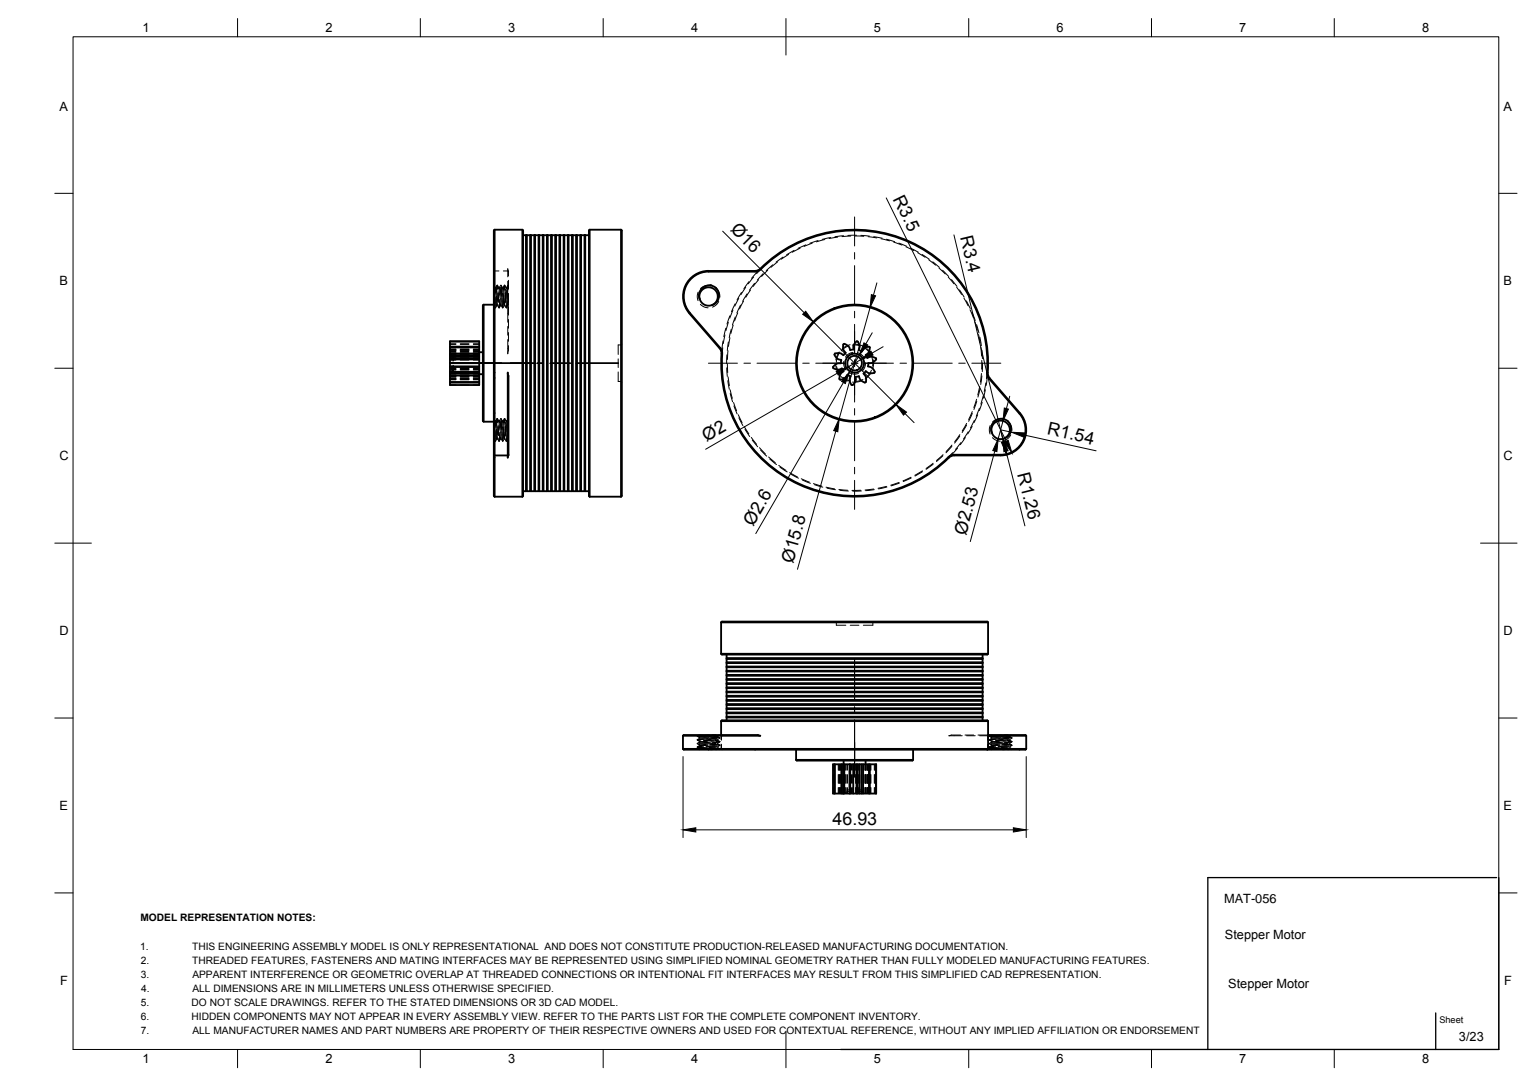
ISO-10303-21;
HEADER;
/* Generated by software containing ST-Developer
 * from STEP Tools, Inc. (www.steptools.com) 
 */

FILE_DESCRIPTION(
/* description */ (''),
/* implementation_level */ '2;1');

FILE_NAME(
/* name */ 'Stepper Motor.step',
/* time_stamp */ '2026-10-28T16:47:13+01:00',
/* author */ (''),
/* organization */ (''),
/* preprocessor_version */ 'ST-DEVELOPER v20.2',
/* originating_system */ 'Autodesk Translation Framework v15.17.0.0',
/* authorisation */ '');

FILE_SCHEMA (('AUTOMOTIVE_DESIGN { 1 0 10303 214 3 1 1 }'));
ENDSEC;

DATA;
#10=MECHANICAL_DESIGN_GEOMETRIC_PRESENTATION_REPRESENTATION('',(#4494,#4495,#4496,#4497,#4498,#4499,#4500,#4501,#4502,#4503,#4504,#4505,#4506,#4507,#4508,#4509,#4510,#4511,#4512,#4513,#4514,#4515,#4516,#4517,#4518,#4519,#4520,#4521,#4522,#4523,#4524,#4525,#4526,#4527,#4528,#4529,#4530,#4531,#4532,#4533,#4534,#4535,#4536,#4537,#4538,#4539,#4540,#4541,#4542,#4543,#4544,#4545,#4546,#4547,#4548,#4549,#4550,#4551,#4552,#4553,#4554,#4555,#4556,#4557,#4558,#4559,#4560,#4561,#4562,#4563,#4564,#4565,#4566),#459242);
#4405=SHAPE_REPRESENTATION_RELATIONSHIP('SRR','None',#459330,#4426);
#4426=ADVANCED_BREP_SHAPE_REPRESENTATION('',(#4447),#459219);
#4447=MANIFOLD_SOLID_BREP('NEMA14 body',#94623);
#4494=STYLED_ITEM('',(#459540),#88842);
#4495=STYLED_ITEM('',(#459540),#88843);
#4496=STYLED_ITEM('',(#459540),#88846);
#4497=STYLED_ITEM('',(#459540),#88849);
#4498=STYLED_ITEM('',(#459540),#88881);
#4499=STYLED_ITEM('',(#459540),#88885);
#4500=STYLED_ITEM('',(#459540),#88886);
#4501=STYLED_ITEM('',(#459540),#88887);
#4502=STYLED_ITEM('',(#459540),#88888);
#4503=STYLED_ITEM('',(#459540),#88889);
#4504=STYLED_ITEM('',(#459540),#88890);
#4505=STYLED_ITEM('',(#459540),#88891);
#4506=STYLED_ITEM('',(#459540),#88892);
#4507=STYLED_ITEM('',(#459540),#88893);
#4508=STYLED_ITEM('',(#459540),#88894);
#4509=STYLED_ITEM('',(#459540),#88895);
#4510=STYLED_ITEM('',(#459540),#88896);
#4511=STYLED_ITEM('',(#459540),#88897);
#4512=STYLED_ITEM('',(#459540),#88898);
#4513=STYLED_ITEM('',(#459540),#88899);
#4514=STYLED_ITEM('',(#459540),#88900);
#4515=STYLED_ITEM('',(#459540),#88901);
#4516=STYLED_ITEM('',(#459540),#88902);
#4517=STYLED_ITEM('',(#459540),#88903);
#4518=STYLED_ITEM('',(#459540),#88904);
#4519=STYLED_ITEM('',(#459540),#88905);
#4520=STYLED_ITEM('',(#459540),#88906);
#4521=STYLED_ITEM('',(#459540),#88907);
#4522=STYLED_ITEM('',(#459540),#88908);
#4523=STYLED_ITEM('',(#459540),#88909);
#4524=STYLED_ITEM('',(#459540),#88910);
#4525=STYLED_ITEM('',(#459540),#88911);
#4526=STYLED_ITEM('',(#459540),#88912);
#4527=STYLED_ITEM('',(#459540),#88913);
#4528=STYLED_ITEM('',(#459540),#88914);
#4529=STYLED_ITEM('',(#459540),#88915);
#4530=STYLED_ITEM('',(#459540),#88916);
#4531=STYLED_ITEM('',(#459540),#88917);
#4532=STYLED_ITEM('',(#459540),#88918);
#4533=STYLED_ITEM('',(#459540),#88919);
#4534=STYLED_ITEM('',(#459540),#88920);
#4535=STYLED_ITEM('',(#459540),#88921);
#4536=STYLED_ITEM('',(#459540),#88922);
#4537=STYLED_ITEM('',(#459540),#88923);
#4538=STYLED_ITEM('',(#459540),#88924);
#4539=STYLED_ITEM('',(#459540),#88925);
#4540=STYLED_ITEM('',(#459540),#88926);
#4541=STYLED_ITEM('',(#459540),#88927);
#4542=STYLED_ITEM('',(#459540),#88928);
#4543=STYLED_ITEM('',(#459540),#88929);
#4544=STYLED_ITEM('',(#459540),#88930);
#4545=STYLED_ITEM('',(#459540),#88931);
#4546=STYLED_ITEM('',(#459540),#88932);
#4547=STYLED_ITEM('',(#459540),#88933);
#4548=STYLED_ITEM('',(#459540),#88934);
#4549=STYLED_ITEM('',(#459540),#88935);
#4550=STYLED_ITEM('',(#459540),#88936);
#4551=STYLED_ITEM('',(#459540),#88937);
#4552=STYLED_ITEM('',(#459540),#88938);
#4553=STYLED_ITEM('',(#459540),#88939);
#4554=STYLED_ITEM('',(#459540),#88940);
#4555=STYLED_ITEM('',(#459540),#88941);
#4556=STYLED_ITEM('',(#459540),#88942);
#4557=STYLED_ITEM('',(#459540),#88943);
#4558=STYLED_ITEM('',(#459540),#88944);
#4559=STYLED_ITEM('',(#459540),#88945);
#4560=STYLED_ITEM('',(#459540),#88946);
#4561=STYLED_ITEM('',(#459540),#88947);
#4562=STYLED_ITEM('',(#459540),#88948);
#4563=STYLED_ITEM('',(#459540),#88949);
#4564=STYLED_ITEM('',(#459540),#88997);
#4565=STYLED_ITEM('',(#459540),#88999);
#4566=STYLED_ITEM('',(#459540),#4447);
#4614=CONICAL_SURFACE('',#94946,7.95,0.785398163397448);
#4615=CONICAL_SURFACE('',#94953,18.2,0.785398163397448);
#4616=CONICAL_SURFACE('',#94962,18.2,0.785398163397437);
#4617=CONICAL_SURFACE('',#94970,2.55,0.785398163397459);
#4618=CONICAL_SURFACE('',#94977,18.2,0.785398163397459);
#4619=CONICAL_SURFACE('',#94978,1.05,0.785398163397442);
#4620=CONICAL_SURFACE('',#94981,3.45000000056584,0.785398163397459);
#4621=CONICAL_SURFACE('',#94984,1.05,0.785398163397449);
#4622=CONICAL_SURFACE('',#94986,1.05,0.785398163397451);
#4623=CONICAL_SURFACE('',#94989,3.44999999943895,0.785398163397441);
#4624=CONICAL_SURFACE('',#94992,1.05,0.785398163397451);
#4625=CONICAL_SURFACE('',#94995,3.44999999943895,0.785398163397441);
#4626=CONICAL_SURFACE('',#94999,1.05,0.785398163397451);
#4627=CONICAL_SURFACE('',#95002,18.2,0.785398163397448);
#4628=CONICAL_SURFACE('',#95004,1.05,0.785398163397449);
#4629=CONICAL_SURFACE('',#95008,3.45000000056584,0.785398163397459);
#4630=CONICAL_SURFACE('',#95012,1.05,0.785398163397442);
#4631=CONICAL_SURFACE('',#95015,18.2,0.785398163397437);
#4632=CONICAL_SURFACE('',#95017,1.05,0.785398163397451);
#4633=CONICAL_SURFACE('',#95029,1.15,0.785398163397448);
#4634=CONICAL_SURFACE('',#95118,17.45,1.10714871779409);
#4635=CONICAL_SURFACE('',#95122,17.45,1.10714871779411);
#4636=CONICAL_SURFACE('',#95129,17.45,1.10714871779409);
#4637=CONICAL_SURFACE('',#95133,17.45,1.10714871779411);
#4638=CONICAL_SURFACE('',#95137,17.45,1.10714871779409);
#4639=CONICAL_SURFACE('',#95141,17.45,1.10714871779411);
#4640=CONICAL_SURFACE('',#95145,17.45,1.10714871779409);
#4641=CONICAL_SURFACE('',#95149,17.45,1.10714871779411);
#4642=CONICAL_SURFACE('',#95153,17.45,1.10714871779409);
#4643=CONICAL_SURFACE('',#95157,17.45,1.10714871779411);
#4644=CONICAL_SURFACE('',#95161,17.45,1.10714871779409);
#4645=CONICAL_SURFACE('',#95165,17.45,1.10714871779411);
#4646=CONICAL_SURFACE('',#95169,17.45,1.10714871779409);
#4647=CONICAL_SURFACE('',#95173,17.45,1.10714871779411);
#4648=CONICAL_SURFACE('',#95177,17.45,1.10714871779409);
#4649=CONICAL_SURFACE('',#95181,17.45,1.10714871779411);
#4650=CONICAL_SURFACE('',#95185,17.45,1.10714871779409);
#4651=CONICAL_SURFACE('',#95189,17.45,1.10714871779411);
#4652=CONICAL_SURFACE('',#95193,17.45,1.10714871779409);
#4653=CONICAL_SURFACE('',#95197,17.45,1.10714871779411);
#4654=CONICAL_SURFACE('',#95201,17.45,1.10714871779409);
#4655=CONICAL_SURFACE('',#95205,17.45,1.10714871779411);
#4656=CONICAL_SURFACE('',#95209,17.45,1.10714871779409);
#4657=CONICAL_SURFACE('',#95213,17.45,1.10714871779411);
#4658=CONICAL_SURFACE('',#95217,17.45,1.10714871779409);
#4659=CONICAL_SURFACE('',#95221,17.45,1.10714871779411);
#4660=CONICAL_SURFACE('',#95225,17.45,1.10714871779409);
#4661=CONICAL_SURFACE('',#95229,17.45,1.10714871779411);
#4662=CONICAL_SURFACE('',#95234,17.45,1.10714871779409);
#4663=CONICAL_SURFACE('',#95238,17.45,1.10714871779411);
#5113=FACE_BOUND('',#12182,.T.);
#5114=FACE_BOUND('',#12186,.T.);
#5115=FACE_BOUND('',#12190,.T.);
#5116=FACE_BOUND('',#12194,.T.);
#5117=FACE_BOUND('',#12198,.T.);
#5118=FACE_BOUND('',#12201,.T.);
#5119=FACE_BOUND('',#12232,.T.);
#5120=FACE_BOUND('',#12233,.T.);
#5121=FACE_BOUND('',#12234,.T.);
#5122=FACE_BOUND('',#12241,.T.);
#5123=FACE_BOUND('',#12244,.T.);
#5278=PLANE('',#94935);
#5279=PLANE('',#94940);
#5280=PLANE('',#94951);
#5281=PLANE('',#94960);
#5282=PLANE('',#94968);
#5283=PLANE('',#94973);
#5284=PLANE('',#94980);
#5285=PLANE('',#94983);
#5286=PLANE('',#94988);
#5287=PLANE('',#94991);
#5288=PLANE('',#94994);
#5289=PLANE('',#94998);
#5290=PLANE('',#95007);
#5291=PLANE('',#95011);
#5292=PLANE('',#95021);
#5293=PLANE('',#95024);
#5294=PLANE('',#95025);
#5295=PLANE('',#95028);
#5296=PLANE('',#95034);
#5297=PLANE('',#95055);
#5298=PLANE('',#95056);
#5299=PLANE('',#95078);
#5300=PLANE('',#95080);
#5301=PLANE('',#95083);
#5302=PLANE('',#95085);
#5303=PLANE('',#95087);
#5304=PLANE('',#95089);
#5305=PLANE('',#95091);
#5306=PLANE('',#95093);
#5307=PLANE('',#95095);
#5308=PLANE('',#95097);
#5309=PLANE('',#95099);
#5310=PLANE('',#95101);
#5311=PLANE('',#95103);
#5312=PLANE('',#95105);
#5313=PLANE('',#95107);
#5314=PLANE('',#95109);
#5315=PLANE('',#95111);
#5316=PLANE('',#95113);
#5317=PLANE('',#95115);
#5318=PLANE('',#95117);
#5319=PLANE('',#95241);
#5320=PLANE('',#95242);
#6181=B_SPLINE_SURFACE_WITH_KNOTS('',3,3,((#136116,#136117,#136118,#136119,
#136120,#136121,#136122,#136123,#136124,#136125,#136126,#136127,#136128,
#136129,#136130,#136131,#136132,#136133,#136134,#136135,#136136,#136137,
#136138,#136139,#136140,#136141,#136142,#136143,#136144,#136145,#136146),
(#136147,#136148,#136149,#136150,#136151,#136152,#136153,#136154,#136155,
#136156,#136157,#136158,#136159,#136160,#136161,#136162,#136163,#136164,
#136165,#136166,#136167,#136168,#136169,#136170,#136171,#136172,#136173,
#136174,#136175,#136176,#136177),(#136178,#136179,#136180,#136181,#136182,
#136183,#136184,#136185,#136186,#136187,#136188,#136189,#136190,#136191,
#136192,#136193,#136194,#136195,#136196,#136197,#136198,#136199,#136200,
#136201,#136202,#136203,#136204,#136205,#136206,#136207,#136208),(#136209,
#136210,#136211,#136212,#136213,#136214,#136215,#136216,#136217,#136218,
#136219,#136220,#136221,#136222,#136223,#136224,#136225,#136226,#136227,
#136228,#136229,#136230,#136231,#136232,#136233,#136234,#136235,#136236,
#136237,#136238,#136239)),.UNSPECIFIED.,.F.,.F.,.F.,(4,4),(4,1,1,1,1,1,
1,1,1,1,1,1,1,1,1,1,1,1,1,1,1,1,1,1,1,1,1,1,4),(-0.000238175110720029,0.0327432610208062),
(11.8551230884687,12.8251224678821,13.7948836721847,14.7646448764874,15.7344060807901,
16.7041672850928,17.6739284893955,18.6436896936982,19.6134508980009,20.5832121023036,
21.5529733066062,22.5227345109089,23.4924957152116,24.4622569195143,25.432018123817,
26.4017793281197,27.3715405324224,28.3413017367251,29.3110629410278,30.2808241453304,
31.2505853496331,32.2203465539358,33.1901077582385,34.1598689625412,35.1296301668439,
36.0993913711466,37.0691525754493,38.038913779752,39.0090475285257),
 .UNSPECIFIED.);
#6182=B_SPLINE_SURFACE_WITH_KNOTS('',3,3,((#136336,#136337,#136338,#136339,
#136340,#136341,#136342,#136343,#136344,#136345,#136346,#136347,#136348,
#136349,#136350,#136351,#136352,#136353,#136354,#136355,#136356,#136357,
#136358,#136359,#136360,#136361,#136362,#136363,#136364,#136365,#136366),
(#136367,#136368,#136369,#136370,#136371,#136372,#136373,#136374,#136375,
#136376,#136377,#136378,#136379,#136380,#136381,#136382,#136383,#136384,
#136385,#136386,#136387,#136388,#136389,#136390,#136391,#136392,#136393,
#136394,#136395,#136396,#136397),(#136398,#136399,#136400,#136401,#136402,
#136403,#136404,#136405,#136406,#136407,#136408,#136409,#136410,#136411,
#136412,#136413,#136414,#136415,#136416,#136417,#136418,#136419,#136420,
#136421,#136422,#136423,#136424,#136425,#136426,#136427,#136428),(#136429,
#136430,#136431,#136432,#136433,#136434,#136435,#136436,#136437,#136438,
#136439,#136440,#136441,#136442,#136443,#136444,#136445,#136446,#136447,
#136448,#136449,#136450,#136451,#136452,#136453,#136454,#136455,#136456,
#136457,#136458,#136459)),.UNSPECIFIED.,.F.,.F.,.F.,(4,4),(4,1,1,1,1,1,
1,1,1,1,1,1,1,1,1,1,1,1,1,1,1,1,1,1,1,1,1,1,4),(-0.000593092618099697,0.0323402178569243),
(14.3981249632437,15.3681613312746,16.3379225355772,17.3076837398799,18.2774449441826,
19.2472061484853,20.216967352788,21.1867285570907,22.1564897613934,23.1262509656961,
24.0960121699988,25.0657733743014,26.0355345786041,27.0052957829068,27.9750569872095,
28.9448181915122,29.9145793958149,30.8843406001176,31.8541018044203,32.8238630087229,
33.7936242130256,34.7633854173283,35.733146621631,36.7029078259337,37.6726690302364,
38.6424302345391,39.6121914388418,40.5819526431444,41.5517138474471),
 .UNSPECIFIED.);
#6183=B_SPLINE_SURFACE_WITH_KNOTS('',3,3,((#136639,#136640,#136641,#136642,
#136643,#136644,#136645,#136646,#136647,#136648,#136649,#136650,#136651,
#136652,#136653,#136654,#136655,#136656,#136657,#136658,#136659,#136660,
#136661,#136662,#136663,#136664,#136665,#136666,#136667,#136668,#136669),
(#136670,#136671,#136672,#136673,#136674,#136675,#136676,#136677,#136678,
#136679,#136680,#136681,#136682,#136683,#136684,#136685,#136686,#136687,
#136688,#136689,#136690,#136691,#136692,#136693,#136694,#136695,#136696,
#136697,#136698,#136699,#136700),(#136701,#136702,#136703,#136704,#136705,
#136706,#136707,#136708,#136709,#136710,#136711,#136712,#136713,#136714,
#136715,#136716,#136717,#136718,#136719,#136720,#136721,#136722,#136723,
#136724,#136725,#136726,#136727,#136728,#136729,#136730,#136731),(#136732,
#136733,#136734,#136735,#136736,#136737,#136738,#136739,#136740,#136741,
#136742,#136743,#136744,#136745,#136746,#136747,#136748,#136749,#136750,
#136751,#136752,#136753,#136754,#136755,#136756,#136757,#136758,#136759,
#136760,#136761,#136762)),.UNSPECIFIED.,.F.,.F.,.F.,(4,4),(4,1,1,1,1,1,
1,1,1,1,1,1,1,1,1,1,1,1,1,1,1,1,1,1,1,1,1,1,4),(-0.000238191648974563,0.0327432700752779),
(11.8551230719304,12.825122467882,13.7948836721847,14.7646448764874,15.7344060807901,
16.7041672850928,17.6739284893955,18.6436896936982,19.6134508980009,20.5832121023035,
21.5529733066062,22.5227345109089,23.4924957152116,24.4622569195143,25.432018123817,
26.4017793281197,27.3715405324224,28.3413017367251,29.3110629410277,30.2808241453304,
31.2505853496331,32.2203465539358,33.1901077582385,34.1598689625412,35.1296301668439,
36.0993913711466,37.0691525754492,38.0389137797519,39.0090475313925),
 .UNSPECIFIED.);
#6184=B_SPLINE_SURFACE_WITH_KNOTS('',3,3,((#136859,#136860,#136861,#136862,
#136863,#136864,#136865,#136866,#136867,#136868,#136869,#136870,#136871,
#136872,#136873,#136874,#136875,#136876,#136877,#136878,#136879,#136880,
#136881,#136882,#136883,#136884,#136885,#136886,#136887,#136888,#136889),
(#136890,#136891,#136892,#136893,#136894,#136895,#136896,#136897,#136898,
#136899,#136900,#136901,#136902,#136903,#136904,#136905,#136906,#136907,
#136908,#136909,#136910,#136911,#136912,#136913,#136914,#136915,#136916,
#136917,#136918,#136919,#136920),(#136921,#136922,#136923,#136924,#136925,
#136926,#136927,#136928,#136929,#136930,#136931,#136932,#136933,#136934,
#136935,#136936,#136937,#136938,#136939,#136940,#136941,#136942,#136943,
#136944,#136945,#136946,#136947,#136948,#136949,#136950,#136951),(#136952,
#136953,#136954,#136955,#136956,#136957,#136958,#136959,#136960,#136961,
#136962,#136963,#136964,#136965,#136966,#136967,#136968,#136969,#136970,
#136971,#136972,#136973,#136974,#136975,#136976,#136977,#136978,#136979,
#136980,#136981,#136982)),.UNSPECIFIED.,.F.,.F.,.F.,(4,4),(4,1,1,1,1,1,
1,1,1,1,1,1,1,1,1,1,1,1,1,1,1,1,1,1,1,1,1,1,4),(-0.000593069084645025,0.0323402181589899),
(14.3981249570381,15.3681613312745,16.3379225355772,17.3076837398799,18.2774449441826,
19.2472061484853,20.216967352788,21.1867285570907,22.1564897613934,23.1262509656961,
24.0960121699987,25.0657733743014,26.0355345786041,27.0052957829068,27.9750569872095,
28.9448181915122,29.9145793958149,30.8843406001176,31.8541018044202,32.8238630087229,
33.7936242130256,34.7633854173283,35.733146621631,36.7029078259337,37.6726690302364,
38.6424302345391,39.6121914388417,40.5819526431444,41.5517138474471),
 .UNSPECIFIED.);
#6185=B_SPLINE_SURFACE_WITH_KNOTS('',3,1,((#137824,#137825),(#137826,#137827),
(#137828,#137829),(#137830,#137831),(#137832,#137833),(#137834,#137835)),
 .UNSPECIFIED.,.F.,.F.,.F.,(4,1,1,4),(2,2),(0.,0.285714285714286,0.571428571428571,
1.),(0.,0.576),.UNSPECIFIED.);
#6186=B_SPLINE_SURFACE_WITH_KNOTS('',3,1,((#137839,#137840),(#137841,#137842),
(#137843,#137844),(#137845,#137846),(#137847,#137848),(#137849,#137850)),
 .UNSPECIFIED.,.F.,.F.,.F.,(4,2,4),(2,2),(0.,0.483208689475554,1.),(0.,
0.576000000000006),.UNSPECIFIED.);
#6187=B_SPLINE_SURFACE_WITH_KNOTS('',3,1,((#137861,#137862),(#137863,#137864),
(#137865,#137866),(#137867,#137868),(#137869,#137870),(#137871,#137872)),
 .UNSPECIFIED.,.F.,.F.,.F.,(4,1,1,4),(2,2),(0.,0.285714285714286,0.571428571428571,
1.),(0.,0.576),.UNSPECIFIED.);
#6188=B_SPLINE_SURFACE_WITH_KNOTS('',3,1,((#137876,#137877),(#137878,#137879),
(#137880,#137881),(#137882,#137883),(#137884,#137885),(#137886,#137887)),
 .UNSPECIFIED.,.F.,.F.,.F.,(4,2,4),(2,2),(0.,0.483208689475554,1.),(0.,
0.576000000000006),.UNSPECIFIED.);
#6189=B_SPLINE_SURFACE_WITH_KNOTS('',3,1,((#137895,#137896),(#137897,#137898),
(#137899,#137900),(#137901,#137902),(#137903,#137904),(#137905,#137906)),
 .UNSPECIFIED.,.F.,.F.,.F.,(4,1,1,4),(2,2),(0.,0.285714285714286,0.571428571428571,
1.),(0.,0.576),.UNSPECIFIED.);
#6190=B_SPLINE_SURFACE_WITH_KNOTS('',3,1,((#137910,#137911),(#137912,#137913),
(#137914,#137915),(#137916,#137917),(#137918,#137919),(#137920,#137921)),
 .UNSPECIFIED.,.F.,.F.,.F.,(4,2,4),(2,2),(0.,0.483208689475554,1.),(0.,
0.576000000000006),.UNSPECIFIED.);
#6191=B_SPLINE_SURFACE_WITH_KNOTS('',3,1,((#137929,#137930),(#137931,#137932),
(#137933,#137934),(#137935,#137936),(#137937,#137938),(#137939,#137940)),
 .UNSPECIFIED.,.F.,.F.,.F.,(4,1,1,4),(2,2),(0.,0.285714285714286,0.571428571428571,
1.),(0.,0.576),.UNSPECIFIED.);
#6192=B_SPLINE_SURFACE_WITH_KNOTS('',3,1,((#137944,#137945),(#137946,#137947),
(#137948,#137949),(#137950,#137951),(#137952,#137953),(#137954,#137955)),
 .UNSPECIFIED.,.F.,.F.,.F.,(4,2,4),(2,2),(0.,0.483208689475554,1.),(0.,
0.576000000000006),.UNSPECIFIED.);
#6193=B_SPLINE_SURFACE_WITH_KNOTS('',3,1,((#137963,#137964),(#137965,#137966),
(#137967,#137968),(#137969,#137970),(#137971,#137972),(#137973,#137974)),
 .UNSPECIFIED.,.F.,.F.,.F.,(4,1,1,4),(2,2),(0.,0.285714285714286,0.571428571428571,
1.),(0.,0.576),.UNSPECIFIED.);
#6194=B_SPLINE_SURFACE_WITH_KNOTS('',3,1,((#137978,#137979),(#137980,#137981),
(#137982,#137983),(#137984,#137985),(#137986,#137987),(#137988,#137989)),
 .UNSPECIFIED.,.F.,.F.,.F.,(4,2,4),(2,2),(0.,0.483208689475554,1.),(0.,
0.576000000000006),.UNSPECIFIED.);
#6195=B_SPLINE_SURFACE_WITH_KNOTS('',3,1,((#137997,#137998),(#137999,#138000),
(#138001,#138002),(#138003,#138004),(#138005,#138006),(#138007,#138008)),
 .UNSPECIFIED.,.F.,.F.,.F.,(4,1,1,4),(2,2),(0.,0.285714285714286,0.571428571428571,
1.),(0.,0.576),.UNSPECIFIED.);
#6196=B_SPLINE_SURFACE_WITH_KNOTS('',3,1,((#138012,#138013),(#138014,#138015),
(#138016,#138017),(#138018,#138019),(#138020,#138021),(#138022,#138023)),
 .UNSPECIFIED.,.F.,.F.,.F.,(4,2,4),(2,2),(0.,0.483208689475554,1.),(0.,
0.576000000000006),.UNSPECIFIED.);
#6197=B_SPLINE_SURFACE_WITH_KNOTS('',3,1,((#138031,#138032),(#138033,#138034),
(#138035,#138036),(#138037,#138038),(#138039,#138040),(#138041,#138042)),
 .UNSPECIFIED.,.F.,.F.,.F.,(4,1,1,4),(2,2),(0.,0.285714285714286,0.571428571428571,
1.),(0.,0.576),.UNSPECIFIED.);
#6198=B_SPLINE_SURFACE_WITH_KNOTS('',3,1,((#138046,#138047),(#138048,#138049),
(#138050,#138051),(#138052,#138053),(#138054,#138055),(#138056,#138057)),
 .UNSPECIFIED.,.F.,.F.,.F.,(4,2,4),(2,2),(0.,0.483208689475554,1.),(0.,
0.576000000000006),.UNSPECIFIED.);
#6199=B_SPLINE_SURFACE_WITH_KNOTS('',3,1,((#138065,#138066),(#138067,#138068),
(#138069,#138070),(#138071,#138072),(#138073,#138074),(#138075,#138076)),
 .UNSPECIFIED.,.F.,.F.,.F.,(4,1,1,4),(2,2),(0.,0.285714285714286,0.571428571428571,
1.),(0.,0.576),.UNSPECIFIED.);
#6200=B_SPLINE_SURFACE_WITH_KNOTS('',3,1,((#138080,#138081),(#138082,#138083),
(#138084,#138085),(#138086,#138087),(#138088,#138089),(#138090,#138091)),
 .UNSPECIFIED.,.F.,.F.,.F.,(4,2,4),(2,2),(0.,0.483208689475554,1.),(0.,
0.576000000000006),.UNSPECIFIED.);
#6201=B_SPLINE_SURFACE_WITH_KNOTS('',3,1,((#138099,#138100),(#138101,#138102),
(#138103,#138104),(#138105,#138106),(#138107,#138108),(#138109,#138110)),
 .UNSPECIFIED.,.F.,.F.,.F.,(4,1,1,4),(2,2),(0.,0.285714285714286,0.571428571428571,
1.),(0.,0.576),.UNSPECIFIED.);
#6202=B_SPLINE_SURFACE_WITH_KNOTS('',3,1,((#138114,#138115),(#138116,#138117),
(#138118,#138119),(#138120,#138121),(#138122,#138123),(#138124,#138125)),
 .UNSPECIFIED.,.F.,.F.,.F.,(4,2,4),(2,2),(0.,0.483208689475554,1.),(0.,
0.576000000000006),.UNSPECIFIED.);
#6203=B_SPLINE_SURFACE_WITH_KNOTS('',3,1,((#138132,#138133),(#138134,#138135),
(#138136,#138137),(#138138,#138139),(#138140,#138141),(#138142,#138143)),
 .UNSPECIFIED.,.F.,.F.,.F.,(4,1,1,4),(2,2),(0.,0.285714285714286,0.571428571428571,
1.),(0.,0.576),.UNSPECIFIED.);
#6204=B_SPLINE_SURFACE_WITH_KNOTS('',3,1,((#138147,#138148),(#138149,#138150),
(#138151,#138152),(#138153,#138154),(#138155,#138156),(#138157,#138158)),
 .UNSPECIFIED.,.F.,.F.,.F.,(4,2,4),(2,2),(0.,0.483208689475554,1.),(0.,
0.576000000000006),.UNSPECIFIED.);
#6351=FACE_OUTER_BOUND('',#12159,.T.);
#6352=FACE_OUTER_BOUND('',#12160,.T.);
#6353=FACE_OUTER_BOUND('',#12161,.T.);
#6354=FACE_OUTER_BOUND('',#12162,.T.);
#6355=FACE_OUTER_BOUND('',#12163,.T.);
#6356=FACE_OUTER_BOUND('',#12164,.T.);
#6357=FACE_OUTER_BOUND('',#12165,.T.);
#6358=FACE_OUTER_BOUND('',#12166,.T.);
#6359=FACE_OUTER_BOUND('',#12167,.T.);
#6360=FACE_OUTER_BOUND('',#12168,.T.);
#6361=FACE_OUTER_BOUND('',#12169,.T.);
#6362=FACE_OUTER_BOUND('',#12170,.T.);
#6363=FACE_OUTER_BOUND('',#12171,.T.);
#6364=FACE_OUTER_BOUND('',#12172,.T.);
#6365=FACE_OUTER_BOUND('',#12173,.T.);
#6366=FACE_OUTER_BOUND('',#12174,.T.);
#6367=FACE_OUTER_BOUND('',#12175,.T.);
#6368=FACE_OUTER_BOUND('',#12176,.T.);
#6369=FACE_OUTER_BOUND('',#12177,.T.);
#6370=FACE_OUTER_BOUND('',#12178,.T.);
#6371=FACE_OUTER_BOUND('',#12179,.T.);
#6372=FACE_OUTER_BOUND('',#12180,.T.);
#6373=FACE_OUTER_BOUND('',#12181,.T.);
#6374=FACE_OUTER_BOUND('',#12183,.T.);
#6375=FACE_OUTER_BOUND('',#12184,.T.);
#6376=FACE_OUTER_BOUND('',#12185,.T.);
#6377=FACE_OUTER_BOUND('',#12187,.T.);
#6378=FACE_OUTER_BOUND('',#12188,.T.);
#6379=FACE_OUTER_BOUND('',#12189,.T.);
#6380=FACE_OUTER_BOUND('',#12191,.T.);
#6381=FACE_OUTER_BOUND('',#12192,.T.);
#6382=FACE_OUTER_BOUND('',#12193,.T.);
#6383=FACE_OUTER_BOUND('',#12195,.T.);
#6384=FACE_OUTER_BOUND('',#12196,.T.);
#6385=FACE_OUTER_BOUND('',#12197,.T.);
#6386=FACE_OUTER_BOUND('',#12199,.T.);
#6387=FACE_OUTER_BOUND('',#12200,.T.);
#6388=FACE_OUTER_BOUND('',#12202,.T.);
#6389=FACE_OUTER_BOUND('',#12203,.T.);
#6390=FACE_OUTER_BOUND('',#12204,.T.);
#6391=FACE_OUTER_BOUND('',#12205,.T.);
#6392=FACE_OUTER_BOUND('',#12206,.T.);
#6393=FACE_OUTER_BOUND('',#12207,.T.);
#6394=FACE_OUTER_BOUND('',#12208,.T.);
#6395=FACE_OUTER_BOUND('',#12209,.T.);
#6396=FACE_OUTER_BOUND('',#12210,.T.);
#6397=FACE_OUTER_BOUND('',#12211,.T.);
#6398=FACE_OUTER_BOUND('',#12212,.T.);
#6399=FACE_OUTER_BOUND('',#12213,.T.);
#6400=FACE_OUTER_BOUND('',#12214,.T.);
#6401=FACE_OUTER_BOUND('',#12215,.T.);
#6402=FACE_OUTER_BOUND('',#12216,.T.);
#6403=FACE_OUTER_BOUND('',#12217,.T.);
#6404=FACE_OUTER_BOUND('',#12218,.T.);
#6405=FACE_OUTER_BOUND('',#12219,.T.);
#6406=FACE_OUTER_BOUND('',#12220,.T.);
#6407=FACE_OUTER_BOUND('',#12221,.T.);
#6408=FACE_OUTER_BOUND('',#12222,.T.);
#6409=FACE_OUTER_BOUND('',#12223,.T.);
#6410=FACE_OUTER_BOUND('',#12224,.T.);
#6411=FACE_OUTER_BOUND('',#12225,.T.);
#6412=FACE_OUTER_BOUND('',#12226,.T.);
#6413=FACE_OUTER_BOUND('',#12227,.T.);
#6414=FACE_OUTER_BOUND('',#12228,.T.);
#6415=FACE_OUTER_BOUND('',#12229,.T.);
#6416=FACE_OUTER_BOUND('',#12230,.T.);
#6417=FACE_OUTER_BOUND('',#12231,.T.);
#6418=FACE_OUTER_BOUND('',#12235,.T.);
#6419=FACE_OUTER_BOUND('',#12236,.T.);
#6420=FACE_OUTER_BOUND('',#12237,.T.);
#6421=FACE_OUTER_BOUND('',#12238,.T.);
#6422=FACE_OUTER_BOUND('',#12239,.T.);
#6423=FACE_OUTER_BOUND('',#12240,.T.);
#6424=FACE_OUTER_BOUND('',#12242,.T.);
#6425=FACE_OUTER_BOUND('',#12243,.T.);
#6426=FACE_OUTER_BOUND('',#12245,.T.);
#6427=FACE_OUTER_BOUND('',#12246,.T.);
#6428=FACE_OUTER_BOUND('',#12247,.T.);
#6429=FACE_OUTER_BOUND('',#12248,.T.);
#6430=FACE_OUTER_BOUND('',#12249,.T.);
#6431=FACE_OUTER_BOUND('',#12250,.T.);
#6432=FACE_OUTER_BOUND('',#12251,.T.);
#6433=FACE_OUTER_BOUND('',#12252,.T.);
#6434=FACE_OUTER_BOUND('',#12253,.T.);
#6435=FACE_OUTER_BOUND('',#12254,.T.);
#6436=FACE_OUTER_BOUND('',#12255,.T.);
#6437=FACE_OUTER_BOUND('',#12256,.T.);
#6438=FACE_OUTER_BOUND('',#12257,.T.);
#6439=FACE_OUTER_BOUND('',#12258,.T.);
#6440=FACE_OUTER_BOUND('',#12259,.T.);
#6441=FACE_OUTER_BOUND('',#12260,.T.);
#6442=FACE_OUTER_BOUND('',#12261,.T.);
#6443=FACE_OUTER_BOUND('',#12262,.T.);
#6444=FACE_OUTER_BOUND('',#12263,.T.);
#6445=FACE_OUTER_BOUND('',#12264,.T.);
#6446=FACE_OUTER_BOUND('',#12265,.T.);
#6447=FACE_OUTER_BOUND('',#12266,.T.);
#6448=FACE_OUTER_BOUND('',#12267,.T.);
#6449=FACE_OUTER_BOUND('',#12268,.T.);
#6450=FACE_OUTER_BOUND('',#12269,.T.);
#6451=FACE_OUTER_BOUND('',#12270,.T.);
#6452=FACE_OUTER_BOUND('',#12271,.T.);
#6453=FACE_OUTER_BOUND('',#12272,.T.);
#6454=FACE_OUTER_BOUND('',#12273,.T.);
#6455=FACE_OUTER_BOUND('',#12274,.T.);
#6456=FACE_OUTER_BOUND('',#12275,.T.);
#6457=FACE_OUTER_BOUND('',#12276,.T.);
#6458=FACE_OUTER_BOUND('',#12277,.T.);
#6459=FACE_OUTER_BOUND('',#12278,.T.);
#6460=FACE_OUTER_BOUND('',#12279,.T.);
#6461=FACE_OUTER_BOUND('',#12280,.T.);
#6462=FACE_OUTER_BOUND('',#12281,.T.);
#6463=FACE_OUTER_BOUND('',#12282,.T.);
#6464=FACE_OUTER_BOUND('',#12283,.T.);
#6465=FACE_OUTER_BOUND('',#12284,.T.);
#6466=FACE_OUTER_BOUND('',#12285,.T.);
#6467=FACE_OUTER_BOUND('',#12286,.T.);
#6468=FACE_OUTER_BOUND('',#12287,.T.);
#6469=FACE_OUTER_BOUND('',#12288,.T.);
#6470=FACE_OUTER_BOUND('',#12289,.T.);
#6471=FACE_OUTER_BOUND('',#12290,.T.);
#6472=FACE_OUTER_BOUND('',#12291,.T.);
#6473=FACE_OUTER_BOUND('',#12292,.T.);
#6474=FACE_OUTER_BOUND('',#12293,.T.);
#6475=FACE_OUTER_BOUND('',#12294,.T.);
#6476=FACE_OUTER_BOUND('',#12295,.T.);
#6477=FACE_OUTER_BOUND('',#12296,.T.);
#6478=FACE_OUTER_BOUND('',#12297,.T.);
#6479=FACE_OUTER_BOUND('',#12298,.T.);
#6480=FACE_OUTER_BOUND('',#12299,.T.);
#6481=FACE_OUTER_BOUND('',#12300,.T.);
#6482=FACE_OUTER_BOUND('',#12301,.T.);
#6483=FACE_OUTER_BOUND('',#12302,.T.);
#6484=FACE_OUTER_BOUND('',#12303,.T.);
#6485=FACE_OUTER_BOUND('',#12304,.T.);
#6486=FACE_OUTER_BOUND('',#12305,.T.);
#6487=FACE_OUTER_BOUND('',#12306,.T.);
#6488=FACE_OUTER_BOUND('',#12307,.T.);
#6489=FACE_OUTER_BOUND('',#12308,.T.);
#6490=FACE_OUTER_BOUND('',#12309,.T.);
#6491=FACE_OUTER_BOUND('',#12310,.T.);
#6492=FACE_OUTER_BOUND('',#12311,.T.);
#6493=FACE_OUTER_BOUND('',#12312,.T.);
#6494=FACE_OUTER_BOUND('',#12313,.T.);
#6495=FACE_OUTER_BOUND('',#12314,.T.);
#6496=FACE_OUTER_BOUND('',#12315,.T.);
#6497=FACE_OUTER_BOUND('',#12316,.T.);
#6498=FACE_OUTER_BOUND('',#12317,.T.);
#6499=FACE_OUTER_BOUND('',#12318,.T.);
#6500=FACE_OUTER_BOUND('',#12319,.T.);
#6501=FACE_OUTER_BOUND('',#12320,.T.);
#6502=FACE_OUTER_BOUND('',#12321,.T.);
#6503=FACE_OUTER_BOUND('',#12322,.T.);
#6504=FACE_OUTER_BOUND('',#12323,.T.);
#6505=FACE_OUTER_BOUND('',#12324,.T.);
#6506=FACE_OUTER_BOUND('',#12325,.T.);
#6507=FACE_OUTER_BOUND('',#12326,.T.);
#6508=FACE_OUTER_BOUND('',#12327,.T.);
#6509=FACE_OUTER_BOUND('',#12328,.T.);
#6510=FACE_OUTER_BOUND('',#12329,.T.);
#6511=FACE_OUTER_BOUND('',#12330,.T.);
#6512=FACE_OUTER_BOUND('',#12331,.T.);
#6513=FACE_OUTER_BOUND('',#12332,.T.);
#6514=FACE_OUTER_BOUND('',#12333,.T.);
#6515=FACE_OUTER_BOUND('',#12334,.T.);
#6516=FACE_OUTER_BOUND('',#12335,.T.);
#6517=FACE_OUTER_BOUND('',#12336,.T.);
#6518=FACE_OUTER_BOUND('',#12337,.T.);
#6519=FACE_OUTER_BOUND('',#12338,.T.);
#6520=FACE_OUTER_BOUND('',#12339,.T.);
#6521=FACE_OUTER_BOUND('',#12340,.T.);
#6522=FACE_OUTER_BOUND('',#12341,.T.);
#6523=FACE_OUTER_BOUND('',#12342,.T.);
#6524=FACE_OUTER_BOUND('',#12343,.T.);
#6525=FACE_OUTER_BOUND('',#12344,.T.);
#6526=FACE_OUTER_BOUND('',#12345,.T.);
#6527=FACE_OUTER_BOUND('',#12346,.T.);
#6528=FACE_OUTER_BOUND('',#12347,.T.);
#6529=FACE_OUTER_BOUND('',#12348,.T.);
#6530=FACE_OUTER_BOUND('',#12349,.T.);
#6531=FACE_OUTER_BOUND('',#12350,.T.);
#6532=FACE_OUTER_BOUND('',#12351,.T.);
#6533=FACE_OUTER_BOUND('',#12352,.T.);
#6534=FACE_OUTER_BOUND('',#12353,.T.);
#6535=FACE_OUTER_BOUND('',#12354,.T.);
#12159=EDGE_LOOP('',(#58028,#58029,#58030,#58031,#58032));
#12160=EDGE_LOOP('',(#58033,#58034,#58035,#58036,#58037));
#12161=EDGE_LOOP('',(#58038,#58039,#58040,#58041,#58042));
#12162=EDGE_LOOP('',(#58043,#58044,#58045,#58046));
#12163=EDGE_LOOP('',(#58047,#58048,#58049,#58050,#58051));
#12164=EDGE_LOOP('',(#58052,#58053,#58054,#58055,#58056));
#12165=EDGE_LOOP('',(#58057,#58058,#58059,#58060,#58061));
#12166=EDGE_LOOP('',(#58062,#58063,#58064,#58065));
#12167=EDGE_LOOP('',(#58066,#58067,#58068,#58069));
#12168=EDGE_LOOP('',(#58070,#58071,#58072,#58073,#58074,#58075));
#12169=EDGE_LOOP('',(#58076,#58077,#58078,#58079,#58080,#58081));
#12170=EDGE_LOOP('',(#58082,#58083,#58084,#58085,#58086));
#12171=EDGE_LOOP('',(#58087,#58088,#58089,#58090));
#12172=EDGE_LOOP('',(#58091,#58092,#58093,#58094,#58095,#58096));
#12173=EDGE_LOOP('',(#58097,#58098,#58099,#58100,#58101,#58102));
#12174=EDGE_LOOP('',(#58103,#58104,#58105,#58106,#58107));
#12175=EDGE_LOOP('',(#58108,#58109,#58110,#58111));
#12176=EDGE_LOOP('',(#58112,#58113,#58114,#58115));
#12177=EDGE_LOOP('',(#58116,#58117,#58118,#58119,#58120));
#12178=EDGE_LOOP('',(#58121,#58122,#58123,#58124,#58125));
#12179=EDGE_LOOP('',(#58126,#58127,#58128,#58129,#58130,#58131,#58132,#58133,
#58134,#58135,#58136,#58137,#58138,#58139));
#12180=EDGE_LOOP('',(#58140,#58141,#58142,#58143,#58144,#58145,#58146,#58147,
#58148,#58149,#58150,#58151,#58152,#58153,#58154,#58155,#58156,#58157,#58158,
#58159));
#12181=EDGE_LOOP('',(#58160,#58161,#58162,#58163,#58164,#58165));
#12182=EDGE_LOOP('',(#58166,#58167,#58168,#58169));
#12183=EDGE_LOOP('',(#58170,#58171,#58172,#58173,#58174,#58175,#58176,#58177,
#58178,#58179,#58180,#58181,#58182,#58183));
#12184=EDGE_LOOP('',(#58184,#58185,#58186,#58187,#58188,#58189,#58190,#58191,
#58192,#58193,#58194,#58195,#58196,#58197,#58198,#58199,#58200,#58201,#58202,
#58203));
#12185=EDGE_LOOP('',(#58204,#58205,#58206,#58207,#58208,#58209,#58210));
#12186=EDGE_LOOP('',(#58211,#58212,#58213,#58214));
#12187=EDGE_LOOP('',(#58215,#58216,#58217,#58218));
#12188=EDGE_LOOP('',(#58219,#58220,#58221,#58222));
#12189=EDGE_LOOP('',(#58223));
#12190=EDGE_LOOP('',(#58224));
#12191=EDGE_LOOP('',(#58225,#58226,#58227,#58228,#58229));
#12192=EDGE_LOOP('',(#58230,#58231,#58232,#58233,#58234,#58235,#58236,#58237,
#58238,#58239,#58240,#58241,#58242,#58243,#58244,#58245,#58246));
#12193=EDGE_LOOP('',(#58247));
#12194=EDGE_LOOP('',(#58248));
#12195=EDGE_LOOP('',(#58249,#58250,#58251,#58252,#58253));
#12196=EDGE_LOOP('',(#58254,#58255,#58256,#58257,#58258));
#12197=EDGE_LOOP('',(#58259));
#12198=EDGE_LOOP('',(#58260));
#12199=EDGE_LOOP('',(#58261,#58262,#58263,#58264));
#12200=EDGE_LOOP('',(#58265));
#12201=EDGE_LOOP('',(#58266));
#12202=EDGE_LOOP('',(#58267,#58268,#58269,#58270));
#12203=EDGE_LOOP('',(#58271,#58272,#58273,#58274));
#12204=EDGE_LOOP('',(#58275,#58276,#58277,#58278));
#12205=EDGE_LOOP('',(#58279,#58280,#58281,#58282));
#12206=EDGE_LOOP('',(#58283,#58284,#58285,#58286));
#12207=EDGE_LOOP('',(#58287,#58288,#58289,#58290));
#12208=EDGE_LOOP('',(#58291,#58292,#58293,#58294));
#12209=EDGE_LOOP('',(#58295,#58296,#58297,#58298));
#12210=EDGE_LOOP('',(#58299,#58300,#58301,#58302));
#12211=EDGE_LOOP('',(#58303,#58304,#58305,#58306));
#12212=EDGE_LOOP('',(#58307,#58308,#58309,#58310));
#12213=EDGE_LOOP('',(#58311,#58312,#58313,#58314));
#12214=EDGE_LOOP('',(#58315,#58316,#58317,#58318));
#12215=EDGE_LOOP('',(#58319,#58320,#58321,#58322));
#12216=EDGE_LOOP('',(#58323,#58324,#58325,#58326));
#12217=EDGE_LOOP('',(#58327,#58328,#58329,#58330));
#12218=EDGE_LOOP('',(#58331,#58332,#58333,#58334));
#12219=EDGE_LOOP('',(#58335,#58336,#58337,#58338));
#12220=EDGE_LOOP('',(#58339,#58340,#58341,#58342));
#12221=EDGE_LOOP('',(#58343,#58344,#58345,#58346));
#12222=EDGE_LOOP('',(#58347,#58348,#58349,#58350));
#12223=EDGE_LOOP('',(#58351,#58352,#58353,#58354));
#12224=EDGE_LOOP('',(#58355,#58356,#58357,#58358));
#12225=EDGE_LOOP('',(#58359,#58360,#58361,#58362));
#12226=EDGE_LOOP('',(#58363,#58364,#58365,#58366));
#12227=EDGE_LOOP('',(#58367,#58368,#58369,#58370));
#12228=EDGE_LOOP('',(#58371,#58372,#58373,#58374));
#12229=EDGE_LOOP('',(#58375,#58376,#58377,#58378));
#12230=EDGE_LOOP('',(#58379,#58380,#58381,#58382));
#12231=EDGE_LOOP('',(#58383,#58384,#58385,#58386,#58387,#58388,#58389,#58390,
#58391,#58392,#58393,#58394));
#12232=EDGE_LOOP('',(#58395,#58396,#58397,#58398,#58399));
#12233=EDGE_LOOP('',(#58400,#58401,#58402,#58403,#58404));
#12234=EDGE_LOOP('',(#58405));
#12235=EDGE_LOOP('',(#58406,#58407,#58408,#58409));
#12236=EDGE_LOOP('',(#58410,#58411,#58412,#58413));
#12237=EDGE_LOOP('',(#58414,#58415,#58416,#58417));
#12238=EDGE_LOOP('',(#58418,#58419,#58420,#58421));
#12239=EDGE_LOOP('',(#58422,#58423,#58424,#58425));
#12240=EDGE_LOOP('',(#58426,#58427,#58428,#58429,#58430,#58431,#58432,#58433,
#58434,#58435,#58436,#58437,#58438,#58439,#58440,#58441,#58442,#58443,#58444,
#58445,#58446,#58447,#58448,#58449,#58450,#58451,#58452,#58453,#58454,#58455,
#58456,#58457,#58458,#58459,#58460,#58461,#58462,#58463,#58464,#58465,#58466,
#58467,#58468,#58469,#58470,#58471,#58472,#58473,#58474,#58475,#58476,#58477,
#58478,#58479,#58480,#58481,#58482,#58483,#58484,#58485));
#12241=EDGE_LOOP('',(#58486));
#12242=EDGE_LOOP('',(#58487));
#12243=EDGE_LOOP('',(#58488,#58489,#58490,#58491,#58492,#58493,#58494,#58495,
#58496,#58497,#58498,#58499,#58500,#58501,#58502,#58503,#58504,#58505,#58506,
#58507,#58508,#58509,#58510,#58511,#58512,#58513,#58514,#58515,#58516,#58517,
#58518,#58519,#58520,#58521,#58522,#58523,#58524,#58525,#58526,#58527,#58528,
#58529,#58530,#58531,#58532,#58533,#58534,#58535,#58536,#58537,#58538,#58539,
#58540,#58541,#58542,#58543,#58544,#58545,#58546,#58547));
#12244=EDGE_LOOP('',(#58548));
#12245=EDGE_LOOP('',(#58549,#58550,#58551,#58552));
#12246=EDGE_LOOP('',(#58553,#58554,#58555,#58556));
#12247=EDGE_LOOP('',(#58557,#58558,#58559,#58560));
#12248=EDGE_LOOP('',(#58561,#58562,#58563,#58564));
#12249=EDGE_LOOP('',(#58565,#58566,#58567,#58568));
#12250=EDGE_LOOP('',(#58569,#58570,#58571,#58572));
#12251=EDGE_LOOP('',(#58573,#58574,#58575,#58576));
#12252=EDGE_LOOP('',(#58577,#58578,#58579,#58580));
#12253=EDGE_LOOP('',(#58581,#58582,#58583,#58584));
#12254=EDGE_LOOP('',(#58585,#58586,#58587,#58588));
#12255=EDGE_LOOP('',(#58589,#58590,#58591,#58592));
#12256=EDGE_LOOP('',(#58593,#58594,#58595,#58596));
#12257=EDGE_LOOP('',(#58597,#58598,#58599,#58600));
#12258=EDGE_LOOP('',(#58601,#58602,#58603,#58604));
#12259=EDGE_LOOP('',(#58605,#58606,#58607,#58608));
#12260=EDGE_LOOP('',(#58609,#58610,#58611,#58612));
#12261=EDGE_LOOP('',(#58613,#58614,#58615,#58616));
#12262=EDGE_LOOP('',(#58617,#58618,#58619,#58620));
#12263=EDGE_LOOP('',(#58621,#58622,#58623,#58624));
#12264=EDGE_LOOP('',(#58625,#58626,#58627,#58628));
#12265=EDGE_LOOP('',(#58629,#58630,#58631,#58632));
#12266=EDGE_LOOP('',(#58633,#58634,#58635,#58636));
#12267=EDGE_LOOP('',(#58637,#58638,#58639,#58640));
#12268=EDGE_LOOP('',(#58641,#58642,#58643,#58644));
#12269=EDGE_LOOP('',(#58645,#58646,#58647,#58648));
#12270=EDGE_LOOP('',(#58649,#58650,#58651,#58652));
#12271=EDGE_LOOP('',(#58653,#58654,#58655,#58656));
#12272=EDGE_LOOP('',(#58657,#58658,#58659,#58660));
#12273=EDGE_LOOP('',(#58661,#58662,#58663,#58664));
#12274=EDGE_LOOP('',(#58665,#58666,#58667,#58668));
#12275=EDGE_LOOP('',(#58669,#58670,#58671,#58672));
#12276=EDGE_LOOP('',(#58673,#58674,#58675,#58676));
#12277=EDGE_LOOP('',(#58677,#58678,#58679,#58680));
#12278=EDGE_LOOP('',(#58681,#58682,#58683,#58684));
#12279=EDGE_LOOP('',(#58685,#58686,#58687,#58688));
#12280=EDGE_LOOP('',(#58689,#58690,#58691,#58692));
#12281=EDGE_LOOP('',(#58693,#58694,#58695,#58696));
#12282=EDGE_LOOP('',(#58697,#58698,#58699,#58700));
#12283=EDGE_LOOP('',(#58701,#58702,#58703,#58704));
#12284=EDGE_LOOP('',(#58705,#58706,#58707,#58708));
#12285=EDGE_LOOP('',(#58709,#58710,#58711,#58712));
#12286=EDGE_LOOP('',(#58713,#58714,#58715,#58716));
#12287=EDGE_LOOP('',(#58717,#58718,#58719,#58720));
#12288=EDGE_LOOP('',(#58721,#58722,#58723,#58724));
#12289=EDGE_LOOP('',(#58725,#58726,#58727,#58728));
#12290=EDGE_LOOP('',(#58729,#58730,#58731,#58732));
#12291=EDGE_LOOP('',(#58733,#58734,#58735,#58736));
#12292=EDGE_LOOP('',(#58737,#58738,#58739,#58740));
#12293=EDGE_LOOP('',(#58741,#58742,#58743,#58744));
#12294=EDGE_LOOP('',(#58745,#58746,#58747,#58748));
#12295=EDGE_LOOP('',(#58749,#58750,#58751,#58752));
#12296=EDGE_LOOP('',(#58753,#58754,#58755,#58756));
#12297=EDGE_LOOP('',(#58757,#58758,#58759,#58760));
#12298=EDGE_LOOP('',(#58761,#58762,#58763,#58764));
#12299=EDGE_LOOP('',(#58765,#58766,#58767,#58768));
#12300=EDGE_LOOP('',(#58769,#58770,#58771,#58772));
#12301=EDGE_LOOP('',(#58773,#58774,#58775,#58776));
#12302=EDGE_LOOP('',(#58777,#58778,#58779,#58780));
#12303=EDGE_LOOP('',(#58781,#58782,#58783,#58784));
#12304=EDGE_LOOP('',(#58785,#58786,#58787,#58788));
#12305=EDGE_LOOP('',(#58789,#58790,#58791,#58792,#58793));
#12306=EDGE_LOOP('',(#58794,#58795,#58796,#58797,#58798));
#12307=EDGE_LOOP('',(#58799,#58800,#58801,#58802,#58803,#58804));
#12308=EDGE_LOOP('',(#58805,#58806,#58807,#58808,#58809));
#12309=EDGE_LOOP('',(#58810,#58811,#58812,#58813,#58814));
#12310=EDGE_LOOP('',(#58815,#58816,#58817,#58818,#58819));
#12311=EDGE_LOOP('',(#58820,#58821,#58822,#58823,#58824,#58825));
#12312=EDGE_LOOP('',(#58826,#58827,#58828,#58829,#58830));
#12313=EDGE_LOOP('',(#58831,#58832,#58833,#58834,#58835));
#12314=EDGE_LOOP('',(#58836,#58837,#58838,#58839,#58840,#58841));
#12315=EDGE_LOOP('',(#58842,#58843,#58844,#58845,#58846));
#12316=EDGE_LOOP('',(#58847,#58848,#58849,#58850,#58851));
#12317=EDGE_LOOP('',(#58852,#58853,#58854,#58855,#58856,#58857));
#12318=EDGE_LOOP('',(#58858,#58859,#58860,#58861,#58862));
#12319=EDGE_LOOP('',(#58863,#58864,#58865,#58866,#58867));
#12320=EDGE_LOOP('',(#58868,#58869,#58870,#58871,#58872,#58873));
#12321=EDGE_LOOP('',(#58874,#58875,#58876,#58877,#58878));
#12322=EDGE_LOOP('',(#58879,#58880,#58881,#58882,#58883));
#12323=EDGE_LOOP('',(#58884,#58885,#58886,#58887,#58888,#58889));
#12324=EDGE_LOOP('',(#58890,#58891,#58892,#58893,#58894));
#12325=EDGE_LOOP('',(#58895,#58896,#58897,#58898,#58899));
#12326=EDGE_LOOP('',(#58900,#58901,#58902,#58903,#58904,#58905));
#12327=EDGE_LOOP('',(#58906,#58907,#58908,#58909,#58910));
#12328=EDGE_LOOP('',(#58911,#58912,#58913,#58914,#58915));
#12329=EDGE_LOOP('',(#58916,#58917,#58918,#58919,#58920,#58921));
#12330=EDGE_LOOP('',(#58922,#58923,#58924,#58925,#58926));
#12331=EDGE_LOOP('',(#58927,#58928,#58929,#58930,#58931));
#12332=EDGE_LOOP('',(#58932,#58933,#58934,#58935,#58936,#58937));
#12333=EDGE_LOOP('',(#58938,#58939,#58940,#58941,#58942));
#12334=EDGE_LOOP('',(#58943,#58944,#58945,#58946,#58947));
#12335=EDGE_LOOP('',(#58948,#58949,#58950,#58951,#58952,#58953));
#12336=EDGE_LOOP('',(#58954,#58955,#58956,#58957,#58958));
#12337=EDGE_LOOP('',(#58959,#58960,#58961,#58962,#58963));
#12338=EDGE_LOOP('',(#58964,#58965,#58966,#58967,#58968,#58969));
#12339=EDGE_LOOP('',(#58970,#58971,#58972,#58973,#58974));
#12340=EDGE_LOOP('',(#58975,#58976,#58977,#58978,#58979));
#12341=EDGE_LOOP('',(#58980,#58981,#58982,#58983,#58984,#58985));
#12342=EDGE_LOOP('',(#58986,#58987,#58988,#58989,#58990));
#12343=EDGE_LOOP('',(#58991,#58992,#58993,#58994,#58995));
#12344=EDGE_LOOP('',(#58996,#58997,#58998,#58999,#59000,#59001));
#12345=EDGE_LOOP('',(#59002,#59003,#59004,#59005,#59006));
#12346=EDGE_LOOP('',(#59007,#59008,#59009,#59010,#59011));
#12347=EDGE_LOOP('',(#59012,#59013,#59014,#59015));
#12348=EDGE_LOOP('',(#59016,#59017,#59018,#59019,#59020,#59021));
#12349=EDGE_LOOP('',(#59022,#59023,#59024,#59025,#59026));
#12350=EDGE_LOOP('',(#59027,#59028,#59029,#59030,#59031));
#12351=EDGE_LOOP('',(#59032,#59033,#59034,#59035,#59036));
#12352=EDGE_LOOP('',(#59037,#59038,#59039,#59040));
#12353=EDGE_LOOP('',(#59041,#59042,#59043,#59044));
#12354=EDGE_LOOP('',(#59045));
#18132=CIRCLE('',#94908,1.2645);
#18133=CIRCLE('',#94912,1.2645);
#18134=CIRCLE('',#94914,1.2645);
#18135=CIRCLE('',#94918,1.2645);
#18136=CIRCLE('',#94920,1.543);
#18137=CIRCLE('',#94924,1.543);
#18138=CIRCLE('',#94926,1.543);
#18139=CIRCLE('',#94930,1.543);
#18140=CIRCLE('',#94936,1.1);
#18141=CIRCLE('',#94937,3.40000000056584);
#18142=CIRCLE('',#94938,1.1);
#18143=CIRCLE('',#94939,18.25);
#18144=CIRCLE('',#94941,1.1);
#18145=CIRCLE('',#94942,3.39999999943896);
#18146=CIRCLE('',#94943,1.1);
#18147=CIRCLE('',#94944,18.25);
#18148=CIRCLE('',#94945,18.25);
#18149=CIRCLE('',#94947,8.);
#18150=CIRCLE('',#94948,7.9);
#18151=CIRCLE('',#94950,8.);
#18152=CIRCLE('',#94952,1.5);
#18153=CIRCLE('',#94954,18.25);
#18154=CIRCLE('',#94955,18.15);
#18155=CIRCLE('',#94956,18.25);
#18156=CIRCLE('',#94958,18.25);
#18157=CIRCLE('',#94959,18.25);
#18158=CIRCLE('',#94961,17.5);
#18159=CIRCLE('',#94963,18.25);
#18160=CIRCLE('',#94964,18.15);
#18161=CIRCLE('',#94965,18.25);
#18162=CIRCLE('',#94967,18.25);
#18163=CIRCLE('',#94969,17.5);
#18164=CIRCLE('',#94971,2.5);
#18165=CIRCLE('',#94972,2.6);
#18166=CIRCLE('',#94974,18.15);
#18167=CIRCLE('',#94976,2.5);
#18168=CIRCLE('',#94979,1.);
#18169=CIRCLE('',#94982,3.50000000056584);
#18170=CIRCLE('',#94985,1.);
#18171=CIRCLE('',#94987,1.);
#18172=CIRCLE('',#94990,3.49999999943895);
#18173=CIRCLE('',#94993,1.);
#18174=CIRCLE('',#94996,3.49999999943895);
#18175=CIRCLE('',#94997,3.39999999943896);
#18176=CIRCLE('',#95000,1.);
#18177=CIRCLE('',#95001,1.1);
#18178=CIRCLE('',#95003,18.15);
#18179=CIRCLE('',#95005,1.);
#18180=CIRCLE('',#95006,1.1);
#18181=CIRCLE('',#95009,3.50000000056584);
#18182=CIRCLE('',#95010,3.40000000056584);
#18183=CIRCLE('',#95013,1.);
#18184=CIRCLE('',#95014,1.1);
#18185=CIRCLE('',#95016,18.15);
#18186=CIRCLE('',#95018,1.);
#18187=CIRCLE('',#95019,1.1);
#18188=CIRCLE('',#95030,1.);
#18189=CIRCLE('',#95031,1.3);
#18190=CIRCLE('',#95033,1.);
#18191=CIRCLE('',#95035,1.875);
#18192=CIRCLE('',#95036,3.);
#18193=CIRCLE('',#95037,1.875);
#18194=CIRCLE('',#95038,3.);
#18195=CIRCLE('',#95039,1.875);
#18196=CIRCLE('',#95040,3.);
#18197=CIRCLE('',#95041,1.875);
#18198=CIRCLE('',#95042,3.);
#18199=CIRCLE('',#95043,1.875);
#18200=CIRCLE('',#95044,3.);
#18201=CIRCLE('',#95045,1.875);
#18202=CIRCLE('',#95046,3.);
#18203=CIRCLE('',#95047,1.875);
#18204=CIRCLE('',#95048,3.);
#18205=CIRCLE('',#95049,1.875);
#18206=CIRCLE('',#95050,3.);
#18207=CIRCLE('',#95051,1.875);
#18208=CIRCLE('',#95052,3.);
#18209=CIRCLE('',#95053,1.875);
#18210=CIRCLE('',#95054,3.);
#18211=CIRCLE('',#95057,1.875);
#18212=CIRCLE('',#95058,3.);
#18213=CIRCLE('',#95059,1.875);
#18214=CIRCLE('',#95060,3.);
#18215=CIRCLE('',#95061,1.875);
#18216=CIRCLE('',#95062,3.);
#18217=CIRCLE('',#95063,1.875);
#18218=CIRCLE('',#95064,3.);
#18219=CIRCLE('',#95065,1.875);
#18220=CIRCLE('',#95066,3.);
#18221=CIRCLE('',#95067,1.875);
#18222=CIRCLE('',#95068,3.);
#18223=CIRCLE('',#95069,1.875);
#18224=CIRCLE('',#95070,3.);
#18225=CIRCLE('',#95071,1.875);
#18226=CIRCLE('',#95072,3.);
#18227=CIRCLE('',#95073,1.875);
#18228=CIRCLE('',#95074,3.);
#18229=CIRCLE('',#95075,1.875);
#18230=CIRCLE('',#95076,3.);
#18231=CIRCLE('',#95077,1.5);
#18232=CIRCLE('',#95119,17.5);
#18233=CIRCLE('',#95120,17.4);
#18234=CIRCLE('',#95121,17.5);
#18235=CIRCLE('',#95123,17.5);
#18236=CIRCLE('',#95124,17.5);
#18237=CIRCLE('',#95126,17.5);
#18238=CIRCLE('',#95127,17.5);
#18239=CIRCLE('',#95130,17.5);
#18240=CIRCLE('',#95131,17.4);
#18241=CIRCLE('',#95132,17.5);
#18242=CIRCLE('',#95135,17.5);
#18243=CIRCLE('',#95136,17.5);
#18244=CIRCLE('',#95138,17.5);
#18245=CIRCLE('',#95139,17.4);
#18246=CIRCLE('',#95140,17.5);
#18247=CIRCLE('',#95143,17.5);
#18248=CIRCLE('',#95144,17.5);
#18249=CIRCLE('',#95146,17.5);
#18250=CIRCLE('',#95147,17.4);
#18251=CIRCLE('',#95148,17.5);
#18252=CIRCLE('',#95151,17.5);
#18253=CIRCLE('',#95152,17.5);
#18254=CIRCLE('',#95154,17.5);
#18255=CIRCLE('',#95155,17.4);
#18256=CIRCLE('',#95156,17.5);
#18257=CIRCLE('',#95159,17.5);
#18258=CIRCLE('',#95160,17.5);
#18259=CIRCLE('',#95162,17.5);
#18260=CIRCLE('',#95163,17.4);
#18261=CIRCLE('',#95164,17.5);
#18262=CIRCLE('',#95167,17.5);
#18263=CIRCLE('',#95168,17.5);
#18264=CIRCLE('',#95170,17.5);
#18265=CIRCLE('',#95171,17.4);
#18266=CIRCLE('',#95172,17.5);
#18267=CIRCLE('',#95175,17.5);
#18268=CIRCLE('',#95176,17.5);
#18269=CIRCLE('',#95178,17.5);
#18270=CIRCLE('',#95179,17.4);
#18271=CIRCLE('',#95180,17.5);
#18272=CIRCLE('',#95183,17.5);
#18273=CIRCLE('',#95184,17.5);
#18274=CIRCLE('',#95186,17.5);
#18275=CIRCLE('',#95187,17.4);
#18276=CIRCLE('',#95188,17.5);
#18277=CIRCLE('',#95191,17.5);
#18278=CIRCLE('',#95192,17.5);
#18279=CIRCLE('',#95194,17.5);
#18280=CIRCLE('',#95195,17.4);
#18281=CIRCLE('',#95196,17.5);
#18282=CIRCLE('',#95199,17.5);
#18283=CIRCLE('',#95200,17.5);
#18284=CIRCLE('',#95202,17.5);
#18285=CIRCLE('',#95203,17.4);
#18286=CIRCLE('',#95204,17.5);
#18287=CIRCLE('',#95207,17.5);
#18288=CIRCLE('',#95208,17.5);
#18289=CIRCLE('',#95210,17.5);
#18290=CIRCLE('',#95211,17.4);
#18291=CIRCLE('',#95212,17.5);
#18292=CIRCLE('',#95215,17.5);
#18293=CIRCLE('',#95216,17.5);
#18294=CIRCLE('',#95218,17.5);
#18295=CIRCLE('',#95219,17.4);
#18296=CIRCLE('',#95220,17.5);
#18297=CIRCLE('',#95223,17.5);
#18298=CIRCLE('',#95224,17.5);
#18299=CIRCLE('',#95226,17.5);
#18300=CIRCLE('',#95227,17.4);
#18301=CIRCLE('',#95228,17.5);
#18302=CIRCLE('',#95232,17.5);
#18303=CIRCLE('',#95233,17.5);
#18304=CIRCLE('',#95235,17.5);
#18305=CIRCLE('',#95236,17.5);
#18306=CIRCLE('',#95237,17.4);
#23498=B_SPLINE_CURVE_WITH_KNOTS('',3,(#130727,#130728,#130729,#130730,
#130731,#130732,#130733,#130734,#130735,#130736,#130737,#130738,#130739,
#130740,#130741,#130742,#130743,#130744,#130745,#130746,#130747,#130748,
#130749,#130750,#130751,#130752,#130753,#130754,#130755,#130756,#130757,
#130758,#130759,#130760,#130761,#130762,#130763,#130764,#130765,#130766,
#130767,#130768,#130769,#130770,#130771,#130772,#130773,#130774,#130775,
#130776,#130777,#130778,#130779,#130780,#130781,#130782,#130783,#130784,
#130785,#130786,#130787,#130788,#130789,#130790,#130791,#130792,#130793),
 .UNSPECIFIED.,.F.,.F.,(4,3,3,3,3,3,3,3,3,3,3,3,3,3,3,3,3,3,3,3,3,3,4),
(24.5160776815829,24.6338502836512,24.7515779097144,24.8693943986912,24.9872495119034,
25.105327266425,25.2137469589919,25.2137913118699,25.3221913605844,25.3350114624077,
25.4518815112335,25.5686444395478,25.6853513110055,25.8020530911996,25.9188834125999,
26.0357913091352,26.1452292168737,26.1529168472848,26.1835170015641,26.1835525161726,
26.3016558198144,26.3399124732618,26.4422968683701),.UNSPECIFIED.);
#23499=B_SPLINE_CURVE_WITH_KNOTS('',3,(#130795,#130796,#130797,#130798,
#130799,#130800,#130801,#130802,#130803,#130804,#130805,#130806,#130807,
#130808,#130809,#130810,#130811,#130812,#130813,#130814,#130815,#130816),
 .UNSPECIFIED.,.F.,.F.,(4,3,3,3,3,3,3,4),(-0.0902749387754822,-0.0742826152768497,
-0.0647281330592198,-0.0554146586505969,-0.0451640473161138,-0.033509184847726,
-0.00675287661166353,0.),.UNSPECIFIED.);
#23500=B_SPLINE_CURVE_WITH_KNOTS('',3,(#130819,#130820,#130821,#130822,
#130823,#130824,#130825,#130826,#130827,#130828,#130829,#130830,#130831,
#130832,#130833,#130834,#130835,#130836,#130837,#130838,#130839,#130840,
#130841,#130842,#130843,#130844,#130845,#130846,#130847,#130848,#130849,
#130850,#130851,#130852,#130853,#130854,#130855,#130856,#130857,#130858,
#130859,#130860,#130861,#130862,#130863,#130864,#130865,#130866,#130867,
#130868,#130869,#130870,#130871,#130872,#130873,#130874,#130875,#130876,
#130877,#130878,#130879,#130880,#130881,#130882,#130883,#130884,#130885,
#130886,#130887,#130888,#130889,#130890,#130891,#130892,#130893,#130894,
#130895,#130896,#130897,#130898,#130899,#130900,#130901,#130902),
 .UNSPECIFIED.,.F.,.F.,(4,2,2,2,2,2,2,2,2,2,2,2,2,2,2,2,2,2,2,2,2,2,2,2,
2,2,2,2,2,2,2,2,2,2,2,2,2,2,2,2,2,4),(-3.18439516658457,-3.15974881539495,
-3.14750129282652,-3.13703041818299,-3.12844802307121,-3.11639166588861,
-3.08592199300131,-3.07681556285727,-3.07174260228611,-3.06513991741923,
-3.03589139873531,-3.02003342723502,-3.01118711648019,-3.0019557243139,
-2.97314287852745,-2.96147727551602,-2.9533181918626,-2.94843288600149,
-2.94182402102507,-2.91271400453299,-2.89692673378685,-2.88814855910042,
-2.87904381531293,-2.8610699969371,-2.84219439832436,-2.83162052918509,
-2.82647232988103,-2.82058879757083,-2.79817695746129,-2.77549565690187,
-2.76631068751743,-2.75747581459958,-2.74152565839784,-2.72017905583269,
-2.71215881373051,-2.70573910057196,-2.70073398133747,-2.69173779062522,
-2.66793712484695,-2.65135784589242,-2.64248009746824,-2.63341280352093),
 .UNSPECIFIED.);
#23501=B_SPLINE_CURVE_WITH_KNOTS('',3,(#130908,#130909,#130910,#130911,
#130912,#130913,#130914,#130915,#130916,#130917,#130918,#130919,#130920,
#130921,#130922,#130923,#130924,#130925,#130926,#130927,#130928,#130929,
#130930,#130931,#130932,#130933,#130934,#130935,#130936,#130937,#130938,
#130939,#130940,#130941,#130942,#130943,#130944,#130945,#130946,#130947,
#130948,#130949,#130950,#130951,#130952,#130953,#130954,#130955,#130956,
#130957,#130958,#130959,#130960,#130961,#130962,#130963,#130964,#130965,
#130966,#130967,#130968,#130969,#130970,#130971,#130972,#130973,#130974,
#130975,#130976,#130977),.UNSPECIFIED.,.F.,.F.,(4,3,3,3,3,3,3,3,3,3,3,3,
3,3,3,3,3,3,3,3,3,3,3,4),(18.2318964876154,18.3499056532152,18.4254225164394,
18.4254628817511,18.534901772586,18.5466830322889,18.6645202599371,18.7822476497643,
18.89991442255,19.0237418384259,19.1415118943581,19.2593532998693,19.3681535102728,
19.3773894458933,19.3951836495535,19.3952240860538,19.5034482315185,19.5116532718969,
19.6279187937169,19.7440728916638,19.8602107593755,19.9763360740262,20.0925768794781,
20.1591190620682),.UNSPECIFIED.);
#23502=B_SPLINE_CURVE_WITH_KNOTS('',3,(#130978,#130979,#130980,#130981,
#130982,#130983,#130984,#130985,#130986,#130987,#130988,#130989,#130990,
#130991,#130992,#130993,#130994,#130995,#130996,#130997,#130998,#130999,
#131000,#131001,#131002,#131003,#131004,#131005,#131006,#131007,#131008,
#131009,#131010,#131011,#131012,#131013,#131014,#131015,#131016,#131017,
#131018,#131019,#131020,#131021,#131022,#131023,#131024,#131025,#131026,
#131027,#131028,#131029,#131030,#131031,#131032,#131033,#131034,#131035,
#131036,#131037,#131038,#131039,#131040,#131041,#131042,#131043,#131044,
#131045,#131046,#131047,#131048,#131049,#131050,#131051,#131052,#131053,
#131054,#131055,#131056,#131057,#131058,#131059,#131060,#131061,#131062,
#131063,#131064,#131065,#131066,#131067,#131068,#131069,#131070,#131071,
#131072,#131073,#131074,#131075,#131076,#131077,#131078,#131079,#131080,
#131081,#131082,#131083,#131084,#131085,#131086,#131087,#131088,#131089,
#131090,#131091,#131092,#131093,#131094,#131095,#131096,#131097,#131098,
#131099,#131100,#131101,#131102,#131103,#131104,#131105,#131106,#131107,
#131108,#131109,#131110,#131111,#131112,#131113,#131114,#131115,#131116,
#131117,#131118,#131119,#131120,#131121,#131122,#131123,#131124,#131125,
#131126,#131127,#131128,#131129,#131130,#131131,#131132,#131133,#131134,
#131135,#131136,#131137,#131138,#131139,#131140,#131141,#131142,#131143,
#131144,#131145,#131146),.UNSPECIFIED.,.F.,.F.,(4,3,3,3,3,3,3,3,3,3,3,3,
3,3,3,3,3,3,3,3,3,3,3,3,3,3,3,3,3,3,3,3,3,3,3,3,3,3,3,3,3,3,3,3,3,3,3,3,
3,3,3,3,3,3,3,3,4),(20.1591190625159,20.2764390861516,20.3187722441127,
20.3649448921207,20.3649852903565,20.4744178307227,20.4862054408943,20.6040549110511,
20.7217943849732,20.8394730597834,20.9632914185023,21.081072765058,21.198925234886,
21.3077530804529,21.3169720402184,21.3347063043336,21.3347464946591,21.4442281539202,
21.4559666451969,21.5738204779957,21.6915646661758,21.8092483924545,21.9330632190813,
22.0508503771043,22.1687089093655,22.2774753621084,22.2867620791089,22.3044668695445,
22.3045076989618,22.4138254986466,22.4257278494996,22.5434478115752,22.6610580097667,
22.7786079083108,22.8961468703754,23.0137997695757,23.1315225935855,23.2408830638024,
23.2494441255917,23.2742286828635,23.2742689032645,23.3837602833423,23.3954890538023,
23.5135003420354,23.6314006664449,23.7492388874001,23.8729366924419,23.9908721599826,
24.10887664777,24.2178717905383,24.227071312369,24.243991123088,24.2440301075672,
24.3536754995663,24.3621270739351,24.480036883431,24.5160776809557),
 .UNSPECIFIED.);
#23503=B_SPLINE_CURVE_WITH_KNOTS('',3,(#131147,#131148,#131149,#131150,
#131151,#131152,#131153,#131154,#131155,#131156,#131157,#131158,#131159,
#131160,#131161,#131162,#131163,#131164,#131165,#131166,#131167,#131168,
#131169,#131170,#131171,#131172,#131173,#131174,#131175,#131176,#131177,
#131178,#131179,#131180,#131181,#131182,#131183,#131184,#131185,#131186,
#131187,#131188,#131189,#131190,#131191,#131192,#131193,#131194,#131195,
#131196,#131197,#131198,#131199,#131200,#131201,#131202,#131203,#131204,
#131205,#131206,#131207,#131208,#131209,#131210,#131211,#131212,#131213,
#131214,#131215,#131216,#131217,#131218,#131219,#131220,#131221,#131222,
#131223,#131224,#131225,#131226,#131227,#131228,#131229,#131230,#131231,
#131232,#131233,#131234,#131235,#131236,#131237,#131238,#131239,#131240,
#131241,#131242,#131243,#131244,#131245,#131246,#131247,#131248,#131249,
#131250,#131251,#131252,#131253,#131254,#131255,#131256,#131257,#131258,
#131259,#131260,#131261,#131262,#131263,#131264,#131265,#131266,#131267,
#131268,#131269,#131270,#131271,#131272,#131273,#131274,#131275,#131276,
#131277,#131278),.UNSPECIFIED.,.F.,.F.,(4,2,2,2,2,2,2,2,2,2,2,2,2,2,2,2,
2,2,2,2,2,2,2,2,2,2,2,2,2,2,2,2,2,2,2,2,2,2,2,2,2,2,2,2,2,2,2,2,2,2,2,2,
2,2,2,2,2,2,2,2,2,2,2,2,2,4),(-2.63341280352093,-2.63338908590916,-2.61475077252263,
-2.59625974636104,-2.58578420982809,-2.58063284435739,-2.57470277043636,
-2.5603653957494,-2.54033455876387,-2.53026043017817,-2.52097003372362,
-2.51223669831331,-2.49728887792193,-2.47471711241325,-2.46325775592071,
-2.45800484991181,-2.45225752364046,-2.43791426300124,-2.41757964125372,
-2.40744820567261,-2.39812483100095,-2.38939762360827,-2.37457182362478,
-2.35186459507239,-2.34365529463354,-2.33713766240529,-2.33216521116693,
-2.32346121809268,-2.2995507987335,-2.2875813199158,-2.27729863580044,-2.26882022586542,
-2.25694334169315,-2.23001808279554,-2.2212988600583,-2.21451702781106,
-2.20958429245329,-2.20138147088039,-2.17574348926931,-2.16413634608837,
-2.1540388650897,-2.14553861920783,-2.13331947430134,-2.10696134396377,
-2.09830456306287,-2.09155462124085,-2.0866177365907,-2.07835966124171,
-2.05425218617961,-2.03700607791523,-2.02807903382094,-2.01905076582828,
-1.98720884630738,-1.97243327564618,-1.96690070443741,-1.96147826300303,
-1.95047478829063,-1.92724571493476,-1.91274763706247,-1.90405001510231,
-1.89466835474604,-1.86490369174868,-1.85426067665749,-1.84655505358699,
-1.84164637788602,-1.83698289437714),.UNSPECIFIED.);
#23504=B_SPLINE_CURVE_WITH_KNOTS('',3,(#131284,#131285,#131286,#131287,
#131288,#131289,#131290,#131291,#131292,#131293,#131294,#131295,#131296,
#131297,#131298,#131299,#131300,#131301,#131302,#131303,#131304,#131305,
#131306,#131307,#131308,#131309,#131310,#131311,#131312,#131313,#131314,
#131315,#131316,#131317,#131318,#131319,#131320,#131321,#131322,#131323,
#131324,#131325,#131326,#131327,#131328,#131329,#131330,#131331,#131332,
#131333,#131334,#131335,#131336,#131337,#131338,#131339,#131340,#131341,
#131342,#131343,#131344,#131345,#131346,#131347,#131348,#131349,#131350,
#131351,#131352,#131353,#131354,#131355,#131356),.UNSPECIFIED.,.F.,.F.,
(4,3,3,3,3,3,3,3,3,3,3,3,3,3,3,3,3,3,3,3,3,3,3,3,4),(11.949635603067,12.0673156376958,
12.1849657013768,12.3027149435704,12.4205166426525,12.5385271257885,12.6068552638494,
12.6068956559349,12.7163278647347,12.7281158064727,12.8459491616131,12.9636726575015,
13.081335523404,13.2051658576124,13.3229320283064,13.4407695618705,13.549573048494,
13.5588018855446,13.5766164679027,13.5766568602376,13.6924275886706,13.7171311440579,
13.8384365525919,13.8560591163181,13.8759337548445),.UNSPECIFIED.);
#23505=B_SPLINE_CURVE_WITH_KNOTS('',3,(#131357,#131358,#131359,#131360,
#131361,#131362,#131363,#131364,#131365,#131366,#131367,#131368,#131369,
#131370,#131371,#131372,#131373,#131374,#131375,#131376,#131377,#131378,
#131379,#131380,#131381,#131382,#131383,#131384,#131385,#131386,#131387,
#131388,#131389,#131390,#131391,#131392,#131393,#131394,#131395,#131396,
#131397,#131398,#131399,#131400,#131401,#131402,#131403,#131404,#131405,
#131406,#131407,#131408,#131409,#131410,#131411,#131412,#131413,#131414,
#131415,#131416,#131417,#131418,#131419,#131420,#131421,#131422,#131423,
#131424,#131425,#131426,#131427,#131428,#131429,#131430,#131431,#131432,
#131433,#131434,#131435,#131436,#131437,#131438,#131439,#131440,#131441,
#131442,#131443,#131444,#131445,#131446,#131447,#131448,#131449,#131450,
#131451,#131452,#131453,#131454,#131455,#131456,#131457,#131458,#131459,
#131460,#131461,#131462,#131463,#131464,#131465,#131466,#131467,#131468,
#131469,#131470,#131471,#131472,#131473,#131474,#131475,#131476,#131477,
#131478,#131479,#131480,#131481,#131482,#131483,#131484,#131485,#131486,
#131487,#131488,#131489,#131490,#131491,#131492,#131493,#131494,#131495,
#131496,#131497,#131498,#131499,#131500,#131501,#131502,#131503,#131504,
#131505,#131506,#131507,#131508,#131509,#131510),.UNSPECIFIED.,.F.,.F.,
(4,3,3,3,3,3,3,3,3,3,3,3,3,3,3,3,3,3,3,3,3,3,3,3,3,3,3,3,3,3,3,3,3,3,3,
3,3,3,3,3,3,3,3,3,3,3,3,3,3,3,3,4),(13.8759337553363,13.9931001932589,14.1102297434989,
14.227456018938,14.344730230585,14.4622230561964,14.5463776723912,14.5464180645403,
14.6558502206054,14.6676382150781,14.7854717016337,14.9031953297728,15.0208583284965,
15.1446885635831,15.2624548668063,15.3802925326214,15.4890963578799,15.4983249871425,
15.5161388802809,15.516179268843,15.6256123754232,15.6373994193808,15.7552334260967,
15.8729575772568,15.9906211007147,16.1144509438225,16.2322177687725,16.3500559544883,
16.4588592317635,16.4680889221782,16.4859000772313,16.4859404731457,16.5953716279568,
16.6071606236835,16.7249924873266,16.8427144992418,16.9603758917638,17.0842073381849,
17.2019720818873,17.3198082065096,17.4286109026081,17.4378391578116,17.4556612819127,
17.4557016774484,17.5649968567153,17.5737108697352,17.6915524576925,17.8092758653084,
17.9269654710807,18.0446320306057,18.1623925787244,18.2318964870053),
 .UNSPECIFIED.);
#23506=B_SPLINE_CURVE_WITH_KNOTS('',3,(#131511,#131512,#131513,#131514,
#131515,#131516,#131517,#131518,#131519,#131520,#131521,#131522,#131523,
#131524,#131525,#131526,#131527,#131528,#131529,#131530,#131531,#131532,
#131533,#131534,#131535,#131536,#131537,#131538,#131539,#131540,#131541,
#131542,#131543,#131544,#131545,#131546,#131547,#131548,#131549,#131550,
#131551,#131552,#131553,#131554,#131555,#131556,#131557,#131558,#131559,
#131560,#131561,#131562,#131563,#131564,#131565,#131566,#131567,#131568,
#131569,#131570,#131571,#131572,#131573,#131574,#131575,#131576,#131577,
#131578,#131579,#131580,#131581,#131582,#131583,#131584,#131585,#131586,
#131587,#131588,#131589,#131590,#131591,#131592,#131593,#131594,#131595,
#131596,#131597,#131598,#131599,#131600,#131601,#131602,#131603,#131604,
#131605,#131606,#131607,#131608,#131609,#131610,#131611,#131612,#131613,
#131614,#131615,#131616,#131617,#131618,#131619,#131620,#131621,#131622,
#131623,#131624,#131625,#131626,#131627,#131628,#131629,#131630,#131631,
#131632,#131633,#131634,#131635,#131636),.UNSPECIFIED.,.F.,.F.,(4,2,2,2,
2,2,2,2,2,2,2,2,2,2,2,2,2,2,2,2,2,2,2,2,2,2,2,2,2,2,2,2,2,2,2,2,2,2,2,2,
2,2,2,2,2,2,2,2,2,2,2,2,2,2,2,2,2,2,2,2,2,2,4),(-1.83698289437714,-1.83450952322168,
-1.80608476101656,-1.79042517070769,-1.78162444808961,-1.77243081013779,
-1.7503408384697,-1.73456941244788,-1.7249015434468,-1.71983535496605,-1.71368757517374,
-1.6837109178935,-1.67220860664121,-1.66216542597266,-1.65365749763611,
-1.64132646297389,-1.61515183154271,-1.60298920152642,-1.59766578617113,
-1.59201641470727,-1.57475374211352,-1.5466611850744,-1.53741065722368,
-1.52864837761914,-1.51340581989546,-1.48699773037434,-1.47841600401358,
-1.47345504174387,-1.46688302543023,-1.45856799126273,-1.435069853613,-1.42085695998277,
-1.4122731987527,-1.40286934027383,-1.39258460820883,-1.37134319401564,
-1.35810032092574,-1.35246748979556,-1.34713280090652,-1.33484535845507,
-1.30796723459815,-1.29605786773587,-1.28757933475715,-1.27732000283747,
-1.26539595606936,-1.24153571280251,-1.23276161007615,-1.22778473505187,
-1.22130699705758,-1.21317068503583,-1.19100494486867,-1.17570953094654,
-1.16694325088905,-1.15770293996463,-1.13397037665446,-1.11328131781741,
-1.10727342224715,-1.10215365759373,-1.09197859212924,-1.0745490245242,
-1.05465390886544,-1.04551395773332,-1.04064761107749),.UNSPECIFIED.);
#23507=B_SPLINE_CURVE_WITH_KNOTS('',3,(#131642,#131643,#131644,#131645,
#131646,#131647,#131648,#131649,#131650,#131651,#131652,#131653,#131654,
#131655,#131656,#131657,#131658,#131659,#131660,#131661,#131662,#131663,
#131664,#131665,#131666,#131667,#131668,#131669,#131670,#131671,#131672,
#131673,#131674,#131675,#131676,#131677,#131678,#131679,#131680,#131681,
#131682,#131683),.UNSPECIFIED.,.F.,.F.,(4,2,2,2,2,2,2,2,2,2,2,2,2,2,2,2,
2,2,2,2,4),(-0.244126851835458,-0.242266589745228,-0.232767411029632,-0.20227844630268,
-0.189805359946467,-0.181570707052886,-0.172343713890524,-0.162123567604387,
-0.140240762435818,-0.128266635619279,-0.12281204083496,-0.117496476174122,
-0.105970253642188,-0.0842702830154775,-0.066515665373926,-0.0566811651008963,
-0.0466317253481053,-0.025601938924746,-0.00728212488525174,-0.00327759413548372,
-9.99999999390377E-7),.UNSPECIFIED.);
#23508=B_SPLINE_CURVE_WITH_KNOTS('',3,(#131686,#131687,#131688,#131689,
#131690,#131691,#131692,#131693,#131694,#131695,#131696,#131697,#131698,
#131699,#131700,#131701,#131702,#131703,#131704,#131705,#131706,#131707,
#131708,#131709,#131710,#131711,#131712,#131713,#131714,#131715,#131716,
#131717,#131718,#131719,#131720,#131721,#131722,#131723,#131724,#131725,
#131726,#131727,#131728,#131729,#131730,#131731,#131732,#131733,#131734,
#131735,#131736,#131737,#131738,#131739,#131740,#131741,#131742,#131743,
#131744,#131745,#131746,#131747,#131748,#131749,#131750,#131751,#131752,
#131753,#131754,#131755,#131756,#131757,#131758,#131759,#131760,#131761,
#131762,#131763,#131764,#131765,#131766,#131767,#131768,#131769,#131770,
#131771,#131772,#131773,#131774,#131775,#131776,#131777,#131778,#131779,
#131780,#131781,#131782,#131783,#131784,#131785,#131786,#131787,#131788,
#131789,#131790,#131791,#131792,#131793,#131794,#131795,#131796,#131797,
#131798,#131799,#131800,#131801,#131802,#131803,#131804,#131805,#131806,
#131807,#131808,#131809),.UNSPECIFIED.,.F.,.F.,(4,3,3,3,3,3,3,3,3,3,3,3,
3,3,3,3,3,3,3,3,3,3,3,3,3,3,3,3,3,3,3,3,3,3,3,3,3,3,3,3,3,4),(2.02979676262917,
2.13731224702246,2.25387842932559,2.37034643280507,2.48676778078347,2.60327116203147,
2.71981651592146,2.83656470629628,2.90924454559889,2.90928361290806,3.01897299074406,
3.0305037634459,3.14850451785552,3.26639853642502,3.3842346685647,3.50793720572621,
3.62588111593657,3.74389766548153,3.85268061258365,3.86210939485147,3.87900455825299,
3.87904481721075,3.98841323710296,4.00026496774859,4.11798860660234,4.23560100936115,
4.35315164410215,4.47068987590689,4.58833990365881,4.70605859647816,4.8153662846805,
4.82397422696118,4.84876523421727,4.84880602151344,4.95807676401619,4.96683180286505,
5.08469155674416,5.20243465709765,5.32015563758868,5.43785412192805,5.55567628577564,
5.66554986544235),.UNSPECIFIED.);
#23509=B_SPLINE_CURVE_WITH_KNOTS('',3,(#131815,#131816,#131817,#131818,
#131819,#131820,#131821,#131822,#131823,#131824,#131825,#131826,#131827,
#131828,#131829,#131830,#131831,#131832,#131833,#131834,#131835,#131836,
#131837,#131838,#131839,#131840,#131841,#131842,#131843,#131844,#131845,
#131846,#131847,#131848,#131849,#131850,#131851,#131852,#131853,#131854,
#131855,#131856,#131857,#131858,#131859,#131860,#131861,#131862,#131863,
#131864,#131865,#131866,#131867,#131868,#131869,#131870,#131871,#131872,
#131873,#131874,#131875,#131876,#131877,#131878,#131879,#131880,#131881),
 .UNSPECIFIED.,.F.,.F.,(4,3,3,3,3,3,3,3,3,3,3,3,3,3,3,3,3,3,3,3,3,3,4),
(24.5160781364108,24.6338513924193,24.7515796689379,24.8693967972321,24.9872525443042,
25.1053309156037,25.2137469623114,25.2137913118699,25.3221904411987,25.3350114624077,
25.4518800492476,25.5686415181165,25.68534693484,25.8020472671814,25.9188761600837,
26.0357826375004,26.1452199094595,26.1529067833318,26.1835169867254,26.1835525161726,
26.3016565030475,26.3399218786873,26.4422968782847),.UNSPECIFIED.);
#23510=B_SPLINE_CURVE_WITH_KNOTS('',3,(#131883,#131884,#131885,#131886,
#131887,#131888,#131889,#131890,#131891,#131892,#131893,#131894,#131895,
#131896,#131897,#131898,#131899,#131900,#131901,#131902,#131903,#131904),
 .UNSPECIFIED.,.F.,.F.,(4,3,3,3,3,3,3,4),(-0.0902748495005752,-0.074282404340397,
-0.0647286421966786,-0.0554142010493536,-0.045164026211744,-0.0335103866407499,
-0.00675201620121094,0.),.UNSPECIFIED.);
#23511=B_SPLINE_CURVE_WITH_KNOTS('',3,(#131907,#131908,#131909,#131910,
#131911,#131912,#131913,#131914,#131915,#131916,#131917,#131918,#131919,
#131920,#131921,#131922,#131923,#131924,#131925,#131926,#131927,#131928,
#131929,#131930,#131931,#131932,#131933,#131934,#131935,#131936,#131937,
#131938,#131939,#131940,#131941,#131942,#131943,#131944,#131945,#131946,
#131947,#131948,#131949,#131950,#131951,#131952,#131953,#131954,#131955,
#131956,#131957,#131958,#131959,#131960,#131961,#131962,#131963,#131964,
#131965,#131966,#131967,#131968,#131969,#131970,#131971,#131972,#131973,
#131974,#131975,#131976,#131977,#131978,#131979,#131980,#131981,#131982,
#131983,#131984,#131985,#131986,#131987,#131988,#131989,#131990,#131991,
#131992),.UNSPECIFIED.,.F.,.F.,(4,2,2,2,2,2,2,2,2,2,2,2,2,2,2,2,2,2,2,2,
2,2,2,2,2,2,2,2,2,2,2,2,2,2,2,2,2,2,2,2,2,2,4),(-3.18475804076959,-3.15980016638694,
-3.14273948012479,-3.13374539783552,-3.12454062706717,-3.10423748937383,
-3.08760027365706,-3.07766771004778,-3.07251605124589,-3.06621772700951,
-3.03649018045794,-3.02050583915172,-3.01165074901096,-3.00243773194935,
-2.98151171764926,-2.9592535975697,-2.95250011400159,-2.94757330454844,
-2.93935856742012,-2.91247851666974,-2.89715062959167,-2.88841337344926,
-2.87924916601703,-2.85742178608931,-2.83610768400626,-2.82941275923196,
-2.82448685551502,-2.81623443939348,-2.7921150364245,-2.77989286674714,
-2.76947546235326,-2.76098995901444,-2.74925789120506,-2.7221445396627,
-2.71340473293917,-2.70661000614579,-2.70166558365389,-2.69341637264005,
-2.66929546992004,-2.65205014777285,-2.6431216788472,-2.63409010065303,
-2.63384867082664),.UNSPECIFIED.);
#23512=B_SPLINE_CURVE_WITH_KNOTS('',3,(#131998,#131999,#132000,#132001,
#132002,#132003,#132004,#132005,#132006,#132007,#132008,#132009,#132010,
#132011,#132012,#132013,#132014,#132015,#132016,#132017,#132018,#132019,
#132020,#132021,#132022,#132023,#132024,#132025,#132026,#132027,#132028,
#132029,#132030,#132031,#132032,#132033,#132034,#132035,#132036,#132037,
#132038,#132039,#132040,#132041,#132042,#132043,#132044,#132045,#132046,
#132047,#132048,#132049,#132050,#132051,#132052,#132053,#132054,#132055,
#132056,#132057,#132058,#132059,#132060,#132061,#132062,#132063,#132064,
#132065,#132066,#132067),.UNSPECIFIED.,.F.,.F.,(4,3,3,3,3,3,3,3,3,3,3,3,
3,3,3,3,3,3,3,3,3,3,3,4),(18.2318968787514,18.3499060448615,18.4254225216423,
18.4254628817511,18.5349017943127,18.5466830322889,18.6645202762246,18.7822476823724,
18.8999144714775,19.0237418751216,19.1415119471466,19.2593533686491,19.3681535768292,
19.3773895303943,19.3951836545557,19.3952240860538,19.5034482068642,19.5116532354367,
19.6279187208041,19.7440727823547,19.8602106139534,19.9763358926106,20.0925766625481,
20.1591190620686),.UNSPECIFIED.);
#23513=B_SPLINE_CURVE_WITH_KNOTS('',3,(#132068,#132069,#132070,#132071,
#132072,#132073,#132074,#132075,#132076,#132077,#132078,#132079,#132080,
#132081,#132082,#132083,#132084,#132085,#132086,#132087,#132088,#132089,
#132090,#132091,#132092,#132093,#132094,#132095,#132096,#132097,#132098,
#132099,#132100,#132101,#132102,#132103,#132104,#132105,#132106,#132107,
#132108,#132109,#132110,#132111,#132112,#132113,#132114,#132115,#132116,
#132117,#132118,#132119,#132120,#132121,#132122,#132123,#132124,#132125,
#132126,#132127,#132128,#132129,#132130,#132131,#132132,#132133,#132134,
#132135,#132136,#132137,#132138,#132139,#132140,#132141,#132142,#132143,
#132144,#132145,#132146,#132147,#132148,#132149,#132150,#132151,#132152,
#132153,#132154,#132155,#132156,#132157,#132158,#132159,#132160,#132161,
#132162,#132163,#132164,#132165,#132166,#132167,#132168,#132169,#132170,
#132171,#132172,#132173,#132174,#132175,#132176,#132177,#132178,#132179,
#132180,#132181,#132182,#132183,#132184,#132185,#132186,#132187,#132188,
#132189,#132190,#132191,#132192,#132193,#132194,#132195,#132196,#132197,
#132198,#132199,#132200,#132201,#132202,#132203,#132204,#132205,#132206,
#132207,#132208,#132209,#132210,#132211,#132212,#132213,#132214,#132215,
#132216,#132217,#132218,#132219,#132220,#132221,#132222,#132223,#132224,
#132225,#132226,#132227,#132228,#132229,#132230,#132231,#132232,#132233,
#132234,#132235,#132236),.UNSPECIFIED.,.F.,.F.,(4,3,3,3,3,3,3,3,3,3,3,3,
3,3,3,3,3,3,3,3,3,3,3,3,3,3,3,3,3,3,3,3,3,3,3,3,3,3,3,3,3,3,3,3,3,3,3,3,
3,3,3,3,3,3,3,3,4),(20.1591190625159,20.2764390510706,20.3187721935057,
20.3649448970694,20.3649852903564,20.474417801013,20.4862054408942,20.6040549230358,
20.7217944086693,20.8394730948977,20.963291444838,21.0810728019401,21.1989252820012,
21.3077531878469,21.3169720970495,21.3347063100803,21.3347464946591,21.4442282833429,
21.4559666451969,21.5738205697139,21.6915648498455,21.8092486681115,21.9330634258241,
22.0508506746636,22.1687092972027,22.2774757196079,22.286762555749,22.3044668739246,
22.3045076989618,22.4138253643461,22.4257278494996,22.5434476083366,22.6610576036881,
22.7786073001942,22.8961460614269,23.0137987630076,23.1315213911073,23.2408817617996,
23.2494427315033,23.2742286871683,23.2742689032645,23.3837601059622,23.3954890538023,
23.5135004049658,23.6314007909792,23.7492390721056,23.872936830971,23.9908723543834,
24.1088768964893,24.2178723756311,24.227071612826,24.243991132142,24.2440301075672,
24.3536763359503,24.36212772944,24.4800381950529,24.5160781357833),
 .UNSPECIFIED.);
#23514=B_SPLINE_CURVE_WITH_KNOTS('',3,(#132237,#132238,#132239,#132240,
#132241,#132242,#132243,#132244,#132245,#132246,#132247,#132248,#132249,
#132250,#132251,#132252,#132253,#132254,#132255,#132256,#132257,#132258,
#132259,#132260,#132261,#132262,#132263,#132264,#132265,#132266,#132267,
#132268,#132269,#132270,#132271,#132272,#132273,#132274,#132275,#132276,
#132277,#132278,#132279,#132280,#132281,#132282,#132283,#132284,#132285,
#132286,#132287,#132288,#132289,#132290,#132291,#132292,#132293,#132294,
#132295,#132296,#132297,#132298,#132299,#132300,#132301,#132302,#132303,
#132304,#132305,#132306,#132307,#132308,#132309,#132310,#132311,#132312,
#132313,#132314,#132315,#132316,#132317,#132318,#132319,#132320,#132321,
#132322,#132323,#132324,#132325,#132326,#132327,#132328,#132329,#132330,
#132331,#132332,#132333,#132334,#132335,#132336,#132337,#132338,#132339,
#132340,#132341,#132342,#132343,#132344,#132345,#132346,#132347,#132348,
#132349,#132350,#132351,#132352,#132353,#132354,#132355,#132356,#132357,
#132358,#132359,#132360,#132361,#132362,#132363,#132364),.UNSPECIFIED.,
 .F.,.F.,(4,2,2,2,2,2,2,2,2,2,2,2,2,2,2,2,2,2,2,2,2,2,2,2,2,2,2,2,2,2,2,
2,2,2,2,2,2,2,2,2,2,2,2,2,2,2,2,2,2,2,2,2,2,2,2,2,2,2,2,2,2,2,2,4),(-2.63384867082664,
-2.60067956115208,-2.59119414892037,-2.58402991229563,-2.57912411549598,
-2.57146069037577,-2.5473132317638,-2.53466143758753,-2.52403834163957,
-2.5155862270938,-2.50422460492688,-2.4778500674872,-2.46829890759395,-2.4611038002552,
-2.45619820385995,-2.44856786564464,-2.42444097166765,-2.41174747505461,
-2.40110117074743,-2.39264221378778,-2.38128293886777,-2.35344473355548,
-2.34099561201416,-2.33564330964062,-2.33002410084309,-2.31728322222918,
-2.29564491923898,-2.28528930652753,-2.27584719821023,-2.26727488092526,
-2.25321574587793,-2.22951661748433,-2.22117593417236,-2.21458911856265,
-2.20962903418765,-2.20107179807238,-2.17709296678601,-2.16011550663879,
-2.1512076056052,-2.14215607868278,-2.12531024847009,-2.1054024507707,-2.09455795636171,
-2.08936637732718,-2.08350642644974,-2.05509108134002,-2.04263269994247,
-2.03210378346703,-2.02364244755537,-2.01213803513009,-1.98581119979471,
-1.97640028808093,-1.9692728629665,-1.96436386244352,-1.95664639724681,
-1.93246646956722,-1.91455841226969,-1.905585369101,-1.89660593350099,-1.86360397177841,
-1.85380258767236,-1.84648679371643,-1.84158243035126,-1.83725267846888),
 .UNSPECIFIED.);
#23515=B_SPLINE_CURVE_WITH_KNOTS('',3,(#132370,#132371,#132372,#132373,
#132374,#132375,#132376,#132377,#132378,#132379,#132380,#132381,#132382,
#132383,#132384,#132385,#132386,#132387,#132388,#132389,#132390,#132391,
#132392,#132393,#132394,#132395,#132396,#132397,#132398,#132399,#132400,
#132401,#132402,#132403,#132404,#132405,#132406,#132407,#132408,#132409,
#132410,#132411,#132412,#132413,#132414,#132415,#132416,#132417,#132418,
#132419,#132420,#132421,#132422,#132423,#132424,#132425,#132426,#132427,
#132428,#132429,#132430,#132431,#132432,#132433,#132434,#132435,#132436,
#132437,#132438,#132439,#132440,#132441,#132442),.UNSPECIFIED.,.F.,.F.,
(4,3,3,3,3,3,3,3,3,3,3,3,3,3,3,3,3,3,3,3,3,3,3,3,4),(11.9496359932348,12.0673160274323,
12.1849660908497,12.3027153329077,12.4205170320056,12.5385275150523,12.6068552689481,
12.6068956559349,12.716327864626,12.7281158064727,12.8459491614091,12.9636726570828,
13.0813355227604,13.2051658571297,13.322932027576,13.4407695608851,13.5495730494168,
13.5588018842955,13.5766164730029,13.5766568602376,13.6924275909584,13.7171311431147,
13.8384365563071,13.8560591145712,13.8759337548442),.UNSPECIFIED.);
#23516=B_SPLINE_CURVE_WITH_KNOTS('',3,(#132443,#132444,#132445,#132446,
#132447,#132448,#132449,#132450,#132451,#132452,#132453,#132454,#132455,
#132456,#132457,#132458,#132459,#132460,#132461,#132462,#132463,#132464,
#132465,#132466,#132467,#132468,#132469,#132470,#132471,#132472,#132473,
#132474,#132475,#132476,#132477,#132478,#132479,#132480,#132481,#132482,
#132483,#132484,#132485,#132486,#132487,#132488,#132489,#132490,#132491,
#132492,#132493,#132494,#132495,#132496,#132497,#132498,#132499,#132500,
#132501,#132502,#132503,#132504,#132505,#132506,#132507,#132508,#132509,
#132510,#132511,#132512,#132513,#132514,#132515,#132516,#132517,#132518,
#132519,#132520,#132521,#132522,#132523,#132524,#132525,#132526,#132527,
#132528,#132529,#132530,#132531,#132532,#132533,#132534,#132535,#132536,
#132537,#132538,#132539,#132540,#132541,#132542,#132543,#132544,#132545,
#132546,#132547,#132548,#132549,#132550,#132551,#132552,#132553,#132554,
#132555,#132556,#132557,#132558,#132559,#132560,#132561,#132562,#132563,
#132564,#132565,#132566,#132567,#132568,#132569,#132570,#132571,#132572,
#132573,#132574,#132575,#132576,#132577,#132578,#132579,#132580,#132581,
#132582,#132583,#132584,#132585,#132586,#132587,#132588,#132589,#132590,
#132591,#132592,#132593,#132594,#132595,#132596),.UNSPECIFIED.,.F.,.F.,
(4,3,3,3,3,3,3,3,3,3,3,3,3,3,3,3,3,3,3,3,3,3,3,3,3,3,3,3,3,3,3,3,3,3,3,
3,3,3,3,3,3,3,3,3,3,3,3,3,3,3,3,4),(13.8759337553363,13.9931001931372,14.1102297432661,
14.227456018611,14.3447302301731,14.4622230557154,14.5463776774895,14.5464180645403,
14.6558502199931,14.6676382150781,14.7854717014034,14.9031953293054,15.0208583277855,
15.1446885630499,15.2624548660176,15.3802925315736,15.4890963596955,15.4983249858325,
15.5161388853966,15.516179268843,15.6256123789708,15.6373994193808,15.7552334287766,
15.8729575826182,15.9906211087535,16.1144509498516,16.2322177774323,16.350055965759,
16.4588592445964,16.468088936011,16.4859000823221,16.4859404731457,16.5953716256398,
16.6071606236835,16.72499248228,16.8427144891674,16.9603758766909,17.0842073268803,
17.201972065724,17.3198081855426,17.4286108793835,17.4378391321563,17.4556612869848,
17.4557016774484,17.5649968511712,17.5737108704674,17.691552459125,17.809275867409,
17.9269654738832,18.0446320340746,18.1623925830577,18.2318968781416),
 .UNSPECIFIED.);
#23517=B_SPLINE_CURVE_WITH_KNOTS('',3,(#132597,#132598,#132599,#132600,
#132601,#132602,#132603,#132604,#132605,#132606,#132607,#132608,#132609,
#132610,#132611,#132612,#132613,#132614,#132615,#132616,#132617,#132618,
#132619,#132620,#132621,#132622,#132623,#132624,#132625,#132626,#132627,
#132628,#132629,#132630,#132631,#132632,#132633,#132634,#132635,#132636,
#132637,#132638,#132639,#132640,#132641,#132642,#132643,#132644,#132645,
#132646,#132647,#132648,#132649,#132650,#132651,#132652,#132653,#132654,
#132655,#132656,#132657,#132658,#132659,#132660,#132661,#132662,#132663,
#132664,#132665,#132666,#132667,#132668,#132669,#132670,#132671,#132672,
#132673,#132674,#132675,#132676,#132677,#132678,#132679,#132680,#132681,
#132682,#132683,#132684,#132685,#132686,#132687,#132688,#132689,#132690,
#132691,#132692,#132693,#132694,#132695,#132696,#132697,#132698,#132699,
#132700,#132701,#132702,#132703,#132704,#132705,#132706,#132707,#132708,
#132709,#132710,#132711,#132712,#132713,#132714,#132715,#132716,#132717,
#132718,#132719,#132720,#132721,#132722),.UNSPECIFIED.,.F.,.F.,(4,2,2,2,
2,2,2,2,2,2,2,2,2,2,2,2,2,2,2,2,2,2,2,2,2,2,2,2,2,2,2,2,2,2,2,2,2,2,2,2,
2,2,2,2,2,2,2,2,2,2,2,2,2,2,2,2,2,2,2,2,2,2,4),(-1.83725267846888,-1.83540027261704,
-1.80649375697848,-1.7907382655999,-1.78192911062747,-1.77274762825419,
-1.75171025246169,-1.72954720864117,-1.72288070231471,-1.71793252782111,
-1.70952556097505,-1.68548227945112,-1.67335330776921,-1.66298902805841,
-1.65451607444484,-1.64276697738429,-1.61561732441011,-1.60328339766176,
-1.5979428133892,-1.59231277798626,-1.57562459927013,-1.54653158396036,
-1.53736727038257,-1.52854686968659,-1.51265221693632,-1.4832057820726,
-1.47673981772376,-1.47175743220665,-1.46294422715869,-1.44962073482292,
-1.42498282195484,-1.41544140299866,-1.4068077330654,-1.39301630384327,
-1.3723064328929,-1.35832268342317,-1.3526594265846,-1.34734360822437,-1.33527350157431,
-1.30963880664845,-1.29693930152237,-1.28840114107177,-1.27851407155737,
-1.26731537638929,-1.23958430815731,-1.23198506747337,-1.22707912560906,
-1.21985226203874,-1.21023587080884,-1.18383288203522,-1.17252500208232,
-1.16406968181561,-1.15338946439338,-1.14062577328499,-1.11656054394905,
-1.10900138834538,-1.10409489772297,-1.09682586225881,-1.08712210264066,
-1.06070683511646,-1.0494855520871,-1.04103037475671,-1.04064001717697),
 .UNSPECIFIED.);
#23518=B_SPLINE_CURVE_WITH_KNOTS('',3,(#132728,#132729,#132730,#132731,
#132732,#132733,#132734,#132735,#132736,#132737,#132738,#132739,#132740,
#132741,#132742,#132743,#132744,#132745,#132746,#132747,#132748,#132749,
#132750,#132751,#132752,#132753,#132754,#132755,#132756,#132757,#132758,
#132759,#132760,#132761,#132762,#132763,#132764,#132765,#132766,#132767),
 .UNSPECIFIED.,.F.,.F.,(4,2,2,2,2,2,2,2,2,2,2,2,2,2,2,2,2,2,2,4),(-0.244113824073537,
-0.239274607958611,-0.232075560584042,-0.215284623761484,-0.193721270389367,
-0.184734703888983,-0.176413733489245,-0.162966360303477,-0.142799703874305,
-0.128605522576123,-0.123032716585563,-0.117806633684679,-0.106999069803744,
-0.088067278378308,-0.0671333114716234,-0.0571684315808229,-0.0472634875266598,
-0.0365466086441564,-0.00613189374829842,-9.999999997512E-7),
 .UNSPECIFIED.);
#23519=B_SPLINE_CURVE_WITH_KNOTS('',3,(#132770,#132771,#132772,#132773,
#132774,#132775,#132776,#132777,#132778,#132779,#132780,#132781,#132782,
#132783,#132784,#132785,#132786,#132787,#132788,#132789,#132790,#132791,
#132792,#132793,#132794,#132795,#132796,#132797,#132798,#132799,#132800,
#132801,#132802,#132803,#132804,#132805,#132806,#132807,#132808,#132809,
#132810,#132811,#132812,#132813,#132814,#132815,#132816,#132817,#132818,
#132819,#132820,#132821,#132822,#132823,#132824,#132825,#132826,#132827,
#132828,#132829,#132830,#132831,#132832,#132833,#132834,#132835,#132836,
#132837,#132838,#132839,#132840,#132841,#132842,#132843,#132844,#132845,
#132846,#132847,#132848,#132849,#132850,#132851,#132852,#132853,#132854,
#132855,#132856,#132857,#132858,#132859,#132860,#132861,#132862,#132863,
#132864,#132865,#132866,#132867,#132868,#132869,#132870,#132871,#132872,
#132873,#132874,#132875,#132876,#132877,#132878,#132879,#132880,#132881,
#132882,#132883,#132884,#132885,#132886,#132887,#132888,#132889,#132890,
#132891,#132892,#132893),.UNSPECIFIED.,.F.,.F.,(4,3,3,3,3,3,3,3,3,3,3,3,
3,3,3,3,3,3,3,3,3,3,3,3,3,3,3,3,3,3,3,3,3,3,3,3,3,3,3,3,3,4),(2.02979616106461,
2.13731278964836,2.25387952414295,2.37034808538608,2.48676999582052,2.60327394271786,
2.7198198649459,2.83656862171718,2.90924455446903,2.90928361290806,3.01897333379382,
3.0305037634459,3.14850457265912,3.26639864796982,3.38423483867336,3.50793733330771,
3.62588130590733,3.74389791908222,3.85268065170137,3.86210971336039,3.87900456259159,
3.87904481721075,3.98841302401164,4.00026496774859,4.1179884109348,4.23560061539567,
4.3531510496196,4.47068907909621,4.58833890332437,4.70605739173758,4.81536506782819,
4.82397281846676,4.84876523864822,4.84880602151344,4.95807677792782,4.96683189172654,
5.0846917355895,5.20243492684846,5.32015599904385,5.43785457553909,5.55567683153886,
5.66555025291942),.UNSPECIFIED.);
#23520=B_SPLINE_CURVE_WITH_KNOTS('',3,(#132899,#132900,#132901,#132902,
#132903,#132904,#132905,#132906,#132907,#132908,#132909,#132910,#132911,
#132912,#132913,#132914,#132915,#132916,#132917,#132918,#132919,#132920,
#132921,#132922,#132923,#132924,#132925,#132926,#132927,#132928,#132929,
#132930,#132931,#132932,#132933,#132934,#132935,#132936,#132937,#132938,
#132939,#132940,#132941,#132942,#132943,#132944,#132945,#132946,#132947,
#132948,#132949,#132950),.UNSPECIFIED.,.F.,.F.,(4,2,2,2,2,2,2,2,2,2,2,2,
2,2,2,2,2,2,2,2,2,2,2,2,2,4),(0.344554558968716,0.344695447752049,0.370408719319506,
0.382229545579032,0.387689649352779,0.39262279171678,0.401708900904157,
0.414890311351945,0.450541662365071,0.460731339588076,0.468816672676823,
0.47883136281416,0.501888851608725,0.531468925320272,0.537561368006789,
0.542411001121594,0.549967383213274,0.559703908103843,0.587319345975018,
0.607371005886695,0.617729857954321,0.627231554499862,0.642213057001694,
0.678980954192163,0.68447448160504,0.688655615358866),.UNSPECIFIED.);
#23521=B_SPLINE_CURVE_WITH_KNOTS('',3,(#132953,#132954,#132955,#132956,
#132957,#132958,#132959,#132960,#132961,#132962,#132963,#132964,#132965,
#132966,#132967,#132968,#132969,#132970,#132971,#132972,#132973,#132974,
#132975,#132976,#132977,#132978,#132979,#132980,#132981,#132982,#132983,
#132984,#132985,#132986,#132987,#132988,#132989,#132990,#132991,#132992,
#132993,#132994,#132995,#132996,#132997,#132998,#132999,#133000,#133001,
#133002,#133003,#133004,#133005,#133006,#133007,#133008,#133009,#133010),
 .UNSPECIFIED.,.F.,.F.,(4,2,2,2,2,2,2,2,2,2,2,2,2,2,2,2,2,2,2,2,2,2,2,2,
2,2,2,2,4),(0.00011252101050449,0.041699780384492,0.0557287632500945,0.0645534172788003,
0.0737635674151307,0.091079388371737,0.11795996984337,0.12736070271703,
0.134692008622996,0.13962170386702,0.14639769538055,0.168035682739452,0.196617660235601,
0.207522562098428,0.215900590072862,0.226230086770072,0.247670796581079,
0.276081175629665,0.28396280928484,0.28886530845821,0.295003459806395,0.311857396532249,
0.336823282175015,0.352803198578938,0.36176534231516,0.370488610565894,
0.384591414707687,0.404098492780895,0.424937847293283),.UNSPECIFIED.);
#23522=B_SPLINE_CURVE_WITH_KNOTS('',3,(#133016,#133017,#133018,#133019,
#133020,#133021,#133022,#133023,#133024,#133025,#133026,#133027,#133028,
#133029,#133030,#133031,#133032,#133033,#133034,#133035,#133036,#133037,
#133038,#133039,#133040,#133041,#133042,#133043,#133044,#133045,#133046,
#133047,#133048,#133049,#133050,#133051,#133052,#133053,#133054,#133055,
#133056,#133057,#133058,#133059,#133060,#133061,#133062,#133063,#133064,
#133065,#133066,#133067,#133068,#133069,#133070,#133071,#133072,#133073,
#133074,#133075,#133076,#133077,#133078,#133079,#133080,#133081,#133082,
#133083,#133084,#133085,#133086,#133087,#133088,#133089,#133090,#133091,
#133092,#133093,#133094,#133095,#133096,#133097,#133098,#133099,#133100,
#133101,#133102,#133103),.UNSPECIFIED.,.F.,.F.,(4,2,2,2,2,2,2,2,2,2,2,2,
2,2,2,2,2,2,2,2,2,2,2,2,2,2,2,2,2,2,2,2,2,2,2,2,2,2,2,2,2,2,2,4),(0.344313126688005,
0.354918123843971,0.374366698299649,0.383748143804426,0.392345335212504,
0.405089284051333,0.43908719147313,0.44932272354443,0.457074657025849,0.461929493923398,
0.468150394212971,0.485829073431582,0.521852174852332,0.531959348747117,
0.54039981992874,0.551557879687373,0.564757640353234,0.601877414689068,
0.608288344649744,0.613149924500441,0.620466415978113,0.62986210726005,
0.656605319920672,0.67473191285089,0.683983704285279,0.692636320584211,
0.705836061138201,0.738781598773739,0.752533255556161,0.758702667603722,
0.763630337873969,0.77159418253717,0.782246926162731,0.820662279048881,
0.831090532659605,0.839537414282043,0.850354499700508,0.862914796418882,
0.894352883679797,0.904852002876094,0.910126945759735,0.91548779764376,
0.926695144009761,0.971534887947364),.UNSPECIFIED.);
#23523=B_SPLINE_CURVE_WITH_KNOTS('',3,(#133104,#133105,#133106,#133107,
#133108,#133109,#133110,#133111,#133112,#133113,#133114,#133115,#133116,
#133117,#133118,#133119,#133120,#133121,#133122,#133123,#133124,#133125,
#133126,#133127,#133128,#133129,#133130,#133131,#133132,#133133,#133134,
#133135,#133136,#133137,#133138,#133139,#133140,#133141,#133142,#133143,
#133144,#133145,#133146,#133147,#133148,#133149,#133150,#133151,#133152,
#133153,#133154,#133155,#133156,#133157),.UNSPECIFIED.,.F.,.F.,(4,2,2,2,
2,2,2,2,2,2,2,2,2,2,2,2,2,2,2,2,2,2,2,2,2,2,4),(0.000524566479899316,0.0077941571992236,
0.0151826284352965,0.0243122873221318,0.0406590091156156,0.0706586396051979,
0.0795091358994713,0.0865255523349244,0.0913709499927136,0.0981326219554219,
0.120805284763708,0.141285174801549,0.155804101380645,0.164653423760952,
0.173690646419438,0.189720230658505,0.218883157209673,0.228605882077984,
0.236105313658492,0.241047335047455,0.247603430811587,0.277711278906036,
0.293614276409027,0.306144255402436,0.314795925305086,0.324451976165178,
0.344554558968716),.UNSPECIFIED.);
#23524=B_SPLINE_CURVE_WITH_KNOTS('',3,(#133159,#133160,#133161,#133162,
#133163,#133164,#133165,#133166,#133167,#133168,#133169,#133170,#133171,
#133172,#133173,#133174,#133175,#133176,#133177,#133178,#133179,#133180,
#133181,#133182,#133183,#133184,#133185,#133186,#133187,#133188,#133189,
#133190,#133191,#133192,#133193,#133194,#133195,#133196,#133197,#133198,
#133199,#133200,#133201,#133202,#133203,#133204,#133205,#133206,#133207,
#133208,#133209,#133210,#133211,#133212,#133213,#133214,#133215,#133216),
 .UNSPECIFIED.,.F.,.F.,(4,2,2,2,2,2,2,2,2,2,2,2,2,2,2,2,2,2,2,2,2,2,2,2,
2,2,2,2,4),(0.424937847293283,0.428436000227204,0.435138620818605,0.43996872558882,
0.446986518277264,0.455831102636226,0.47890579835249,0.500189470027702,
0.509890346462041,0.518397659520366,0.530311411427524,0.544957168344203,
0.570901333375234,0.581808427089302,0.587145609789906,0.592482767170828,
0.603425566592698,0.621365986001914,0.647390935126662,0.657912395158918,
0.666329996071405,0.676963193949592,0.689209727077069,0.718398075004121,
0.730491079418018,0.736216066718949,0.74125824996203,0.750232951729319,
0.768709662504308),.UNSPECIFIED.);
#23525=B_SPLINE_CURVE_WITH_KNOTS('',3,(#133217,#133218,#133219,#133220,
#133221,#133222,#133223,#133224,#133225,#133226,#133227,#133228,#133229,
#133230,#133231,#133232,#133233,#133234,#133235,#133236,#133237,#133238,
#133239,#133240,#133241,#133242,#133243,#133244,#133245,#133246,#133247,
#133248,#133249,#133250,#133251,#133252,#133253,#133254,#133255,#133256,
#133257,#133258,#133259,#133260,#133261,#133262,#133263,#133264,#133265,
#133266,#133267,#133268,#133269,#133270,#133271,#133272,#133273,#133274,
#133275,#133276,#133277,#133278,#133279,#133280,#133281,#133282,#133283,
#133284,#133285,#133286,#133287,#133288,#133289,#133290,#133291,#133292,
#133293,#133294,#133295,#133296,#133297,#133298,#133299,#133300,#133301,
#133302,#133303,#133304),.UNSPECIFIED.,.F.,.F.,(4,2,2,2,2,2,2,2,2,2,2,2,
2,2,2,2,2,2,2,2,2,2,2,2,2,2,2,2,2,2,2,2,2,2,2,2,2,2,2,2,2,2,2,4),(0.000419544874521375,
0.0233932134995514,0.0364089109472125,0.045024068885147,0.0542931007919817,
0.0727142211952471,0.0991310565398044,0.108478695324941,0.11576629488603,
0.120620066616287,0.127033193154977,0.154085931685306,0.172261793514291,
0.185823684729299,0.194512570147632,0.203658292275543,0.220896432485435,
0.248636272349738,0.258162051746496,0.265544985518916,0.270406918789259,
0.276760764395479,0.313958603043289,0.332675935597904,0.341976982539643,
0.350487698338711,0.363314427355328,0.395002516451318,0.40635216444106,
0.414650374305314,0.419602519578251,0.425571305817675,0.441130025493829,
0.473089485352324,0.486094575418098,0.494625666168507,0.503874867646591,
0.522087704793587,0.556582967638413,0.564691773798812,0.569620959574018,
0.575673323302464,0.594016680923033,0.627725856927242),.UNSPECIFIED.);
#23526=B_SPLINE_CURVE_WITH_KNOTS('',3,(#133310,#133311,#133312,#133313,
#133314,#133315,#133316,#133317,#133318,#133319,#133320,#133321,#133322,
#133323,#133324,#133325,#133326,#133327,#133328,#133329,#133330,#133331,
#133332,#133333,#133334,#133335,#133336,#133337,#133338,#133339,#133340,
#133341,#133342,#133343,#133344,#133345,#133346,#133347,#133348,#133349,
#133350,#133351,#133352,#133353,#133354,#133355,#133356,#133357,#133358,
#133359,#133360,#133361,#133362,#133363,#133364,#133365,#133366,#133367,
#133368,#133369,#133370,#133371,#133372,#133373,#133374,#133375,#133376,
#133377,#133378,#133379,#133380,#133381,#133382,#133383,#133384,#133385,
#133386,#133387,#133388,#133389,#133390,#133391,#133392,#133393,#133394,
#133395,#133396,#133397,#133398,#133399,#133400,#133401,#133402,#133403,
#133404,#133405,#133406,#133407,#133408,#133409,#133410,#133411,#133412,
#133413,#133414,#133415,#133416,#133417,#133418,#133419,#133420,#133421,
#133422,#133423,#133424,#133425,#133426,#133427,#133428,#133429,#133430,
#133431,#133432,#133433,#133434,#133435,#133436,#133437,#133438,#133439,
#133440,#133441,#133442,#133443,#133444,#133445,#133446,#133447,#133448,
#133449,#133450,#133451,#133452,#133453,#133454),.UNSPECIFIED.,.F.,.F.,
(4,3,3,3,3,3,3,3,3,3,3,3,3,3,3,3,3,3,3,3,3,3,3,3,3,3,3,3,3,3,3,3,3,3,3,
3,3,3,3,3,3,3,3,3,3,3,3,3,4),(24.2160877562439,24.3282107851649,24.433568916188,
24.4405143049486,24.4622569195143,24.4622900504513,24.5642705178838,24.5745672323181,
24.6866901662804,24.7987091946534,24.9106667311218,25.0226050998941,25.134641377221,
25.2467284172589,25.3590102867046,25.432018123817,25.4320512548983,25.534031744494,
25.5443284200344,25.6564513436384,25.7684703654884,25.8804278992591,25.9923662691535,
26.104402553425,26.2164896036862,26.3287714884588,26.4017793281197,26.401812458991,
26.5037928807345,26.5140897641856,26.6262128229447,26.7382319769481,26.8501896396517,
26.9621281350364,27.074164538597,27.1862517048167,27.2985336989236,27.3715405324224,
27.3715736606472,27.4729397858348,27.4843897011581,27.5954688646583,27.7064470869093,
27.8173685700046,27.9316098980805,28.0426142213783,28.1584740518432,28.2669736810215,
28.2743338823082),.UNSPECIFIED.);
#23527=B_SPLINE_CURVE_WITH_KNOTS('',3,(#133455,#133456,#133457,#133458,
#133459,#133460,#133461,#133462,#133463,#133464,#133465,#133466,#133467,
#133468,#133469,#133470,#133471,#133472,#133473,#133474,#133475,#133476,
#133477,#133478,#133479,#133480,#133481,#133482,#133483,#133484,#133485,
#133486,#133487,#133488,#133489,#133490,#133491,#133492,#133493,#133494,
#133495,#133496,#133497,#133498,#133499,#133500,#133501,#133502,#133503,
#133504,#133505,#133506,#133507,#133508),.UNSPECIFIED.,.F.,.F.,(4,2,2,2,
2,2,2,2,2,2,2,2,2,2,2,2,2,2,2,2,2,2,2,2,2,2,4),(0.000401295307783161,0.00458155931597832,
0.00839099750411614,0.0129621842065248,0.0197180999475689,0.0416315109177654,
0.0701737326177952,0.0810165741531973,0.0894483718434477,0.0998096768753931,
0.122012873596538,0.14963882305013,0.157349664678133,0.162242769337582,
0.168520511947801,0.201417066394714,0.216783128127933,0.229060063100129,
0.237602488290952,0.247142420184493,0.26607663779579,0.295650400186901,
0.305631985080099,0.310829084887432,0.316325587180611,0.328401515947946,
0.344313126688005),.UNSPECIFIED.);
#23528=B_SPLINE_CURVE_WITH_KNOTS('',3,(#133510,#133511,#133512,#133513,
#133514,#133515,#133516,#133517,#133518,#133519,#133520,#133521,#133522,
#133523,#133524,#133525,#133526,#133527,#133528,#133529,#133530,#133531,
#133532,#133533,#133534,#133535,#133536,#133537,#133538,#133539,#133540,
#133541,#133542,#133543,#133544,#133545,#133546,#133547,#133548,#133549,
#133550,#133551,#133552,#133553,#133554,#133555,#133556,#133557,#133558,
#133559,#133560,#133561,#133562,#133563,#133564,#133565),.UNSPECIFIED.,
 .F.,.F.,(4,2,2,2,2,2,2,2,2,2,2,2,2,2,2,2,2,2,2,2,2,2,2,2,2,2,2,4),(0.627725856927242,
0.629596283308658,0.63975508292202,0.648183324876226,0.659243417114572,
0.672267110924607,0.707923783258628,0.715270239128067,0.720128254355387,
0.726620854841594,0.734528358704402,0.752578944641735,0.778447337204221,
0.788968913601055,0.797384035844684,0.808010516682078,0.820247867992551,
0.849396806529477,0.861503718464746,0.867231013069058,0.872275104599302,
0.881253555536561,0.894085492808777,0.929024211645749,0.939294873057738,
0.947636430899488,0.955772098337237,0.971766832159165),.UNSPECIFIED.);
#23529=B_SPLINE_CURVE_WITH_KNOTS('',3,(#133566,#133567,#133568,#133569,
#133570,#133571,#133572,#133573,#133574,#133575,#133576,#133577,#133578,
#133579,#133580,#133581,#133582,#133583,#133584,#133585,#133586,#133587,
#133588,#133589,#133590,#133591,#133592,#133593,#133594,#133595,#133596,
#133597,#133598,#133599,#133600,#133601,#133602,#133603,#133604,#133605,
#133606,#133607,#133608,#133609,#133610,#133611,#133612,#133613,#133614,
#133615,#133616,#133617,#133618,#133619,#133620,#133621,#133622,#133623,
#133624,#133625,#133626,#133627,#133628,#133629,#133630,#133631,#133632,
#133633,#133634,#133635,#133636,#133637,#133638,#133639,#133640,#133641,
#133642,#133643,#133644,#133645,#133646,#133647,#133648,#133649,#133650,
#133651,#133652,#133653,#133654,#133655,#133656,#133657),.UNSPECIFIED.,
 .F.,.F.,(4,2,2,2,2,2,2,2,2,2,2,2,2,2,2,2,2,2,2,2,2,2,2,2,2,2,2,2,2,2,2,
2,2,2,2,2,2,2,2,2,2,2,2,2,2,4),(1.73404294796756E-6,0.020495970861449,0.0330996216089653,
0.0419769718929025,0.0470070872550434,0.0527666339134735,0.0650876584115866,
0.0904623397779247,0.110007353955857,0.119387901293855,0.127964585074818,
0.140630912374979,0.174747727887424,0.184991269521981,0.192745046791807,
0.197595130754773,0.203800086830298,0.237149346034272,0.252367379953921,
0.26456711247523,0.273090986304503,0.282637514331492,0.302760301073997,
0.327070486930191,0.33981886423407,0.345394133876651,0.350521619915592,
0.360068857625006,0.392612595549552,0.405291587671783,0.416164293246166,
0.424507136403704,0.434770583644445,0.469617551530864,0.48253403595284,
0.491549675797676,0.496599330746143,0.502315871090777,0.514353726955077,
0.543561663310129,0.555805376093377,0.566436169494636,0.574851582309342,
0.585369517699426,0.610556750243185,0.627052488170293),.UNSPECIFIED.);
#23530=B_SPLINE_CURVE_WITH_KNOTS('',3,(#133663,#133664,#133665,#133666,
#133667,#133668,#133669,#133670,#133671,#133672,#133673,#133674,#133675,
#133676,#133677,#133678,#133679,#133680,#133681,#133682,#133683,#133684,
#133685,#133686,#133687,#133688,#133689,#133690,#133691,#133692,#133693,
#133694,#133695,#133696,#133697,#133698,#133699,#133700,#133701,#133702,
#133703,#133704,#133705,#133706,#133707,#133708,#133709,#133710,#133711,
#133712,#133713,#133714,#133715,#133716),.UNSPECIFIED.,.F.,.F.,(4,2,2,2,
2,2,2,2,2,2,2,2,2,2,2,2,2,2,2,2,2,2,2,2,2,2,4),(1.59817392798203,1.60932378016397,
1.61869868697383,1.62733365173653,1.64023726404545,1.67162575265904,1.68787810507124,
1.69389407117143,1.69895843539788,1.70764196400482,1.71979547470253,1.75709173714892,
1.76672103445419,1.77536478897417,1.78788251698795,1.80364999662174,1.83572560451703,
1.84214503875942,1.84685370433738,1.85369583926341,1.86232249408446,1.88440038256527,
1.90842251392954,1.91795674849125,1.92605688782117,1.93359256393498,1.94232018637391),
 .UNSPECIFIED.);
#23531=B_SPLINE_CURVE_WITH_KNOTS('',3,(#133718,#133719,#133720,#133721,
#133722,#133723,#133724,#133725,#133726,#133727,#133728,#133729,#133730,
#133731,#133732,#133733,#133734,#133735,#133736,#133737,#133738,#133739,
#133740,#133741,#133742,#133743,#133744,#133745,#133746,#133747,#133748,
#133749,#133750,#133751,#133752,#133753,#133754),.UNSPECIFIED.,.F.,.F.,
(4,3,3,3,3,3,3,3,3,3,3,3,4),(14.3984001269719,14.5130169718746,14.6275760065012,
14.7421062972226,14.8566423616352,14.9712187150792,15.0859565871695,15.2007827297925,
15.3158271617794,15.3681613312745,15.4944256857545,15.6197345261748,15.7079562980946),
 .UNSPECIFIED.);
#23532=B_SPLINE_CURVE_WITH_KNOTS('',3,(#133757,#133758,#133759,#133760,
#133761,#133762,#133763,#133764,#133765,#133766,#133767,#133768,#133769,
#133770,#133771,#133772,#133773,#133774,#133775,#133776,#133777,#133778,
#133779,#133780,#133781,#133782,#133783,#133784,#133785,#133786,#133787,
#133788,#133789,#133790,#133791,#133792,#133793,#133794,#133795,#133796,
#133797,#133798,#133799,#133800,#133801,#133802,#133803,#133804,#133805,
#133806,#133807,#133808,#133809,#133810,#133811,#133812,#133813,#133814,
#133815,#133816,#133817,#133818,#133819,#133820,#133821,#133822,#133823,
#133824,#133825,#133826,#133827,#133828,#133829,#133830,#133831,#133832,
#133833,#133834,#133835,#133836,#133837,#133838,#133839,#133840,#133841,
#133842,#133843,#133844,#133845,#133846,#133847,#133848),.UNSPECIFIED.,
 .F.,.F.,(4,2,2,2,2,2,2,2,2,2,2,2,2,2,2,2,2,2,2,2,2,2,2,2,2,2,2,2,2,2,2,
2,2,2,2,2,2,2,2,2,2,2,2,2,2,4),(0.000112843943640144,0.0344150395793074,
0.0475816383246325,0.0587690200146398,0.0673109693046341,0.0776742746139821,
0.0997465742391462,0.120127448680401,0.128509317525733,0.135289254975537,
0.140224646298994,0.146345892304485,0.168696721055489,0.196539466620812,
0.207476193689828,0.215867687975004,0.226204619100925,0.247590733136208,
0.276058306765157,0.283949747422056,0.28885942341835,0.295012543149614,
0.313697765545896,0.348258091607679,0.358533951062235,0.366921877714486,
0.37772491479056,0.406049849906477,0.428390921355262,0.435131777856181,
0.439968748744472,0.446972097379517,0.455786368887416,0.478655399225098,
0.480245614245873,0.500209382896845,0.509923033894279,0.518443987479708,
0.530386213932781,0.545079578918335,0.571611007075396,0.582071175294309,
0.587347021723258,0.592768778481349,0.604275570470769,0.627287656344573),
 .UNSPECIFIED.);
#23533=B_SPLINE_CURVE_WITH_KNOTS('',3,(#133854,#133855,#133856,#133857,
#133858,#133859,#133860,#133861,#133862,#133863,#133864,#133865,#133866,
#133867,#133868,#133869,#133870,#133871,#133872,#133873,#133874,#133875,
#133876,#133877,#133878,#133879,#133880,#133881,#133882,#133883,#133884,
#133885,#133886,#133887,#133888,#133889,#133890,#133891,#133892,#133893,
#133894,#133895,#133896,#133897,#133898,#133899,#133900,#133901,#133902,
#133903,#133904,#133905),.UNSPECIFIED.,.F.,.F.,(4,2,2,2,2,2,2,2,2,2,2,2,
2,2,2,2,2,2,2,2,2,2,2,2,2,4),(0.344554570308029,0.344695448033953,0.370408941196683,
0.382229429901131,0.387689512308191,0.392622655474436,0.401708908818249,
0.41489071511473,0.450540373360975,0.460730051156682,0.468815157898141,
0.478829209174333,0.501882341826355,0.531471648486518,0.537563112243419,
0.542412822498976,0.549970252815005,0.559708722388719,0.587337746402744,
0.607377527237151,0.617735207153022,0.627237693725668,0.642225757460128,
0.679011372906002,0.684485385955298,0.688655730947878),.UNSPECIFIED.);
#23534=B_SPLINE_CURVE_WITH_KNOTS('',3,(#133908,#133909,#133910,#133911,
#133912,#133913,#133914,#133915,#133916,#133917,#133918,#133919,#133920,
#133921,#133922,#133923,#133924,#133925,#133926,#133927,#133928,#133929,
#133930,#133931,#133932,#133933,#133934,#133935,#133936,#133937,#133938,
#133939,#133940,#133941,#133942,#133943,#133944,#133945,#133946,#133947,
#133948,#133949,#133950,#133951,#133952,#133953,#133954,#133955,#133956,
#133957,#133958,#133959,#133960,#133961,#133962,#133963,#133964,#133965,
#133966,#133967),.UNSPECIFIED.,.F.,.F.,(4,2,2,2,2,2,2,2,2,2,2,2,2,2,2,2,
2,2,2,2,2,2,2,2,2,2,2,2,2,4),(0.000112529988380809,0.0345718936956457,0.0476665506061721,
0.0588107019507166,0.0673388910924087,0.0777033809483279,0.0999073175585236,
0.120174202012848,0.128531762294313,0.135296104779885,0.140224046995345,
0.146336449042626,0.169040670185855,0.196595790121934,0.207502067193846,
0.215880876797446,0.226211031245187,0.247646363014807,0.276065348337023,
0.283948227631305,0.288851260167232,0.294989820414519,0.311844188310828,
0.336813210391308,0.352794826152219,0.361757836185347,0.370481925336095,
0.384586044921021,0.404094984019906,0.424935994621487),.UNSPECIFIED.);
#23535=B_SPLINE_CURVE_WITH_KNOTS('',3,(#133973,#133974,#133975,#133976,
#133977,#133978,#133979,#133980,#133981,#133982,#133983,#133984,#133985,
#133986,#133987,#133988,#133989,#133990,#133991,#133992,#133993,#133994,
#133995,#133996,#133997,#133998,#133999,#134000,#134001,#134002,#134003,
#134004,#134005,#134006,#134007,#134008,#134009,#134010,#134011,#134012,
#134013,#134014,#134015,#134016,#134017,#134018,#134019,#134020,#134021,
#134022,#134023,#134024,#134025,#134026,#134027,#134028,#134029,#134030,
#134031,#134032,#134033,#134034,#134035,#134036,#134037,#134038,#134039,
#134040,#134041,#134042,#134043,#134044,#134045,#134046,#134047,#134048,
#134049,#134050,#134051,#134052,#134053,#134054,#134055,#134056,#134057,
#134058,#134059,#134060,#134061,#134062),.UNSPECIFIED.,.F.,.F.,(4,2,2,2,
2,2,2,2,2,2,2,2,2,2,2,2,2,2,2,2,2,2,2,2,2,2,2,2,2,2,2,2,2,2,2,2,2,2,2,2,
2,2,2,2,4),(0.344313486464405,0.354919217679905,0.374367251033343,0.383748646768653,
0.392345856556732,0.405089960994582,0.439087634345528,0.449323145453929,
0.457075068601599,0.461929902784375,0.468150800236277,0.48582949980041,
0.521852601311326,0.531959774696942,0.540400237948904,0.551558272143675,
0.564757988389301,0.601877506238842,0.608288600784844,0.613150160477552,
0.620466393709948,0.629861599602323,0.656601237072781,0.674731088755373,
0.683983221220231,0.692635665603424,0.705834051066166,0.738772359850567,
0.75252375532549,0.758697268725943,0.76362408390867,0.771579943092398,0.782216588592994,
0.820503819569033,0.830989708733161,0.839435301198206,0.850187787984699,
0.862631532694381,0.893170698525703,0.904467358894393,0.909859092781245,
0.915105460942586,0.92552656820499,0.957906589824195,0.971485427032841),
 .UNSPECIFIED.);
#23536=B_SPLINE_CURVE_WITH_KNOTS('',3,(#134063,#134064,#134065,#134066,
#134067,#134068,#134069,#134070,#134071,#134072,#134073,#134074,#134075,
#134076,#134077,#134078,#134079,#134080,#134081,#134082,#134083,#134084,
#134085,#134086,#134087,#134088,#134089,#134090,#134091,#134092,#134093,
#134094,#134095,#134096,#134097,#134098,#134099,#134100,#134101,#134102,
#134103,#134104,#134105,#134106,#134107,#134108,#134109,#134110,#134111,
#134112,#134113,#134114,#134115,#134116),.UNSPECIFIED.,.F.,.F.,(4,2,2,2,
2,2,2,2,2,2,2,2,2,2,2,2,2,2,2,2,2,2,2,2,2,2,4),(0.000524579872864791,0.0077944514346942,
0.0151832658544194,0.0243130963212922,0.0406614428251173,0.0706592319194637,
0.0795094358608527,0.0865256870499652,0.0913710570366877,0.0981327838735026,
0.120801828274982,0.141283992141634,0.155803797723929,0.164653221110243,
0.173690270313448,0.189718555331087,0.218883005374065,0.228605913263831,
0.236105442162938,0.241047510735411,0.247603705193052,0.277710767663671,
0.293613869820421,0.306143913315913,0.31479567257371,0.324451901360994,
0.344554570308029),.UNSPECIFIED.);
#23537=B_SPLINE_CURVE_WITH_KNOTS('',3,(#134118,#134119,#134120,#134121,
#134122,#134123,#134124,#134125,#134126,#134127,#134128,#134129,#134130,
#134131,#134132,#134133,#134134,#134135,#134136,#134137,#134138,#134139,
#134140,#134141,#134142,#134143,#134144,#134145,#134146,#134147,#134148,
#134149,#134150,#134151,#134152,#134153,#134154,#134155,#134156,#134157,
#134158,#134159,#134160,#134161,#134162,#134163,#134164,#134165,#134166,
#134167,#134168,#134169,#134170,#134171,#134172,#134173,#134174,#134175),
 .UNSPECIFIED.,.F.,.F.,(4,2,2,2,2,2,2,2,2,2,2,2,2,2,2,2,2,2,2,2,2,2,2,2,
2,2,2,2,4),(0.424935994621487,0.428434306985777,0.435137547766552,0.439968088825602,
0.446986518483714,0.455831924158091,0.478908971408985,0.500193935217088,
0.509895637397591,0.518403653917941,0.53031833398969,0.544965154453378,
0.570911351546204,0.581820017785732,0.587157739882083,0.592495244586144,
0.603438191516193,0.621377752544442,0.647408712093355,0.65793107966815,
0.666349427953283,0.676983602628536,0.689231289510795,0.718422809269537,
0.730516198872072,0.736241588425334,0.741284281142336,0.750260193385671,
0.768737819720641),.UNSPECIFIED.);
#23538=B_SPLINE_CURVE_WITH_KNOTS('',3,(#134176,#134177,#134178,#134179,
#134180,#134181,#134182,#134183,#134184,#134185,#134186,#134187,#134188,
#134189,#134190,#134191,#134192,#134193,#134194,#134195,#134196,#134197,
#134198,#134199,#134200,#134201,#134202,#134203,#134204,#134205,#134206,
#134207,#134208,#134209,#134210,#134211,#134212,#134213,#134214,#134215,
#134216,#134217,#134218,#134219,#134220,#134221,#134222,#134223,#134224,
#134225,#134226,#134227,#134228,#134229,#134230,#134231,#134232,#134233,
#134234,#134235,#134236,#134237,#134238,#134239,#134240,#134241,#134242,
#134243,#134244,#134245,#134246,#134247,#134248,#134249,#134250,#134251,
#134252,#134253,#134254,#134255,#134256,#134257,#134258,#134259,#134260,
#134261,#134262,#134263),.UNSPECIFIED.,.F.,.F.,(4,2,2,2,2,2,2,2,2,2,2,2,
2,2,2,2,2,2,2,2,2,2,2,2,2,2,2,2,2,2,2,2,2,2,2,2,2,2,2,2,2,2,2,4),(0.000419556825689101,
0.0234235476872869,0.0364236724353723,0.0450369352546755,0.0543102946946294,
0.0727735427684984,0.0991442428415436,0.108485488127689,0.115769686914703,
0.120623273375649,0.127038864838353,0.154066218248185,0.172253033302996,
0.185819599851877,0.194509080518614,0.203653767132057,0.220882755561306,
0.248633390164057,0.258160573644001,0.265544247933525,0.27040623125339,
0.276759577475357,0.313958277312445,0.332675852622128,0.341976930682322,
0.35048764788506,0.363314326813168,0.395002420075205,0.406352115160209,
0.414650349205732,0.419602502276444,0.425571294009416,0.441130002729049,
0.473089471258454,0.486094566989405,0.494625665793476,0.503874881633195,
0.522087790581881,0.556583428730765,0.564691981827064,0.569621141859567,
0.575673634105917,0.59401933078766,0.627725845557793),.UNSPECIFIED.);
#23539=B_SPLINE_CURVE_WITH_KNOTS('',3,(#134269,#134270,#134271,#134272,
#134273,#134274,#134275,#134276,#134277,#134278,#134279,#134280,#134281,
#134282,#134283,#134284,#134285,#134286,#134287,#134288,#134289,#134290,
#134291,#134292,#134293,#134294,#134295,#134296,#134297,#134298,#134299,
#134300,#134301,#134302,#134303,#134304,#134305,#134306,#134307,#134308,
#134309,#134310,#134311,#134312,#134313,#134314,#134315,#134316,#134317,
#134318,#134319,#134320,#134321,#134322,#134323,#134324,#134325,#134326,
#134327,#134328,#134329,#134330,#134331,#134332,#134333,#134334,#134335,
#134336,#134337,#134338,#134339,#134340,#134341,#134342,#134343,#134344,
#134345,#134346,#134347,#134348,#134349,#134350,#134351,#134352,#134353,
#134354,#134355,#134356,#134357,#134358,#134359,#134360,#134361,#134362,
#134363,#134364,#134365,#134366,#134367,#134368,#134369,#134370,#134371,
#134372,#134373,#134374,#134375,#134376,#134377,#134378,#134379,#134380,
#134381,#134382,#134383,#134384,#134385,#134386,#134387,#134388,#134389,
#134390,#134391,#134392,#134393,#134394,#134395,#134396,#134397,#134398,
#134399,#134400,#134401,#134402,#134403,#134404,#134405,#134406,#134407,
#134408,#134409,#134410,#134411,#134412,#134413),.UNSPECIFIED.,.F.,.F.,
(4,3,3,3,3,3,3,3,3,3,3,3,3,3,3,3,3,3,3,3,3,3,3,3,3,3,3,3,3,3,3,3,3,3,3,
3,3,3,3,3,3,3,3,3,3,3,3,3,4),(24.216087767712,24.3282107965545,24.4335689263792,
24.4405143162603,24.4622569195143,24.4622900487738,24.5642705166895,24.5745672322469,
24.6866901661316,24.7987091944231,24.9106667308059,25.022605099489,25.134641376722,
25.246728416663,25.3590102860085,25.432018123817,25.4320512532201,25.5340317434683,
25.5443284199335,25.6564513434411,25.7684703651978,25.8804278988782,25.9923662686856,
26.1044025528757,26.2164896030587,26.3287714877585,26.4017793281197,26.4018124573133,
26.5037928793349,26.5140897641019,26.6262128227728,26.7382319766855,26.8501896392961,
26.9621281345857,27.0741645380486,27.1862517041689,27.2985336981754,27.3715405324224,
27.3715736589642,27.4729397859234,27.4843897011581,27.5954688655842,27.7064470887626,
27.8173685727851,27.9316099001658,28.0426142243821,28.1584740533451,28.2669736829371,
28.2743338823081),.UNSPECIFIED.);
#23540=B_SPLINE_CURVE_WITH_KNOTS('',3,(#134414,#134415,#134416,#134417,
#134418,#134419,#134420,#134421,#134422,#134423,#134424,#134425,#134426,
#134427,#134428,#134429,#134430,#134431,#134432,#134433,#134434,#134435,
#134436,#134437,#134438,#134439,#134440,#134441,#134442,#134443,#134444,
#134445,#134446,#134447,#134448,#134449,#134450,#134451,#134452,#134453,
#134454,#134455,#134456,#134457,#134458,#134459,#134460,#134461,#134462,
#134463,#134464,#134465,#134466,#134467),.UNSPECIFIED.,.F.,.F.,(4,2,2,2,
2,2,2,2,2,2,2,2,2,2,2,2,2,2,2,2,2,2,2,2,2,2,4),(0.000401297033932362,0.0045833394714876,
0.0083941896639838,0.0129672560599783,0.0197274769357702,0.04145800294407,
0.0701402862518669,0.0809963173745193,0.0894284984122356,0.0997787062367564,
0.121842191887511,0.149636983875748,0.157348925773996,0.162242131051256,
0.168519227062528,0.201420136837407,0.216784837708568,0.229061105347135,
0.237603455717508,0.247143637717364,0.266080261220836,0.29565142444061,
0.305632575109507,0.310829609526097,0.31632619907144,0.328402795445856,
0.344313486464405),.UNSPECIFIED.);
#23541=B_SPLINE_CURVE_WITH_KNOTS('',3,(#134469,#134470,#134471,#134472,
#134473,#134474,#134475,#134476,#134477,#134478,#134479,#134480,#134481,
#134482,#134483,#134484,#134485,#134486,#134487,#134488,#134489,#134490,
#134491,#134492,#134493,#134494,#134495,#134496,#134497,#134498,#134499,
#134500,#134501,#134502,#134503,#134504,#134505,#134506,#134507,#134508,
#134509,#134510,#134511,#134512,#134513,#134514,#134515,#134516,#134517,
#134518,#134519,#134520,#134521,#134522,#134523,#134524),.UNSPECIFIED.,
 .F.,.F.,(4,2,2,2,2,2,2,2,2,2,2,2,2,2,2,2,2,2,2,2,2,2,2,2,2,2,2,4),(0.627725845557793,
0.62959455629134,0.639753947806432,0.648182156686605,0.659241458900321,
0.672263694044832,0.707905999391311,0.715261384704962,0.720119965754627,
0.726606149982481,0.734502457838602,0.752500166433806,0.778447993536197,
0.788969327470095,0.797384452912912,0.808011191745445,0.820249004924034,
0.849401196897434,0.861505005868494,0.867231817069353,0.872276138310599,
0.881256199040214,0.894091794706562,0.929020784219794,0.93929260184998,
0.947634105787937,0.955769439433221,0.9717666708796),.UNSPECIFIED.);
#23542=B_SPLINE_CURVE_WITH_KNOTS('',3,(#134525,#134526,#134527,#134528,
#134529,#134530,#134531,#134532,#134533,#134534,#134535,#134536,#134537,
#134538,#134539,#134540,#134541,#134542,#134543,#134544,#134545,#134546,
#134547,#134548,#134549,#134550,#134551,#134552,#134553,#134554,#134555,
#134556,#134557,#134558,#134559,#134560,#134561,#134562,#134563,#134564,
#134565,#134566,#134567,#134568,#134569,#134570,#134571,#134572,#134573,
#134574,#134575,#134576,#134577,#134578,#134579,#134580,#134581,#134582,
#134583,#134584,#134585,#134586,#134587,#134588,#134589,#134590,#134591,
#134592,#134593,#134594,#134595,#134596,#134597,#134598,#134599,#134600,
#134601,#134602,#134603,#134604,#134605,#134606,#134607,#134608,#134609,
#134610,#134611,#134612,#134613,#134614,#134615,#134616),.UNSPECIFIED.,
 .F.,.F.,(4,2,2,2,2,2,2,2,2,2,2,2,2,2,2,2,2,2,2,2,2,2,2,2,2,2,2,2,2,2,2,
2,2,2,2,2,2,2,2,2,2,2,2,2,2,4),(1.73076609795579E-6,0.0308260776152478,
0.0411297792638463,0.0463705483701984,0.0517900282356288,0.0633270135787932,
0.0935679054319864,0.105955696862113,0.116667427218672,0.125085191458525,
0.135531025496316,0.158996962229642,0.178864854816529,0.187140885339661,
0.193842621044572,0.19868886428263,0.20577258821334,0.238558230006278,0.253108382173655,
0.264973594391783,0.273464235953274,0.283156214173948,0.304287981588959,
0.327474597593947,0.339946740811486,0.345488585806428,0.350638405712978,
0.360333271332897,0.392697215803507,0.405355520705415,0.416217202360555,
0.424560368605396,0.434834518734227,0.469613318366356,0.48255615819977,
0.491583663593267,0.496635375565032,0.502349192799566,0.514367772548698,
0.543600330747344,0.555848314144331,0.566481856131924,0.574898085660617,
0.585415364687804,0.610520755007593,0.627106652223347),.UNSPECIFIED.);
#23543=B_SPLINE_CURVE_WITH_KNOTS('',3,(#134622,#134623,#134624,#134625,
#134626,#134627,#134628,#134629,#134630,#134631,#134632,#134633,#134634,
#134635,#134636,#134637,#134638,#134639,#134640,#134641,#134642,#134643,
#134644,#134645,#134646,#134647,#134648,#134649,#134650,#134651,#134652,
#134653,#134654,#134655,#134656,#134657,#134658,#134659,#134660,#134661,
#134662,#134663,#134664,#134665,#134666,#134667,#134668,#134669,#134670,
#134671,#134672,#134673,#134674,#134675),.UNSPECIFIED.,.F.,.F.,(4,2,2,2,
2,2,2,2,2,2,2,2,2,2,2,2,2,2,2,2,2,2,2,2,2,2,4),(1.5983191600895,1.60946910178581,
1.61884493097629,1.62748074613801,1.64038564951555,1.67177729836047,1.68803128256708,
1.69404778312266,1.69911242113056,1.70779607100985,1.7199492720761,1.75725320746205,
1.76688312348883,1.77552740817065,1.7880457114298,1.80381364377214,1.83589481074534,
1.84231437036927,1.84702348653321,1.85386689188086,1.86249540869345,1.88458083085954,
1.90859939226412,1.91813484301809,1.92623635583885,1.93377128574619,1.94249761222262),
 .UNSPECIFIED.);
#23544=B_SPLINE_CURVE_WITH_KNOTS('',3,(#134677,#134678,#134679,#134680,
#134681,#134682,#134683,#134684,#134685,#134686,#134687,#134688,#134689,
#134690,#134691,#134692,#134693,#134694,#134695,#134696,#134697,#134698,
#134699,#134700,#134701,#134702,#134703,#134704,#134705,#134706,#134707,
#134708,#134709,#134710,#134711,#134712,#134713),.UNSPECIFIED.,.F.,.F.,
(4,3,3,3,3,3,3,3,3,3,3,3,4),(14.3984001269719,14.5130159814057,14.6275739868434,
14.7421032271326,14.856638223687,14.9712134956359,15.0859502774624,15.2007753249216,
15.3158186683707,15.3681613312746,15.4944270641862,15.6197373683541,15.7079562990334),
 .UNSPECIFIED.);
#23545=B_SPLINE_CURVE_WITH_KNOTS('',3,(#134716,#134717,#134718,#134719,
#134720,#134721,#134722,#134723,#134724,#134725,#134726,#134727,#134728,
#134729,#134730,#134731,#134732,#134733,#134734,#134735,#134736,#134737,
#134738,#134739,#134740,#134741,#134742,#134743,#134744,#134745,#134746,
#134747,#134748,#134749,#134750,#134751,#134752,#134753,#134754,#134755,
#134756,#134757,#134758,#134759,#134760,#134761,#134762,#134763,#134764,
#134765,#134766,#134767,#134768,#134769,#134770,#134771,#134772,#134773,
#134774,#134775,#134776,#134777,#134778,#134779,#134780,#134781,#134782,
#134783,#134784,#134785,#134786,#134787,#134788,#134789,#134790,#134791,
#134792,#134793,#134794,#134795,#134796,#134797,#134798,#134799,#134800,
#134801,#134802,#134803,#134804,#134805,#134806,#134807),.UNSPECIFIED.,
 .F.,.F.,(4,2,2,2,2,2,2,2,2,2,2,2,2,2,2,2,2,2,2,2,2,2,2,2,2,2,2,2,2,2,2,
2,2,2,2,2,2,2,2,2,2,2,2,2,2,4),(0.000112838215867501,0.0344137848853368,
0.0475811293693514,0.0587689530819971,0.0673110177778552,0.0776742517777449,
0.0997450585740924,0.120126913328797,0.128508978000661,0.135289040547425,
0.140224478619107,0.146345772442547,0.16869308144312,0.19653936634855,0.207475967120287,
0.2158674386007,0.226204420266539,0.247591969570469,0.276058453560075,0.283949792254572,
0.2888594371998,0.295012537477586,0.313697743449704,0.348258117572018,0.358533952470444,
0.366921848083298,0.377724819707815,0.406049259932434,0.428390970158201,
0.435131806471044,0.439968768855761,0.446972104919837,0.45578635292522,
0.478655233889584,0.480248254062548,0.500217393499176,0.50992868790014,
0.518450149366918,0.530397555504147,0.545101171597835,0.57166148007292,
0.582088430897414,0.587359340365255,0.592786863115678,0.604335610698444,
0.627287566072145),.UNSPECIFIED.);
#23546=B_SPLINE_CURVE_WITH_KNOTS('',3,(#134809,#134810,#134811,#134812,
#134813,#134814,#134815,#134816,#134817,#134818,#134819,#134820,#134821,
#134822,#134823,#134824,#134825,#134826,#134827,#134828,#134829,#134830,
#134831,#134832,#134833,#134834,#134835,#134836,#134837,#134838,#134839,
#134840,#134841,#134842,#134843,#134844,#134845,#134846,#134847,#134848,
#134849,#134850,#134851,#134852,#134853,#134854,#134855,#134856,#134857,
#134858,#134859,#134860,#134861,#134862,#134863,#134864,#134865,#134866,
#134867,#134868,#134869,#134870,#134871,#134872,#134873,#134874,#134875,
#134876,#134877,#134878,#134879,#134880,#134881,#134882,#134883,#134884,
#134885,#134886,#134887,#134888,#134889,#134890,#134891,#134892,#134893,
#134894,#134895,#134896,#134897,#134898,#134899,#134900,#134901,#134902,
#134903,#134904,#134905,#134906,#134907,#134908,#134909,#134910,#134911,
#134912,#134913,#134914,#134915,#134916,#134917,#134918,#134919,#134920,
#134921,#134922,#134923,#134924,#134925,#134926,#134927,#134928,#134929,
#134930,#134931,#134932,#134933,#134934,#134935,#134936,#134937,#134938,
#134939,#134940,#134941,#134942,#134943,#134944,#134945,#134946,#134947,
#134948,#134949,#134950),.UNSPECIFIED.,.F.,.F.,(4,2,2,2,2,2,2,2,2,2,2,2,
2,2,2,2,2,2,2,2,2,2,2,2,2,2,2,2,2,2,2,2,2,2,2,2,2,2,2,2,2,2,2,2,2,2,2,2,
2,2,2,2,2,2,2,2,2,2,2,2,2,2,2,2,2,2,2,2,2,2,4),(6.82072967247012E-5,0.020612855930782,
0.0289793048578245,0.0374722935793014,0.0472454148643254,0.07016917077208,
0.0985873974547638,0.106463587934993,0.111372235066616,0.117553851921224,
0.151088051442694,0.166252240727669,0.178428109610994,0.186956007413909,
0.196526979493893,0.216053714943285,0.240778730125056,0.249885028192609,
0.257045289735006,0.26189945094549,0.268555116618211,0.293782279264809,
0.312773881779431,0.326680982466161,0.335423165916425,0.344515934354849,
0.361220486014547,0.389600788076956,0.399211608413098,0.406641268814885,
0.411512630137261,0.417855827415522,0.445667228247553,0.463517194718252,
0.476941553742677,0.485620356841447,0.494812971120406,0.512407478679775,
0.543683969011262,0.554307856288399,0.55960027585328,0.564977267092943,
0.576182088279459,0.594918799241663,0.619813282836159,0.630332419720432,
0.638760589222806,0.649426524278923,0.66172664418531,0.691277440738422,
0.703020891435863,0.708692813393365,0.713778154448283,0.72300524960665,
0.736403914840773,0.772023656998422,0.781766847232403,0.790263071456699,
0.802074302205074,0.816511714099025,0.842313969786416,0.853715704411164,
0.859120950462794,0.864389723841491,0.874851519250536,0.907457399377032,
0.924306359097852,0.933414594761016,0.942143430186657,0.952991945071345,
0.971189088135237),.UNSPECIFIED.);
#23547=B_SPLINE_CURVE_WITH_KNOTS('',3,(#134951,#134952,#134953,#134954,
#134955,#134956,#134957,#134958,#134959,#134960,#134961,#134962,#134963,
#134964,#134965,#134966,#134967,#134968,#134969,#134970,#134971,#134972,
#134973,#134974,#134975,#134976,#134977,#134978,#134979,#134980,#134981,
#134982,#134983,#134984,#134985,#134986,#134987,#134988,#134989,#134990,
#134991,#134992,#134993,#134994,#134995,#134996,#134997,#134998,#134999,
#135000,#135001,#135002,#135003,#135004,#135005,#135006,#135007,#135008,
#135009,#135010,#135011,#135012,#135013,#135014,#135015,#135016,#135017,
#135018,#135019,#135020,#135021,#135022,#135023,#135024,#135025,#135026,
#135027,#135028,#135029,#135030,#135031,#135032,#135033,#135034,#135035,
#135036,#135037,#135038,#135039,#135040,#135041,#135042,#135043,#135044,
#135045,#135046,#135047,#135048,#135049,#135050,#135051,#135052,#135053,
#135054,#135055,#135056,#135057,#135058,#135059,#135060,#135061,#135062,
#135063,#135064,#135065,#135066,#135067,#135068,#135069,#135070,#135071,
#135072,#135073,#135074,#135075,#135076,#135077,#135078,#135079,#135080,
#135081,#135082,#135083,#135084,#135085,#135086,#135087,#135088,#135089,
#135090,#135091,#135092,#135093,#135094,#135095,#135096),.UNSPECIFIED.,
 .F.,.F.,(4,2,2,2,2,2,2,2,2,2,2,2,2,2,2,2,2,2,2,2,2,2,2,2,2,2,2,2,2,2,2,
2,2,2,2,2,2,2,2,2,2,2,2,2,2,2,2,2,2,2,2,2,2,2,2,2,2,2,2,2,2,2,2,2,2,2,2,
2,2,2,2,2,4),(0.627106652223347,0.629123486082643,0.637147607467664,0.643706619587023,
0.648559944568491,0.655817785236257,0.691615180300921,0.704651951605286,
0.71572056621102,0.724150494292224,0.734305893756065,0.769953866615976,
0.782592043807738,0.791484964292521,0.796517901061968,0.802275928685794,
0.814579293200728,0.839961023065592,0.859510168351007,0.868892561545163,
0.87747217535699,0.890146638219859,0.924255507357647,0.93449884137058,0.942252760621376,
0.947102244961131,0.953303129879324,0.971212130986432,1.00691574265751,
1.01705796596725,1.02548279599575,1.0365510806174,1.04959199381931,1.08542572379961,
1.09266652813928,1.09751725079561,1.10408354879256,1.11211938894129,1.1307803944364,
1.1558058844306,1.16632418249714,1.17474254277447,1.18538093246616,1.19763834622744,
1.22692259217994,1.23889768048791,1.24460810929962,1.24967941946219,1.25878977346316,
1.27191966404575,1.3060112483004,1.31636527760657,1.324801785069,1.33566829156301,
1.3644093641721,1.38612043426777,1.39287886762142,1.39770785637703,1.40466892816411,
1.41342214606773,1.43598649976264,1.45827454192538,1.4678799978639,1.47633265693326,
1.4881884256979,1.5027503126632,1.53685237531525,1.54323909784667,1.54809120222948,
1.55538695180452,1.56473743996364,1.5910810217434,1.5983191600895),
 .UNSPECIFIED.);
#23548=B_SPLINE_CURVE_WITH_KNOTS('',3,(#135098,#135099,#135100,#135101,
#135102,#135103,#135104,#135105,#135106,#135107,#135108,#135109,#135110,
#135111,#135112,#135113,#135114,#135115,#135116,#135117,#135118,#135119,
#135120,#135121,#135122,#135123,#135124,#135125,#135126,#135127,#135128,
#135129,#135130,#135131,#135132,#135133,#135134,#135135,#135136,#135137,
#135138,#135139,#135140,#135141,#135142,#135143,#135144,#135145,#135146,
#135147,#135148,#135149,#135150,#135151,#135152,#135153,#135154,#135155,
#135156,#135157,#135158,#135159,#135160,#135161,#135162,#135163,#135164,
#135165,#135166,#135167,#135168,#135169,#135170,#135171,#135172,#135173,
#135174,#135175,#135176,#135177,#135178,#135179,#135180,#135181,#135182,
#135183,#135184,#135185,#135186,#135187,#135188,#135189,#135190,#135191,
#135192,#135193,#135194,#135195,#135196,#135197,#135198,#135199,#135200,
#135201,#135202,#135203,#135204,#135205,#135206,#135207,#135208,#135209,
#135210,#135211,#135212,#135213,#135214,#135215,#135216,#135217,#135218,
#135219,#135220,#135221,#135222,#135223,#135224,#135225,#135226,#135227,
#135228,#135229,#135230,#135231,#135232,#135233,#135234,#135235,#135236,
#135237,#135238,#135239),.UNSPECIFIED.,.F.,.F.,(4,2,2,2,2,2,2,2,2,2,2,2,
2,2,2,2,2,2,2,2,2,2,2,2,2,2,2,2,2,2,2,2,2,2,2,2,2,2,2,2,2,2,2,2,2,2,2,2,
2,2,2,2,2,2,2,2,2,2,2,2,2,2,2,2,2,2,2,2,2,2,4),(6.82064154310527E-5,0.0206122609103592,
0.0289788297288812,0.0374718670697915,0.0472447831254516,0.0701612291856842,
0.0985862746444113,0.106463074562659,0.111371791601236,0.117553109412752,
0.151089409067014,0.166252939478315,0.178428485624057,0.186956358547689,
0.196527482397229,0.216052479328968,0.240778433475478,0.249884875574736,
0.257045216509811,0.261899385421799,0.26855500119635,0.293782789437433,
0.312774097284305,0.326681078434405,0.335423249713859,0.344516048076797,
0.361220826901406,0.389600866084423,0.399211654980418,0.406641299612127,
0.411512662197177,0.417855877817988,0.445667116793014,0.463517154956275,
0.476941547929924,0.485620361207113,0.494812979986727,0.512407480102826,
0.543683926524452,0.554307847707887,0.559600275259536,0.564977269815557,
0.576182094468019,0.594918810755804,0.619813286211509,0.630332428002734,
0.638760605202319,0.649426557329208,0.661726703277235,0.691277663257335,
0.703020968280399,0.70869286743362,0.713778228110877,0.723005439231197,
0.736404372936923,0.772023388484475,0.781766664709639,0.790262880809526,
0.802073962519849,0.816511078884114,0.842313178009023,0.853715464178983,
0.85912078949944,0.86438950272873,0.874850875776926,0.907453929464112,0.924305179270456,
0.933413686956909,0.942142364010327,0.952991291839689,0.97118908114431),
 .UNSPECIFIED.);
#23549=B_SPLINE_CURVE_WITH_KNOTS('',3,(#135240,#135241,#135242,#135243,
#135244,#135245,#135246,#135247,#135248,#135249,#135250,#135251,#135252,
#135253,#135254,#135255,#135256,#135257,#135258,#135259,#135260,#135261,
#135262,#135263,#135264,#135265,#135266,#135267,#135268,#135269,#135270,
#135271,#135272,#135273,#135274,#135275,#135276,#135277,#135278,#135279,
#135280,#135281,#135282,#135283,#135284,#135285,#135286,#135287,#135288,
#135289,#135290,#135291,#135292,#135293,#135294,#135295,#135296,#135297,
#135298,#135299,#135300,#135301,#135302,#135303,#135304,#135305,#135306,
#135307,#135308,#135309,#135310,#135311,#135312,#135313,#135314,#135315,
#135316,#135317,#135318,#135319,#135320,#135321,#135322,#135323,#135324,
#135325,#135326,#135327,#135328,#135329,#135330,#135331,#135332,#135333,
#135334,#135335,#135336,#135337,#135338,#135339,#135340,#135341,#135342,
#135343,#135344,#135345,#135346,#135347,#135348,#135349,#135350,#135351,
#135352,#135353,#135354,#135355,#135356,#135357,#135358,#135359,#135360,
#135361,#135362,#135363,#135364,#135365,#135366,#135367,#135368,#135369,
#135370,#135371,#135372,#135373,#135374,#135375,#135376,#135377,#135378,
#135379,#135380,#135381,#135382,#135383,#135384,#135385),.UNSPECIFIED.,
 .F.,.F.,(4,2,2,2,2,2,2,2,2,2,2,2,2,2,2,2,2,2,2,2,2,2,2,2,2,2,2,2,2,2,2,
2,2,2,2,2,2,2,2,2,2,2,2,2,2,2,2,2,2,2,2,2,2,2,2,2,2,2,2,2,2,2,2,2,2,2,2,
2,2,2,2,2,4),(0.627052488170293,0.629097476923593,0.637108433107913,0.643659753834069,
0.648513112425859,0.655779516904756,0.691558478122418,0.704592503143053,
0.715659250357901,0.724088338715216,0.734243367480604,0.769883613171745,
0.782522117280072,0.791414875982714,0.796447434225467,0.802204710988669,
0.814505448463294,0.839885179036521,0.859433710725933,0.868815335481488,
0.877394104971846,0.890067035347798,0.924173302861861,0.934415734856313,
0.94216895647577,0.947017985429099,0.95321825645414,0.971126021556437,1.00682566147047,
1.01696700696627,1.02539102365338,1.0364581126144,1.04949752150781,1.08532515497896,
1.092566953772,1.09741729528189,1.10398164108412,1.11201438539871,1.13066222401229,
1.15570127483238,1.16621895058941,1.17463650550304,1.18527347923898,1.1975290058821,
1.22680537517602,1.23878404896918,1.24449471591593,1.24956519975383,1.25867215500841,
1.27179493028354,1.30589953622533,1.31625036145358,1.32468619493319,1.33555446558064,
1.36432230424464,1.38599368746079,1.39275208831188,1.39758059777592,1.40454029987336,
1.41329140989759,1.43584607482569,1.458141909584,1.4677465454054,1.47619830951384,
1.48805249355466,1.50261212623886,1.53671332499098,1.54309921399244,1.54795081627567,
1.55524594764188,1.5645956971375,1.59093771395068,1.59817392798203),
 .UNSPECIFIED.);
#23550=B_SPLINE_CURVE_WITH_KNOTS('',3,(#135388,#135389,#135390,#135391,
#135392,#135393,#135394,#135395,#135396,#135397,#135398,#135399,#135400,
#135401,#135402,#135403,#135404,#135405,#135406,#135407,#135408,#135409,
#135410,#135411,#135412,#135413,#135414,#135415,#135416,#135417,#135418,
#135419,#135420,#135421,#135422,#135423,#135424,#135425,#135426,#135427,
#135428,#135429,#135430,#135431,#135432,#135433,#135434,#135435,#135436,
#135437,#135438,#135439,#135440,#135441,#135442,#135443,#135444,#135445,
#135446,#135447,#135448,#135449,#135450,#135451,#135452,#135453,#135454,
#135455,#135456,#135457,#135458,#135459,#135460),.UNSPECIFIED.,.F.,.F.,
(4,3,3,3,3,3,3,3,3,3,3,3,3,3,3,3,3,3,3,3,3,3,3,3,4),(5.66555025349161,5.77596501629269,
5.78359419481329,5.81852702745744,5.81856722581613,5.92802936256689,5.93978737635397,
6.05763571976858,6.17537452312111,6.29305298232785,6.41687184427559,6.53465411287049,
6.65250789513665,6.76130413452367,6.77055655343442,6.78828803449599,6.78832843011882,
6.89648185188166,6.90464476357801,7.02079948264988,7.13684497738031,7.25288906167345,
7.36892199840986,7.48510590926794,7.59274844756046),.UNSPECIFIED.);
#23551=B_SPLINE_CURVE_WITH_KNOTS('',3,(#135461,#135462,#135463,#135464,
#135465,#135466,#135467,#135468,#135469,#135470,#135471,#135472,#135473,
#135474,#135475,#135476,#135477,#135478,#135479,#135480,#135481,#135482,
#135483,#135484,#135485,#135486,#135487,#135488,#135489,#135490,#135491,
#135492,#135493,#135494,#135495,#135496,#135497,#135498,#135499,#135500,
#135501,#135502,#135503,#135504,#135505,#135506,#135507,#135508,#135509,
#135510,#135511,#135512,#135513,#135514,#135515,#135516,#135517,#135518,
#135519,#135520,#135521,#135522,#135523,#135524,#135525,#135526,#135527,
#135528,#135529,#135530,#135531,#135532,#135533,#135534,#135535,#135536,
#135537,#135538,#135539,#135540,#135541,#135542,#135543,#135544,#135545,
#135546,#135547,#135548,#135549,#135550,#135551,#135552,#135553,#135554,
#135555,#135556,#135557,#135558,#135559,#135560,#135561,#135562,#135563,
#135564,#135565,#135566,#135567,#135568,#135569,#135570,#135571,#135572,
#135573,#135574,#135575,#135576,#135577,#135578,#135579,#135580,#135581,
#135582,#135583,#135584,#135585,#135586,#135587,#135588,#135589,#135590,
#135591,#135592,#135593,#135594,#135595,#135596,#135597,#135598,#135599,
#135600,#135601,#135602,#135603,#135604,#135605,#135606,#135607,#135608,
#135609,#135610,#135611,#135612,#135613,#135614,#135615,#135616,#135617,
#135618,#135619,#135620,#135621,#135622,#135623,#135624,#135625,#135626),
 .UNSPECIFIED.,.F.,.F.,(4,3,3,3,3,3,3,3,3,3,3,3,3,3,3,3,3,3,3,3,3,3,3,3,
3,3,3,3,3,3,3,3,3,3,3,3,3,3,3,3,3,3,3,3,3,3,3,3,3,3,3,3,3,3,3,4),(7.5927484481567,
7.70848931082287,7.75804920753855,7.75808963442151,7.86752047919751,7.87930978495934,
7.99714701095087,8.11487440634642,8.23254119187242,8.35636860358536,8.47413868997202,
8.59198013199231,8.70078884284455,8.71001632278144,8.72781047661061,8.72785083872419,
8.83728642518644,8.84907098926203,8.96690551936438,9.08463022262083,9.20229432567408,
9.32612375501228,9.44389122085705,9.56173006773944,9.67053220577472,9.67976372019558,
9.69757165256406,9.69761204302688,9.80704288732126,9.81883219356472,9.9366641213659,
10.0543861697222,10.1720475710507,10.2958789901204,10.413643673577,10.5314797142669,
10.6402827589719,10.6495105488693,10.6673328569863,10.6673732473296,10.7768055714159,
10.7885933978674,10.9064273960726,11.0241515432087,11.1418150671119,11.265644913242,
11.383411749779,11.5012499509012,11.6100540546258,11.6192829392659,11.6370940679108,
11.6371344516323,11.7464312636471,11.7551568359126,11.8729941352346,11.9496359926862),
 .UNSPECIFIED.);
#23552=B_SPLINE_CURVE_WITH_KNOTS('',3,(#135627,#135628,#135629,#135630,
#135631,#135632,#135633,#135634,#135635,#135636,#135637,#135638,#135639,
#135640,#135641,#135642,#135643,#135644,#135645,#135646,#135647,#135648,
#135649,#135650,#135651,#135652,#135653,#135654,#135655,#135656,#135657,
#135658,#135659,#135660,#135661,#135662,#135663,#135664,#135665,#135666,
#135667,#135668,#135669,#135670,#135671,#135672,#135673,#135674,#135675,
#135676,#135677,#135678,#135679,#135680,#135681,#135682,#135683,#135684,
#135685,#135686,#135687,#135688,#135689,#135690,#135691,#135692,#135693,
#135694,#135695,#135696,#135697,#135698,#135699,#135700,#135701,#135702,
#135703,#135704,#135705,#135706,#135707,#135708,#135709,#135710,#135711,
#135712,#135713,#135714,#135715,#135716,#135717,#135718,#135719,#135720,
#135721,#135722,#135723,#135724,#135725,#135726,#135727,#135728,#135729,
#135730,#135731,#135732,#135733,#135734,#135735,#135736,#135737,#135738,
#135739,#135740,#135741,#135742,#135743,#135744,#135745,#135746,#135747,
#135748,#135749,#135750),.UNSPECIFIED.,.F.,.F.,(4,2,2,2,2,2,2,2,2,2,2,2,
2,2,2,2,2,2,2,2,2,2,2,2,2,2,2,2,2,2,2,2,2,2,2,2,2,2,2,2,2,2,2,2,2,2,2,2,
2,2,2,2,2,2,2,2,2,2,2,2,2,4),(-1.04064001717697,-1.03027141349264,-1.0173478683752,
-0.993383177184256,-0.985957107213174,-0.981054610570191,-0.973672075358925,
-0.963727412468284,-0.931041109103776,-0.922049514266625,-0.913099173519084,
-0.895464554635867,-0.870256799917985,-0.86291344632528,-0.85801155538961,
-0.85054911280665,-0.840436223537567,-0.808127266458275,-0.79911329869858,
-0.790169851509594,-0.772700593908835,-0.748480260777749,-0.740479819189106,
-0.73555036712696,-0.728595208219088,-0.719535862834643,-0.689428311189464,
-0.679207808539281,-0.670704191720385,-0.658644789437106,-0.625055523110738,
-0.617373530048558,-0.612479565454441,-0.605389999076659,-0.596042434022061,
-0.569689584841247,-0.55810877463022,-0.549686257406334,-0.53933660593639,
-0.527203875983819,-0.50322166815262,-0.494849075582067,-0.489911422424503,
-0.483248975275109,-0.461281902412592,-0.439891122091201,-0.43066811618859,
-0.421820971123292,-0.405920071611398,-0.376490662455969,-0.370021060472215,
-0.364920156106881,-0.355495588887186,-0.34045320617814,-0.317839437214019,
-0.308616145284517,-0.299638728241579,-0.282779212407393,-0.258916192866437,
-0.250058535195703,-0.245187517922973,-0.244113824073537),.UNSPECIFIED.);
#23553=B_SPLINE_CURVE_WITH_KNOTS('',3,(#135753,#135754,#135755,#135756,
#135757,#135758,#135759,#135760,#135761,#135762,#135763,#135764,#135765,
#135766,#135767,#135768,#135769,#135770,#135771,#135772,#135773,#135774,
#135775,#135776,#135777,#135778,#135779,#135780,#135781,#135782,#135783,
#135784,#135785,#135786,#135787,#135788,#135789,#135790,#135791,#135792,
#135793,#135794,#135795,#135796,#135797,#135798,#135799,#135800,#135801,
#135802,#135803,#135804,#135805,#135806,#135807,#135808,#135809,#135810,
#135811,#135812,#135813,#135814,#135815,#135816,#135817,#135818,#135819,
#135820,#135821,#135822,#135823,#135824,#135825),.UNSPECIFIED.,.F.,.F.,
(4,3,3,3,3,3,3,3,3,3,3,3,3,3,3,3,3,3,3,3,3,3,3,3,4),(5.66554986601471,5.77596453150268,
5.78359371610427,5.81852702174705,5.81856722581613,5.92802930197335,5.93978737635397,
6.0576357094371,6.17537450206838,6.29305295018594,6.41687182016916,6.53465407689312,
6.65250784703394,6.76130412196615,6.77055649293766,6.78828802954264,6.78832843011882,
6.8964818874404,6.90464479286087,7.02079954171015,7.13684506667047,7.25288918170985,
7.36892214952182,7.48510609168556,7.59274844756024),.UNSPECIFIED.);
#23554=B_SPLINE_CURVE_WITH_KNOTS('',3,(#135826,#135827,#135828,#135829,
#135830,#135831,#135832,#135833,#135834,#135835,#135836,#135837,#135838,
#135839,#135840,#135841,#135842,#135843,#135844,#135845,#135846,#135847,
#135848,#135849,#135850,#135851,#135852,#135853,#135854,#135855,#135856,
#135857,#135858,#135859,#135860,#135861,#135862,#135863,#135864,#135865,
#135866,#135867,#135868,#135869,#135870,#135871,#135872,#135873,#135874,
#135875,#135876,#135877,#135878,#135879,#135880,#135881,#135882,#135883,
#135884,#135885,#135886,#135887,#135888,#135889,#135890,#135891,#135892,
#135893,#135894,#135895,#135896,#135897,#135898,#135899,#135900,#135901,
#135902,#135903,#135904,#135905,#135906,#135907,#135908,#135909,#135910,
#135911,#135912,#135913,#135914,#135915,#135916,#135917,#135918,#135919,
#135920,#135921,#135922,#135923,#135924,#135925,#135926,#135927,#135928,
#135929,#135930,#135931,#135932,#135933,#135934,#135935,#135936,#135937,
#135938,#135939,#135940,#135941,#135942,#135943,#135944,#135945,#135946,
#135947,#135948,#135949,#135950,#135951,#135952,#135953,#135954,#135955,
#135956,#135957,#135958,#135959,#135960,#135961,#135962,#135963,#135964,
#135965,#135966,#135967,#135968,#135969,#135970,#135971,#135972,#135973,
#135974,#135975,#135976,#135977,#135978,#135979,#135980,#135981,#135982,
#135983,#135984,#135985,#135986,#135987,#135988,#135989,#135990,#135991),
 .UNSPECIFIED.,.F.,.F.,(4,3,3,3,3,3,3,3,3,3,3,3,3,3,3,3,3,3,3,3,3,3,3,3,
3,3,3,3,3,3,3,3,3,3,3,3,3,3,3,3,3,3,3,3,3,3,3,3,3,3,3,3,3,3,3,4),(7.59274844815668,
7.70848933226218,7.75804920252765,7.7580896344215,7.86752047552237,7.87930978495934,
7.99714699496723,8.11487437422409,8.23254114349144,8.35636856729962,8.47413863735006,
8.59198006303149,8.70078875715278,8.71001623760722,8.72781047141427,8.72785083872419,
8.83728641600613,8.84907098926203,8.96690551890705,9.08463022165414,9.20229432414697,
9.32612375386695,9.44389121902953,9.56173006518838,9.67053220806784,9.67976371686772,
9.6975716474907,9.69761204302688,9.80704289295715,9.81883219356472,9.93666412617729,
10.0543861794204,10.1720475857004,10.2958790011077,10.4136436896112,10.5314797353737,
10.6402827787652,10.6495105750451,10.6673328518942,10.6673732473296,10.7768055701125,
10.7885933978674,10.9064273934618,11.0241515379578,11.1418150591975,11.2656449073062,
11.3834117411574,11.5012499395899,11.6100540394642,11.6192829252808,11.6370940627961,
11.6371344516323,11.7464312623365,11.7551568362625,11.8729941358588,11.9496356025186),
 .UNSPECIFIED.);
#23555=B_SPLINE_CURVE_WITH_KNOTS('',3,(#135992,#135993,#135994,#135995,
#135996,#135997,#135998,#135999,#136000,#136001,#136002,#136003,#136004,
#136005,#136006,#136007,#136008,#136009,#136010,#136011,#136012,#136013,
#136014,#136015,#136016,#136017,#136018,#136019,#136020,#136021,#136022,
#136023,#136024,#136025,#136026,#136027,#136028,#136029,#136030,#136031,
#136032,#136033,#136034,#136035,#136036,#136037,#136038,#136039,#136040,
#136041,#136042,#136043,#136044,#136045,#136046,#136047,#136048,#136049,
#136050,#136051,#136052,#136053,#136054,#136055,#136056,#136057,#136058,
#136059,#136060,#136061,#136062,#136063,#136064,#136065,#136066,#136067,
#136068,#136069,#136070,#136071,#136072,#136073,#136074,#136075,#136076,
#136077,#136078,#136079,#136080,#136081,#136082,#136083,#136084,#136085,
#136086,#136087,#136088,#136089,#136090,#136091,#136092,#136093,#136094,
#136095,#136096,#136097,#136098,#136099,#136100,#136101,#136102,#136103,
#136104,#136105,#136106,#136107,#136108,#136109,#136110,#136111,#136112,
#136113,#136114,#136115),.UNSPECIFIED.,.F.,.F.,(4,2,2,2,2,2,2,2,2,2,2,2,
2,2,2,2,2,2,2,2,2,2,2,2,2,2,2,2,2,2,2,2,2,2,2,2,2,2,2,2,2,2,2,2,2,2,2,2,
2,2,2,2,2,2,2,2,2,2,2,2,2,4),(-1.04064761107749,-1.03667653359214,-1.02057252852155,
-0.9903553805898,-0.984358690916432,-0.979237994977344,-0.969036797980125,
-0.951517128197997,-0.931710771399382,-0.922578938958349,-0.913747451701676,
-0.897661246305512,-0.867498616782207,-0.861470377670638,-0.856362594494266,
-0.846294480025667,-0.829237260592109,-0.808850442624188,-0.799685899242007,
-0.790862380332336,-0.774944861212517,-0.745412546770826,-0.739002804337929,
-0.733993752195202,-0.72497767286612,-0.695095836313415,-0.682350248058098,
-0.673795801795949,-0.663890116730539,-0.652668140312166,-0.62480111204984,
-0.617288212082119,-0.612398318438083,-0.605161188422243,-0.595510337990656,
-0.569063629920645,-0.557792264867719,-0.549381259618363,-0.538805352598925,
-0.526220113176564,-0.502072016440112,-0.49438018345918,-0.489478824102436,
-0.482360419432393,-0.472978497189683,-0.44657915995887,-0.434969508366888,
-0.426469154547465,-0.415917996104292,-0.403435536234545,-0.379226701275057,
-0.37140085348607,-0.366413756853001,-0.359021254014121,-0.349080449971626,
-0.317055397661656,-0.30800989081409,-0.298869341415305,-0.279457361709301,
-0.253038691613122,-0.247188096201178,-0.244126851835458),.UNSPECIFIED.);
#23556=B_SPLINE_CURVE_WITH_KNOTS('',3,(#136240,#136241,#136242,#136243,
#136244,#136245,#136246,#136247,#136248,#136249,#136250,#136251,#136252,
#136253),.UNSPECIFIED.,.F.,.F.,(4,2,2,2,2,2,4),(1.58567647220938E-6,0.0466881077856908,
0.0920988348773926,0.143330833613337,0.192991558600317,0.240911899931117,
0.29038450507933),.UNSPECIFIED.);
#23557=B_SPLINE_CURVE_WITH_KNOTS('',3,(#136254,#136255,#136256,#136257,
#136258,#136259,#136260,#136261,#136262,#136263,#136264,#136265,#136266,
#136267,#136268,#136269,#136270,#136271,#136272,#136273,#136274,#136275,
#136276,#136277,#136278,#136279,#136280,#136281,#136282,#136283,#136284,
#136285,#136286,#136287,#136288,#136289,#136290,#136291,#136292,#136293,
#136294,#136295,#136296,#136297,#136298,#136299,#136300,#136301,#136302,
#136303,#136304,#136305,#136306,#136307,#136308,#136309,#136310,#136311,
#136312,#136313,#136314,#136315,#136316,#136317,#136318,#136319,#136320,
#136321,#136322,#136323,#136324,#136325,#136326,#136327,#136328,#136329,
#136330,#136331,#136332,#136333,#136334,#136335),.UNSPECIFIED.,.F.,.F.,
(4,3,3,3,3,3,3,3,3,3,3,3,3,3,3,3,3,3,3,3,3,3,3,3,3,3,3,4),(0.,0.0154790975076392,
0.0309581950152783,0.043346867455363,0.0480167577448785,0.052157240862597,
0.0686255293071033,0.085061105479412,0.0963127227435478,0.100794587159636,
0.104383686997236,0.12145541211408,0.130067574535955,0.146660502151626,
0.15583969909837,0.158551507968915,0.175605845203202,0.193054946625637,
0.204601396301158,0.210946851258842,0.215063043944209,0.233049916450152,
0.242953934326418,0.247562205886623,0.251095943169411,0.269300892692474,
0.272665987955216,0.285115833988478),.UNSPECIFIED.);
#23558=B_SPLINE_CURVE_WITH_KNOTS('',3,(#136460,#136461,#136462,#136463,
#136464,#136465,#136466,#136467,#136468,#136469,#136470,#136471,#136472,
#136473,#136474,#136475,#136476,#136477,#136478,#136479,#136480,#136481,
#136482,#136483,#136484,#136485,#136486,#136487,#136488,#136489,#136490,
#136491,#136492,#136493,#136494,#136495,#136496,#136497,#136498,#136499,
#136500,#136501,#136502,#136503,#136504,#136505,#136506,#136507,#136508,
#136509,#136510,#136511,#136512,#136513,#136514,#136515,#136516,#136517,
#136518,#136519,#136520,#136521,#136522,#136523,#136524,#136525,#136526,
#136527,#136528,#136529,#136530,#136531,#136532,#136533,#136534,#136535,
#136536,#136537,#136538,#136539,#136540,#136541),.UNSPECIFIED.,.F.,.F.,
(4,3,3,3,3,3,3,3,3,3,3,3,3,3,3,3,3,3,3,3,3,3,3,3,3,3,3,4),(0.,0.0154790634400372,
0.0309581268800745,0.0433468078370607,0.048016628498302,0.0521572525180448,
0.0684584781979448,0.0850610915406634,0.0963127122894887,0.10079456566722,
0.104383680276898,0.121455407850578,0.130067574535964,0.146660523123985,
0.155839744528338,0.158551576529395,0.175605937118379,0.193095393916,0.204601449529331,
0.21094683907126,0.215063044511372,0.233049918293188,0.2429539357087,0.247562235404507,
0.251095975207792,0.269300923802189,0.272665987955236,0.285115831934067),
 .UNSPECIFIED.);
#23559=B_SPLINE_CURVE_WITH_KNOTS('',3,(#136543,#136544,#136545,#136546),
 .UNSPECIFIED.,.F.,.F.,(4,4),(0.,0.00918658431906933),.UNSPECIFIED.);
#23560=B_SPLINE_CURVE_WITH_KNOTS('',3,(#136547,#136548,#136549,#136550,
#136551,#136552,#136553,#136554,#136555,#136556,#136557,#136558,#136559,
#136560,#136561,#136562,#136563,#136564,#136565,#136566,#136567,#136568,
#136569,#136570,#136571,#136572,#136573,#136574,#136575,#136576,#136577,
#136578,#136579,#136580,#136581,#136582,#136583,#136584,#136585,#136586,
#136587,#136588,#136589,#136590,#136591,#136592,#136593,#136594,#136595,
#136596,#136597,#136598,#136599,#136600,#136601,#136602,#136603,#136604,
#136605,#136606,#136607,#136608,#136609,#136610,#136611,#136612,#136613,
#136614,#136615,#136616,#136617,#136618,#136619,#136620,#136621,#136622,
#136623,#136624,#136625),.UNSPECIFIED.,.F.,.F.,(4,3,3,3,3,3,3,3,3,3,3,3,
3,3,3,3,3,3,3,3,3,3,3,3,3,3,4),(0.,0.0178509406758339,0.0360833708446063,
0.0497914557540533,0.0564440624232981,0.0594975215358368,0.0772253906875525,
0.0946647317535434,0.107092444205114,0.114964947860173,0.118088073305871,
0.134959943033528,0.144375581559826,0.160821883027944,0.168625126520761,
0.173118085073618,0.189888464885431,0.206622922460632,0.217641805290516,
0.223770976991618,0.22717570174071,0.243238325838015,0.252063979588582,
0.255940334406271,0.271478860666626,0.275945993304769,0.286347380332248),
 .UNSPECIFIED.);
#23561=B_SPLINE_CURVE_WITH_KNOTS('',3,(#136763,#136764,#136765,#136766,
#136767,#136768,#136769,#136770,#136771,#136772,#136773,#136774,#136775,
#136776),.UNSPECIFIED.,.F.,.F.,(4,2,2,2,2,2,4),(1.58595928405246E-6,0.0466880966579777,
0.0920988245562084,0.143330891570577,0.192991652192899,0.240911943591573,
0.290384482497107),.UNSPECIFIED.);
#23562=B_SPLINE_CURVE_WITH_KNOTS('',3,(#136777,#136778,#136779,#136780,
#136781,#136782,#136783,#136784,#136785,#136786,#136787,#136788,#136789,
#136790,#136791,#136792,#136793,#136794,#136795,#136796,#136797,#136798,
#136799,#136800,#136801,#136802,#136803,#136804,#136805,#136806,#136807,
#136808,#136809,#136810,#136811,#136812,#136813,#136814,#136815,#136816,
#136817,#136818,#136819,#136820,#136821,#136822,#136823,#136824,#136825,
#136826,#136827,#136828,#136829,#136830,#136831,#136832,#136833,#136834,
#136835,#136836,#136837,#136838,#136839,#136840,#136841,#136842,#136843,
#136844,#136845,#136846,#136847,#136848,#136849,#136850,#136851,#136852,
#136853,#136854,#136855,#136856,#136857,#136858),.UNSPECIFIED.,.F.,.F.,
(4,3,3,3,3,3,3,3,3,3,3,3,3,3,3,3,3,3,3,3,3,3,3,3,3,3,3,4),(0.,0.0151429849951974,
0.0309514432426294,0.0433468474135511,0.048016714296136,0.0521572447792291,
0.0684584883549305,0.0850611007943578,0.0963127192297611,0.100794579936147,
0.104383684737716,0.121455410665747,0.130067574535971,0.146660509203611,
0.155839714374814,0.15855153100884,0.17580325611013,0.19305498121142,0.204601414194011,
0.21094684716519,0.215063044140779,0.233049917075482,0.242953934795423,
0.247562215827255,0.25109595394491,0.269300903176924,0.272665987955243,
0.285115833302671),.UNSPECIFIED.);
#23563=B_SPLINE_CURVE_WITH_KNOTS('',3,(#136983,#136984,#136985,#136986,
#136987,#136988,#136989,#136990,#136991,#136992,#136993,#136994,#136995,
#136996,#136997,#136998,#136999,#137000,#137001,#137002,#137003,#137004,
#137005,#137006,#137007,#137008,#137009,#137010,#137011,#137012,#137013,
#137014,#137015,#137016,#137017,#137018,#137019,#137020,#137021,#137022,
#137023,#137024,#137025,#137026,#137027,#137028,#137029,#137030,#137031,
#137032,#137033,#137034,#137035,#137036,#137037,#137038,#137039,#137040,
#137041,#137042,#137043,#137044,#137045,#137046,#137047,#137048,#137049,
#137050,#137051,#137052,#137053,#137054,#137055,#137056,#137057,#137058,
#137059,#137060,#137061,#137062,#137063,#137064),.UNSPECIFIED.,.F.,.F.,
(4,3,3,3,3,3,3,3,3,3,3,3,3,3,3,3,3,3,3,3,3,3,3,3,3,3,3,4),(0.,0.0154790919518317,
0.0309581839036635,0.0433468577327002,0.0480167366668755,0.0521572427623293,
0.0686255280202576,0.0850611032056772,0.0963127210382473,0.100794583654536,
0.104383685901981,0.121455411399997,0.130067574535958,0.146660505573429,
0.155839706510775,0.158551519167426,0.175777335672888,0.193003152178349,
0.20460140499342,0.210946849266856,0.215063044035708,0.233049916749299,
0.242953934550777,0.247562210700648,0.251095948378327,0.26930089774997,
0.27266598795521,0.285115833656387),.UNSPECIFIED.);
#23564=B_SPLINE_CURVE_WITH_KNOTS('',3,(#137066,#137067,#137068,#137069),
 .UNSPECIFIED.,.F.,.F.,(4,4),(0.,0.00918599106546198),.UNSPECIFIED.);
#23565=B_SPLINE_CURVE_WITH_KNOTS('',3,(#137070,#137071,#137072,#137073,
#137074,#137075,#137076,#137077,#137078,#137079,#137080,#137081,#137082,
#137083,#137084,#137085,#137086,#137087,#137088,#137089,#137090,#137091,
#137092,#137093,#137094,#137095,#137096,#137097,#137098,#137099,#137100,
#137101,#137102,#137103,#137104,#137105,#137106,#137107,#137108,#137109,
#137110,#137111,#137112,#137113,#137114,#137115,#137116,#137117,#137118,
#137119,#137120,#137121,#137122,#137123,#137124,#137125,#137126,#137127,
#137128,#137129,#137130,#137131,#137132,#137133,#137134,#137135,#137136,
#137137,#137138,#137139,#137140,#137141,#137142,#137143,#137144,#137145),
 .UNSPECIFIED.,.F.,.F.,(4,3,3,3,3,3,3,3,3,3,3,3,3,3,3,3,3,3,3,3,3,3,3,3,
3,4),(0.,0.018046947694979,0.0362795627609177,0.049791457513174,0.0564440668188989,
0.0594975271731172,0.0772383217588031,0.0946647290647785,0.107092442188542,
0.114964949714838,0.11808807535994,0.134959936152474,0.144375581559832,
0.161646751661216,0.168625123295882,0.173118085365167,0.189917788602839,
0.206622922507054,0.223770964019213,0.227175695758215,0.243238311868422,
0.252063959651552,0.25594031760387,0.271478831695925,0.27594599330477,0.286347380332248),
 .UNSPECIFIED.);
#23566=B_SPLINE_CURVE_WITH_KNOTS('',3,(#137185,#137186,#137187,#137188),
 .UNSPECIFIED.,.F.,.F.,(4,4),(-1.89742724654025,-1.84562728381663),
 .UNSPECIFIED.);
#23567=B_SPLINE_CURVE_WITH_KNOTS('',3,(#137195,#137196,#137197,#137198),
 .UNSPECIFIED.,.F.,.F.,(4,4),(-1.94922720926386,-1.89742724654024),
 .UNSPECIFIED.);
#23568=B_SPLINE_CURVE_WITH_KNOTS('',3,(#137200,#137201,#137202,#137203),
 .UNSPECIFIED.,.F.,.F.,(4,4),(-1.89742724654023,-1.84562728381661),
 .UNSPECIFIED.);
#23569=B_SPLINE_CURVE_WITH_KNOTS('',3,(#137210,#137211,#137212,#137213),
 .UNSPECIFIED.,.F.,.F.,(4,4),(-1.94922720926387,-1.89742724654024),
 .UNSPECIFIED.);
#23570=B_SPLINE_CURVE_WITH_KNOTS('',3,(#137383,#137384,#137385,#137386,
#137387,#137388),.UNSPECIFIED.,.F.,.F.,(4,1,1,4),(0.,0.285714285714286,
0.571428571428571,1.),.UNSPECIFIED.);
#23571=B_SPLINE_CURVE_WITH_KNOTS('',3,(#137392,#137393,#137394,#137395,
#137396,#137397),.UNSPECIFIED.,.F.,.F.,(4,2,4),(0.,0.483208689475554,1.),
 .UNSPECIFIED.);
#23572=B_SPLINE_CURVE_WITH_KNOTS('',3,(#137405,#137406,#137407,#137408,
#137409,#137410),.UNSPECIFIED.,.F.,.F.,(4,1,1,4),(0.,0.285714285714286,
0.571428571428571,1.),.UNSPECIFIED.);
#23573=B_SPLINE_CURVE_WITH_KNOTS('',3,(#137414,#137415,#137416,#137417,
#137418,#137419),.UNSPECIFIED.,.F.,.F.,(4,2,4),(0.,0.483208689475554,1.),
 .UNSPECIFIED.);
#23574=B_SPLINE_CURVE_WITH_KNOTS('',3,(#137427,#137428,#137429,#137430,
#137431,#137432),.UNSPECIFIED.,.F.,.F.,(4,1,1,4),(0.,0.285714285714286,
0.571428571428571,1.),.UNSPECIFIED.);
#23575=B_SPLINE_CURVE_WITH_KNOTS('',3,(#137436,#137437,#137438,#137439,
#137440,#137441),.UNSPECIFIED.,.F.,.F.,(4,2,4),(0.,0.483208689475554,1.),
 .UNSPECIFIED.);
#23576=B_SPLINE_CURVE_WITH_KNOTS('',3,(#137449,#137450,#137451,#137452,
#137453,#137454),.UNSPECIFIED.,.F.,.F.,(4,1,1,4),(0.,0.285714285714286,
0.571428571428571,1.),.UNSPECIFIED.);
#23577=B_SPLINE_CURVE_WITH_KNOTS('',3,(#137458,#137459,#137460,#137461,
#137462,#137463),.UNSPECIFIED.,.F.,.F.,(4,2,4),(0.,0.483208689475554,1.),
 .UNSPECIFIED.);
#23578=B_SPLINE_CURVE_WITH_KNOTS('',3,(#137471,#137472,#137473,#137474,
#137475,#137476),.UNSPECIFIED.,.F.,.F.,(4,1,1,4),(0.,0.285714285714286,
0.571428571428571,1.),.UNSPECIFIED.);
#23579=B_SPLINE_CURVE_WITH_KNOTS('',3,(#137480,#137481,#137482,#137483,
#137484,#137485),.UNSPECIFIED.,.F.,.F.,(4,2,4),(0.,0.483208689475554,1.),
 .UNSPECIFIED.);
#23580=B_SPLINE_CURVE_WITH_KNOTS('',3,(#137493,#137494,#137495,#137496,
#137497,#137498),.UNSPECIFIED.,.F.,.F.,(4,1,1,4),(0.,0.285714285714286,
0.571428571428571,1.),.UNSPECIFIED.);
#23581=B_SPLINE_CURVE_WITH_KNOTS('',3,(#137502,#137503,#137504,#137505,
#137506,#137507),.UNSPECIFIED.,.F.,.F.,(4,2,4),(0.,0.483208689475554,1.),
 .UNSPECIFIED.);
#23582=B_SPLINE_CURVE_WITH_KNOTS('',3,(#137515,#137516,#137517,#137518,
#137519,#137520),.UNSPECIFIED.,.F.,.F.,(4,1,1,4),(0.,0.285714285714286,
0.571428571428571,1.),.UNSPECIFIED.);
#23583=B_SPLINE_CURVE_WITH_KNOTS('',3,(#137524,#137525,#137526,#137527,
#137528,#137529),.UNSPECIFIED.,.F.,.F.,(4,2,4),(0.,0.483208689475554,1.),
 .UNSPECIFIED.);
#23584=B_SPLINE_CURVE_WITH_KNOTS('',3,(#137537,#137538,#137539,#137540,
#137541,#137542),.UNSPECIFIED.,.F.,.F.,(4,1,1,4),(0.,0.285714285714286,
0.571428571428571,1.),.UNSPECIFIED.);
#23585=B_SPLINE_CURVE_WITH_KNOTS('',3,(#137546,#137547,#137548,#137549,
#137550,#137551),.UNSPECIFIED.,.F.,.F.,(4,2,4),(0.,0.483208689475554,1.),
 .UNSPECIFIED.);
#23586=B_SPLINE_CURVE_WITH_KNOTS('',3,(#137559,#137560,#137561,#137562,
#137563,#137564),.UNSPECIFIED.,.F.,.F.,(4,1,1,4),(0.,0.285714285714286,
0.571428571428571,1.),.UNSPECIFIED.);
#23587=B_SPLINE_CURVE_WITH_KNOTS('',3,(#137568,#137569,#137570,#137571,
#137572,#137573),.UNSPECIFIED.,.F.,.F.,(4,2,4),(0.,0.483208689475554,1.),
 .UNSPECIFIED.);
#23588=B_SPLINE_CURVE_WITH_KNOTS('',3,(#137581,#137582,#137583,#137584,
#137585,#137586),.UNSPECIFIED.,.F.,.F.,(4,1,1,4),(0.,0.285714285714286,
0.571428571428571,1.),.UNSPECIFIED.);
#23589=B_SPLINE_CURVE_WITH_KNOTS('',3,(#137590,#137591,#137592,#137593,
#137594,#137595),.UNSPECIFIED.,.F.,.F.,(4,2,4),(0.,0.483208689475554,1.),
 .UNSPECIFIED.);
#23590=B_SPLINE_CURVE_WITH_KNOTS('',3,(#137605,#137606,#137607,#137608,
#137609,#137610),.UNSPECIFIED.,.F.,.F.,(4,2,4),(0.,0.483208689475554,1.),
 .UNSPECIFIED.);
#23591=B_SPLINE_CURVE_WITH_KNOTS('',3,(#137614,#137615,#137616,#137617,
#137618,#137619),.UNSPECIFIED.,.F.,.F.,(4,1,1,4),(0.,0.285714285714286,
0.571428571428571,1.),.UNSPECIFIED.);
#23592=B_SPLINE_CURVE_WITH_KNOTS('',3,(#137627,#137628,#137629,#137630,
#137631,#137632),.UNSPECIFIED.,.F.,.F.,(4,2,4),(0.,0.483208689475554,1.),
 .UNSPECIFIED.);
#23593=B_SPLINE_CURVE_WITH_KNOTS('',3,(#137636,#137637,#137638,#137639,
#137640,#137641),.UNSPECIFIED.,.F.,.F.,(4,1,1,4),(0.,0.285714285714286,
0.571428571428571,1.),.UNSPECIFIED.);
#23594=B_SPLINE_CURVE_WITH_KNOTS('',3,(#137649,#137650,#137651,#137652,
#137653,#137654),.UNSPECIFIED.,.F.,.F.,(4,2,4),(0.,0.483208689475554,1.),
 .UNSPECIFIED.);
#23595=B_SPLINE_CURVE_WITH_KNOTS('',3,(#137658,#137659,#137660,#137661,
#137662,#137663),.UNSPECIFIED.,.F.,.F.,(4,1,1,4),(0.,0.285714285714286,
0.571428571428571,1.),.UNSPECIFIED.);
#23596=B_SPLINE_CURVE_WITH_KNOTS('',3,(#137671,#137672,#137673,#137674,
#137675,#137676),.UNSPECIFIED.,.F.,.F.,(4,2,4),(0.,0.483208689475554,1.),
 .UNSPECIFIED.);
#23597=B_SPLINE_CURVE_WITH_KNOTS('',3,(#137680,#137681,#137682,#137683,
#137684,#137685),.UNSPECIFIED.,.F.,.F.,(4,1,1,4),(0.,0.285714285714286,
0.571428571428571,1.),.UNSPECIFIED.);
#23598=B_SPLINE_CURVE_WITH_KNOTS('',3,(#137693,#137694,#137695,#137696,
#137697,#137698),.UNSPECIFIED.,.F.,.F.,(4,2,4),(0.,0.483208689475554,1.),
 .UNSPECIFIED.);
#23599=B_SPLINE_CURVE_WITH_KNOTS('',3,(#137702,#137703,#137704,#137705,
#137706,#137707),.UNSPECIFIED.,.F.,.F.,(4,1,1,4),(0.,0.285714285714286,
0.571428571428571,1.),.UNSPECIFIED.);
#23600=B_SPLINE_CURVE_WITH_KNOTS('',3,(#137715,#137716,#137717,#137718,
#137719,#137720),.UNSPECIFIED.,.F.,.F.,(4,2,4),(0.,0.483208689475554,1.),
 .UNSPECIFIED.);
#23601=B_SPLINE_CURVE_WITH_KNOTS('',3,(#137724,#137725,#137726,#137727,
#137728,#137729),.UNSPECIFIED.,.F.,.F.,(4,1,1,4),(0.,0.285714285714286,
0.571428571428571,1.),.UNSPECIFIED.);
#23602=B_SPLINE_CURVE_WITH_KNOTS('',3,(#137737,#137738,#137739,#137740,
#137741,#137742),.UNSPECIFIED.,.F.,.F.,(4,2,4),(0.,0.483208689475554,1.),
 .UNSPECIFIED.);
#23603=B_SPLINE_CURVE_WITH_KNOTS('',3,(#137746,#137747,#137748,#137749,
#137750,#137751),.UNSPECIFIED.,.F.,.F.,(4,1,1,4),(0.,0.285714285714286,
0.571428571428571,1.),.UNSPECIFIED.);
#23604=B_SPLINE_CURVE_WITH_KNOTS('',3,(#137759,#137760,#137761,#137762,
#137763,#137764),.UNSPECIFIED.,.F.,.F.,(4,2,4),(0.,0.483208689475554,1.),
 .UNSPECIFIED.);
#23605=B_SPLINE_CURVE_WITH_KNOTS('',3,(#137768,#137769,#137770,#137771,
#137772,#137773),.UNSPECIFIED.,.F.,.F.,(4,1,1,4),(0.,0.285714285714286,
0.571428571428571,1.),.UNSPECIFIED.);
#23606=B_SPLINE_CURVE_WITH_KNOTS('',3,(#137781,#137782,#137783,#137784,
#137785,#137786),.UNSPECIFIED.,.F.,.F.,(4,2,4),(0.,0.483208689475554,1.),
 .UNSPECIFIED.);
#23607=B_SPLINE_CURVE_WITH_KNOTS('',3,(#137790,#137791,#137792,#137793,
#137794,#137795),.UNSPECIFIED.,.F.,.F.,(4,1,1,4),(0.,0.285714285714286,
0.571428571428571,1.),.UNSPECIFIED.);
#23608=B_SPLINE_CURVE_WITH_KNOTS('',3,(#137803,#137804,#137805,#137806,
#137807,#137808),.UNSPECIFIED.,.F.,.F.,(4,2,4),(0.,0.483208689475554,1.),
 .UNSPECIFIED.);
#23609=B_SPLINE_CURVE_WITH_KNOTS('',3,(#137812,#137813,#137814,#137815,
#137816,#137817),.UNSPECIFIED.,.F.,.F.,(4,1,1,4),(0.,0.285714285714286,
0.571428571428571,1.),.UNSPECIFIED.);
#27047=LINE('',#130725,#30849);
#27048=LINE('',#130906,#30850);
#27049=LINE('',#131282,#30851);
#27050=LINE('',#131640,#30852);
#27051=LINE('',#131813,#30853);
#27052=LINE('',#131996,#30854);
#27053=LINE('',#132368,#30855);
#27054=LINE('',#132726,#30856);
#27055=LINE('',#132897,#30857);
#27056=LINE('',#133014,#30858);
#27057=LINE('',#133308,#30859);
#27058=LINE('',#133661,#30860);
#27059=LINE('',#133852,#30861);
#27060=LINE('',#133971,#30862);
#27061=LINE('',#134267,#30863);
#27062=LINE('',#134620,#30864);
#27063=LINE('',#136631,#30865);
#27064=LINE('',#136635,#30866);
#27065=LINE('',#137151,#30867);
#27066=LINE('',#137155,#30868);
#27067=LINE('',#137165,#30869);
#27068=LINE('',#137169,#30870);
#27069=LINE('',#137179,#30871);
#27070=LINE('',#137183,#30872);
#27071=LINE('',#137190,#30873);
#27072=LINE('',#137194,#30874);
#27073=LINE('',#137205,#30875);
#27074=LINE('',#137209,#30876);
#27075=LINE('',#137222,#30877);
#27076=LINE('',#137228,#30878);
#27077=LINE('',#137236,#30879);
#27078=LINE('',#137243,#30880);
#27079=LINE('',#137246,#30881);
#27080=LINE('',#137249,#30882);
#27081=LINE('',#137253,#30883);
#27082=LINE('',#137254,#30884);
#27083=LINE('',#137257,#30885);
#27084=LINE('',#137261,#30886);
#27085=LINE('',#137262,#30887);
#27086=LINE('',#137267,#30888);
#27087=LINE('',#137271,#30889);
#27088=LINE('',#137272,#30890);
#27089=LINE('',#137275,#30891);
#27090=LINE('',#137279,#30892);
#27091=LINE('',#137280,#30893);
#27092=LINE('',#137286,#30894);
#27093=LINE('',#137288,#30895);
#27094=LINE('',#137290,#30896);
#27095=LINE('',#137291,#30897);
#27096=LINE('',#137295,#30898);
#27097=LINE('',#137301,#30899);
#27098=LINE('',#137302,#30900);
#27099=LINE('',#137303,#30901);
#27100=LINE('',#137306,#30902);
#27101=LINE('',#137311,#30903);
#27102=LINE('',#137316,#30904);
#27103=LINE('',#137321,#30905);
#27104=LINE('',#137323,#30906);
#27105=LINE('',#137324,#30907);
#27106=LINE('',#137328,#30908);
#27107=LINE('',#137333,#30909);
#27108=LINE('',#137335,#30910);
#27109=LINE('',#137336,#30911);
#27110=LINE('',#137339,#30912);
#27111=LINE('',#137344,#30913);
#27112=LINE('',#137350,#30914);
#27113=LINE('',#137351,#30915);
#27114=LINE('',#137353,#30916);
#27115=LINE('',#137356,#30917);
#27116=LINE('',#137358,#30918);
#27117=LINE('',#137361,#30919);
#27118=LINE('',#137363,#30920);
#27119=LINE('',#137365,#30921);
#27120=LINE('',#137370,#30922);
#27121=LINE('',#137374,#30923);
#27122=LINE('',#137381,#30924);
#27123=LINE('',#137399,#30925);
#27124=LINE('',#137403,#30926);
#27125=LINE('',#137421,#30927);
#27126=LINE('',#137425,#30928);
#27127=LINE('',#137443,#30929);
#27128=LINE('',#137447,#30930);
#27129=LINE('',#137465,#30931);
#27130=LINE('',#137469,#30932);
#27131=LINE('',#137487,#30933);
#27132=LINE('',#137491,#30934);
#27133=LINE('',#137509,#30935);
#27134=LINE('',#137513,#30936);
#27135=LINE('',#137531,#30937);
#27136=LINE('',#137535,#30938);
#27137=LINE('',#137553,#30939);
#27138=LINE('',#137557,#30940);
#27139=LINE('',#137575,#30941);
#27140=LINE('',#137579,#30942);
#27141=LINE('',#137596,#30943);
#27142=LINE('',#137603,#30944);
#27143=LINE('',#137621,#30945);
#27144=LINE('',#137625,#30946);
#27145=LINE('',#137643,#30947);
#27146=LINE('',#137647,#30948);
#27147=LINE('',#137665,#30949);
#27148=LINE('',#137669,#30950);
#27149=LINE('',#137687,#30951);
#27150=LINE('',#137691,#30952);
#27151=LINE('',#137709,#30953);
#27152=LINE('',#137713,#30954);
#27153=LINE('',#137731,#30955);
#27154=LINE('',#137735,#30956);
#27155=LINE('',#137753,#30957);
#27156=LINE('',#137757,#30958);
#27157=LINE('',#137775,#30959);
#27158=LINE('',#137779,#30960);
#27159=LINE('',#137797,#30961);
#27160=LINE('',#137801,#30962);
#27161=LINE('',#137818,#30963);
#27162=LINE('',#137822,#30964);
#27163=LINE('',#137823,#30965);
#27164=LINE('',#137836,#30966);
#27165=LINE('',#137838,#30967);
#27166=LINE('',#137851,#30968);
#27167=LINE('',#137853,#30969);
#27168=LINE('',#137855,#30970);
#27169=LINE('',#137857,#30971);
#27170=LINE('',#137859,#30972);
#27171=LINE('',#137860,#30973);
#27172=LINE('',#137873,#30974);
#27173=LINE('',#137875,#30975);
#27174=LINE('',#137888,#30976);
#27175=LINE('',#137891,#30977);
#27176=LINE('',#137893,#30978);
#27177=LINE('',#137894,#30979);
#27178=LINE('',#137907,#30980);
#27179=LINE('',#137909,#30981);
#27180=LINE('',#137922,#30982);
#27181=LINE('',#137925,#30983);
#27182=LINE('',#137927,#30984);
#27183=LINE('',#137928,#30985);
#27184=LINE('',#137941,#30986);
#27185=LINE('',#137943,#30987);
#27186=LINE('',#137956,#30988);
#27187=LINE('',#137959,#30989);
#27188=LINE('',#137961,#30990);
#27189=LINE('',#137962,#30991);
#27190=LINE('',#137975,#30992);
#27191=LINE('',#137977,#30993);
#27192=LINE('',#137990,#30994);
#27193=LINE('',#137993,#30995);
#27194=LINE('',#137995,#30996);
#27195=LINE('',#137996,#30997);
#27196=LINE('',#138009,#30998);
#27197=LINE('',#138011,#30999);
#27198=LINE('',#138024,#31000);
#27199=LINE('',#138027,#31001);
#27200=LINE('',#138029,#31002);
#27201=LINE('',#138030,#31003);
#27202=LINE('',#138043,#31004);
#27203=LINE('',#138045,#31005);
#27204=LINE('',#138058,#31006);
#27205=LINE('',#138061,#31007);
#27206=LINE('',#138063,#31008);
#27207=LINE('',#138064,#31009);
#27208=LINE('',#138077,#31010);
#27209=LINE('',#138079,#31011);
#27210=LINE('',#138092,#31012);
#27211=LINE('',#138095,#31013);
#27212=LINE('',#138097,#31014);
#27213=LINE('',#138098,#31015);
#27214=LINE('',#138111,#31016);
#27215=LINE('',#138113,#31017);
#27216=LINE('',#138126,#31018);
#27217=LINE('',#138129,#31019);
#27218=LINE('',#138131,#31020);
#27219=LINE('',#138144,#31021);
#27220=LINE('',#138146,#31022);
#27221=LINE('',#138159,#31023);
#27222=LINE('',#138166,#31024);
#27223=LINE('',#138173,#31025);
#27224=LINE('',#138177,#31026);
#27225=LINE('',#138182,#31027);
#27226=LINE('',#138188,#31028);
#27227=LINE('',#138192,#31029);
#27228=LINE('',#138195,#31030);
#27229=LINE('',#138204,#31031);
#27230=LINE('',#138208,#31032);
#27231=LINE('',#138211,#31033);
#27232=LINE('',#138220,#31034);
#27233=LINE('',#138224,#31035);
#27234=LINE('',#138227,#31036);
#27235=LINE('',#138236,#31037);
#27236=LINE('',#138240,#31038);
#27237=LINE('',#138243,#31039);
#27238=LINE('',#138252,#31040);
#27239=LINE('',#138256,#31041);
#27240=LINE('',#138259,#31042);
#27241=LINE('',#138268,#31043);
#27242=LINE('',#138272,#31044);
#27243=LINE('',#138275,#31045);
#27244=LINE('',#138284,#31046);
#27245=LINE('',#138288,#31047);
#27246=LINE('',#138291,#31048);
#27247=LINE('',#138300,#31049);
#27248=LINE('',#138304,#31050);
#27249=LINE('',#138307,#31051);
#27250=LINE('',#138316,#31052);
#27251=LINE('',#138320,#31053);
#27252=LINE('',#138323,#31054);
#27253=LINE('',#138332,#31055);
#27254=LINE('',#138336,#31056);
#27255=LINE('',#138339,#31057);
#27256=LINE('',#138348,#31058);
#27257=LINE('',#138352,#31059);
#27258=LINE('',#138355,#31060);
#27259=LINE('',#138364,#31061);
#27260=LINE('',#138368,#31062);
#27261=LINE('',#138371,#31063);
#27262=LINE('',#138380,#31064);
#27263=LINE('',#138384,#31065);
#27264=LINE('',#138388,#31066);
#27265=LINE('',#138398,#31067);
#27266=LINE('',#138401,#31068);
#27267=LINE('',#138403,#31069);
#27268=LINE('',#138405,#31070);
#30849=VECTOR('',#105583,1.2645);
#30850=VECTOR('',#105588,1.2645);
#30851=VECTOR('',#105591,1.2645);
#30852=VECTOR('',#105594,1.2645);
#30853=VECTOR('',#105599,1.2645);
#30854=VECTOR('',#105604,1.2645);
#30855=VECTOR('',#105607,1.2645);
#30856=VECTOR('',#105610,1.2645);
#30857=VECTOR('',#105615,1.543);
#30858=VECTOR('',#105620,1.543);
#30859=VECTOR('',#105623,1.543);
#30860=VECTOR('',#105626,1.543);
#30861=VECTOR('',#105631,1.543);
#30862=VECTOR('',#105636,1.543);
#30863=VECTOR('',#105639,1.543);
#30864=VECTOR('',#105642,1.543);
#30865=VECTOR('',#105657,10.);
#30866=VECTOR('',#105660,10.);
#30867=VECTOR('',#105669,10.);
#30868=VECTOR('',#105672,10.);
#30869=VECTOR('',#105683,7.95);
#30870=VECTOR('',#105688,8.);
#30871=VECTOR('',#105699,18.2);
#30872=VECTOR('',#105706,18.25);
#30873=VECTOR('',#105707,10.);
#30874=VECTOR('',#105710,10.);
#30875=VECTOR('',#105711,10.);
#30876=VECTOR('',#105714,10.);
#30877=VECTOR('',#105723,18.2);
#30878=VECTOR('',#105732,18.25);
#30879=VECTOR('',#105741,2.55);
#30880=VECTOR('',#105750,2.5);
#30881=VECTOR('',#105755,18.2);
#30882=VECTOR('',#105758,10.);
#30883=VECTOR('',#105763,10.);
#30884=VECTOR('',#105764,10.);
#30885=VECTOR('',#105767,10.);
#30886=VECTOR('',#105772,10.);
#30887=VECTOR('',#105773,10.);
#30888=VECTOR('',#105780,10.);
#30889=VECTOR('',#105785,10.);
#30890=VECTOR('',#105786,10.);
#30891=VECTOR('',#105789,10.);
#30892=VECTOR('',#105794,10.);
#30893=VECTOR('',#105795,10.);
#30894=VECTOR('',#105802,10.);
#30895=VECTOR('',#105803,10.);
#30896=VECTOR('',#105804,10.);
#30897=VECTOR('',#105805,10.);
#30898=VECTOR('',#105808,10.);
#30899=VECTOR('',#105815,10.);
#30900=VECTOR('',#105816,10.);
#30901=VECTOR('',#105817,10.);
#30902=VECTOR('',#105820,10.);
#30903=VECTOR('',#105827,10.);
#30904=VECTOR('',#105832,10.);
#30905=VECTOR('',#105839,10.);
#30906=VECTOR('',#105840,10.);
#30907=VECTOR('',#105841,10.);
#30908=VECTOR('',#105844,10.);
#30909=VECTOR('',#105851,10.);
#30910=VECTOR('',#105852,10.);
#30911=VECTOR('',#105853,10.);
#30912=VECTOR('',#105856,10.);
#30913=VECTOR('',#105863,10.);
#30914=VECTOR('',#105874,10.);
#30915=VECTOR('',#105875,10.);
#30916=VECTOR('',#105878,10.);
#30917=VECTOR('',#105883,10.);
#30918=VECTOR('',#105886,10.);
#30919=VECTOR('',#105891,10.);
#30920=VECTOR('',#105894,10.);
#30921=VECTOR('',#105897,10.);
#30922=VECTOR('',#105902,1.15);
#30923=VECTOR('',#105907,1.);
#30924=VECTOR('',#105914,10.);
#30925=VECTOR('',#105917,10.);
#30926=VECTOR('',#105920,10.);
#30927=VECTOR('',#105923,10.);
#30928=VECTOR('',#105926,10.);
#30929=VECTOR('',#105929,10.);
#30930=VECTOR('',#105932,10.);
#30931=VECTOR('',#105935,10.);
#30932=VECTOR('',#105938,10.);
#30933=VECTOR('',#105941,10.);
#30934=VECTOR('',#105944,10.);
#30935=VECTOR('',#105947,10.);
#30936=VECTOR('',#105950,10.);
#30937=VECTOR('',#105953,10.);
#30938=VECTOR('',#105956,10.);
#30939=VECTOR('',#105959,10.);
#30940=VECTOR('',#105962,10.);
#30941=VECTOR('',#105965,10.);
#30942=VECTOR('',#105968,10.);
#30943=VECTOR('',#105971,10.);
#30944=VECTOR('',#105978,10.);
#30945=VECTOR('',#105981,10.);
#30946=VECTOR('',#105984,10.);
#30947=VECTOR('',#105987,10.);
#30948=VECTOR('',#105990,10.);
#30949=VECTOR('',#105993,10.);
#30950=VECTOR('',#105996,10.);
#30951=VECTOR('',#105999,10.);
#30952=VECTOR('',#106002,10.);
#30953=VECTOR('',#106005,10.);
#30954=VECTOR('',#106008,10.);
#30955=VECTOR('',#106011,10.);
#30956=VECTOR('',#106014,10.);
#30957=VECTOR('',#106017,10.);
#30958=VECTOR('',#106020,10.);
#30959=VECTOR('',#106023,10.);
#30960=VECTOR('',#106026,10.);
#30961=VECTOR('',#106029,10.);
#30962=VECTOR('',#106032,10.);
#30963=VECTOR('',#106035,10.);
#30964=VECTOR('',#106040,10.);
#30965=VECTOR('',#106041,10.);
#30966=VECTOR('',#106042,10.);
#30967=VECTOR('',#106045,10.);
#30968=VECTOR('',#106046,10.);
#30969=VECTOR('',#106049,10.);
#30970=VECTOR('',#106052,10.);
#30971=VECTOR('',#106055,10.);
#30972=VECTOR('',#106058,10.);
#30973=VECTOR('',#106059,10.);
#30974=VECTOR('',#106060,10.);
#30975=VECTOR('',#106063,10.);
#30976=VECTOR('',#106064,10.);
#30977=VECTOR('',#106069,10.);
#30978=VECTOR('',#106072,10.);
#30979=VECTOR('',#106073,10.);
#30980=VECTOR('',#106074,10.);
#30981=VECTOR('',#106077,10.);
#30982=VECTOR('',#106078,10.);
#30983=VECTOR('',#106083,10.);
#30984=VECTOR('',#106086,10.);
#30985=VECTOR('',#106087,10.);
#30986=VECTOR('',#106088,10.);
#30987=VECTOR('',#106091,10.);
#30988=VECTOR('',#106092,10.);
#30989=VECTOR('',#106097,10.);
#30990=VECTOR('',#106100,10.);
#30991=VECTOR('',#106101,10.);
#30992=VECTOR('',#106102,10.);
#30993=VECTOR('',#106105,10.);
#30994=VECTOR('',#106106,10.);
#30995=VECTOR('',#106111,10.);
#30996=VECTOR('',#106114,10.);
#30997=VECTOR('',#106115,10.);
#30998=VECTOR('',#106116,10.);
#30999=VECTOR('',#106119,10.);
#31000=VECTOR('',#106120,10.);
#31001=VECTOR('',#106125,10.);
#31002=VECTOR('',#106128,10.);
#31003=VECTOR('',#106129,10.);
#31004=VECTOR('',#106130,10.);
#31005=VECTOR('',#106133,10.);
#31006=VECTOR('',#106134,10.);
#31007=VECTOR('',#106139,10.);
#31008=VECTOR('',#106142,10.);
#31009=VECTOR('',#106143,10.);
#31010=VECTOR('',#106144,10.);
#31011=VECTOR('',#106147,10.);
#31012=VECTOR('',#106148,10.);
#31013=VECTOR('',#106153,10.);
#31014=VECTOR('',#106156,10.);
#31015=VECTOR('',#106157,10.);
#31016=VECTOR('',#106158,10.);
#31017=VECTOR('',#106161,10.);
#31018=VECTOR('',#106162,10.);
#31019=VECTOR('',#106167,10.);
#31020=VECTOR('',#106170,10.);
#31021=VECTOR('',#106171,10.);
#31022=VECTOR('',#106174,10.);
#31023=VECTOR('',#106175,10.);
#31024=VECTOR('',#106182,17.45);
#31025=VECTOR('',#106191,17.45);
#31026=VECTOR('',#106196,17.5);
#31027=VECTOR('',#106203,17.5);
#31028=VECTOR('',#106208,17.45);
#31029=VECTOR('',#106215,17.45);
#31030=VECTOR('',#106218,17.5);
#31031=VECTOR('',#106227,17.45);
#31032=VECTOR('',#106234,17.45);
#31033=VECTOR('',#106237,17.5);
#31034=VECTOR('',#106246,17.45);
#31035=VECTOR('',#106253,17.45);
#31036=VECTOR('',#106256,17.5);
#31037=VECTOR('',#106265,17.45);
#31038=VECTOR('',#106272,17.45);
#31039=VECTOR('',#106275,17.5);
#31040=VECTOR('',#106284,17.45);
#31041=VECTOR('',#106291,17.45);
#31042=VECTOR('',#106294,17.5);
#31043=VECTOR('',#106303,17.45);
#31044=VECTOR('',#106310,17.45);
#31045=VECTOR('',#106313,17.5);
#31046=VECTOR('',#106322,17.45);
#31047=VECTOR('',#106329,17.45);
#31048=VECTOR('',#106332,17.5);
#31049=VECTOR('',#106341,17.45);
#31050=VECTOR('',#106348,17.45);
#31051=VECTOR('',#106351,17.5);
#31052=VECTOR('',#106360,17.45);
#31053=VECTOR('',#106367,17.45);
#31054=VECTOR('',#106370,17.5);
#31055=VECTOR('',#106379,17.45);
#31056=VECTOR('',#106386,17.45);
#31057=VECTOR('',#106389,17.5);
#31058=VECTOR('',#106398,17.45);
#31059=VECTOR('',#106405,17.45);
#31060=VECTOR('',#106408,17.5);
#31061=VECTOR('',#106417,17.45);
#31062=VECTOR('',#106424,17.45);
#31063=VECTOR('',#106427,17.5);
#31064=VECTOR('',#106436,17.45);
#31065=VECTOR('',#106443,17.45);
#31066=VECTOR('',#106448,17.5);
#31067=VECTOR('',#106459,17.45);
#31068=VECTOR('',#106464,17.45);
#31069=VECTOR('',#106467,17.5);
#31070=VECTOR('',#106470,1.5);
#34651=VERTEX_POINT('',#130723);
#34652=VERTEX_POINT('',#130724);
#34653=VERTEX_POINT('',#130726);
#34654=VERTEX_POINT('',#130794);
#34655=VERTEX_POINT('',#130817);
#34656=VERTEX_POINT('',#130904);
#34657=VERTEX_POINT('',#130905);
#34658=VERTEX_POINT('',#130907);
#34659=VERTEX_POINT('',#131280);
#34660=VERTEX_POINT('',#131281);
#34661=VERTEX_POINT('',#131283);
#34662=VERTEX_POINT('',#131638);
#34663=VERTEX_POINT('',#131639);
#34664=VERTEX_POINT('',#131641);
#34665=VERTEX_POINT('',#131684);
#34666=VERTEX_POINT('',#131811);
#34667=VERTEX_POINT('',#131812);
#34668=VERTEX_POINT('',#131814);
#34669=VERTEX_POINT('',#131882);
#34670=VERTEX_POINT('',#131905);
#34671=VERTEX_POINT('',#131994);
#34672=VERTEX_POINT('',#131995);
#34673=VERTEX_POINT('',#131997);
#34674=VERTEX_POINT('',#132366);
#34675=VERTEX_POINT('',#132367);
#34676=VERTEX_POINT('',#132369);
#34677=VERTEX_POINT('',#132724);
#34678=VERTEX_POINT('',#132725);
#34679=VERTEX_POINT('',#132727);
#34680=VERTEX_POINT('',#132768);
#34681=VERTEX_POINT('',#132895);
#34682=VERTEX_POINT('',#132896);
#34683=VERTEX_POINT('',#132898);
#34684=VERTEX_POINT('',#132951);
#34685=VERTEX_POINT('',#133012);
#34686=VERTEX_POINT('',#133013);
#34687=VERTEX_POINT('',#133015);
#34688=VERTEX_POINT('',#133158);
#34689=VERTEX_POINT('',#133306);
#34690=VERTEX_POINT('',#133307);
#34691=VERTEX_POINT('',#133309);
#34692=VERTEX_POINT('',#133509);
#34693=VERTEX_POINT('',#133659);
#34694=VERTEX_POINT('',#133660);
#34695=VERTEX_POINT('',#133662);
#34696=VERTEX_POINT('',#133717);
#34697=VERTEX_POINT('',#133755);
#34698=VERTEX_POINT('',#133850);
#34699=VERTEX_POINT('',#133851);
#34700=VERTEX_POINT('',#133853);
#34701=VERTEX_POINT('',#133906);
#34702=VERTEX_POINT('',#133969);
#34703=VERTEX_POINT('',#133970);
#34704=VERTEX_POINT('',#133972);
#34705=VERTEX_POINT('',#134117);
#34706=VERTEX_POINT('',#134265);
#34707=VERTEX_POINT('',#134266);
#34708=VERTEX_POINT('',#134268);
#34709=VERTEX_POINT('',#134468);
#34710=VERTEX_POINT('',#134618);
#34711=VERTEX_POINT('',#134619);
#34712=VERTEX_POINT('',#134621);
#34713=VERTEX_POINT('',#134676);
#34714=VERTEX_POINT('',#134714);
#34715=VERTEX_POINT('',#135387);
#34716=VERTEX_POINT('',#135752);
#34717=VERTEX_POINT('',#136542);
#34718=VERTEX_POINT('',#136627);
#34719=VERTEX_POINT('',#136628);
#34720=VERTEX_POINT('',#136630);
#34721=VERTEX_POINT('',#136632);
#34722=VERTEX_POINT('',#136634);
#34723=VERTEX_POINT('',#136636);
#34724=VERTEX_POINT('',#137065);
#34725=VERTEX_POINT('',#137147);
#34726=VERTEX_POINT('',#137148);
#34727=VERTEX_POINT('',#137150);
#34728=VERTEX_POINT('',#137152);
#34729=VERTEX_POINT('',#137154);
#34730=VERTEX_POINT('',#137156);
#34731=VERTEX_POINT('',#137158);
#34732=VERTEX_POINT('',#137162);
#34733=VERTEX_POINT('',#137164);
#34734=VERTEX_POINT('',#137168);
#34735=VERTEX_POINT('',#137172);
#34736=VERTEX_POINT('',#137175);
#34737=VERTEX_POINT('',#137176);
#34738=VERTEX_POINT('',#137178);
#34739=VERTEX_POINT('',#137184);
#34740=VERTEX_POINT('',#137189);
#34741=VERTEX_POINT('',#137191);
#34742=VERTEX_POINT('',#137193);
#34743=VERTEX_POINT('',#137199);
#34744=VERTEX_POINT('',#137204);
#34745=VERTEX_POINT('',#137206);
#34746=VERTEX_POINT('',#137208);
#34747=VERTEX_POINT('',#137215);
#34748=VERTEX_POINT('',#137218);
#34749=VERTEX_POINT('',#137219);
#34750=VERTEX_POINT('',#137221);
#34751=VERTEX_POINT('',#137226);
#34752=VERTEX_POINT('',#137230);
#34753=VERTEX_POINT('',#137233);
#34754=VERTEX_POINT('',#137235);
#34755=VERTEX_POINT('',#137239);
#34756=VERTEX_POINT('',#137242);
#34757=VERTEX_POINT('',#137248);
#34758=VERTEX_POINT('',#137252);
#34759=VERTEX_POINT('',#137256);
#34760=VERTEX_POINT('',#137260);
#34761=VERTEX_POINT('',#137266);
#34762=VERTEX_POINT('',#137270);
#34763=VERTEX_POINT('',#137274);
#34764=VERTEX_POINT('',#137278);
#34765=VERTEX_POINT('',#137284);
#34766=VERTEX_POINT('',#137285);
#34767=VERTEX_POINT('',#137287);
#34768=VERTEX_POINT('',#137289);
#34769=VERTEX_POINT('',#137293);
#34770=VERTEX_POINT('',#137294);
#34771=VERTEX_POINT('',#137299);
#34772=VERTEX_POINT('',#137300);
#34773=VERTEX_POINT('',#137305);
#34774=VERTEX_POINT('',#137310);
#34775=VERTEX_POINT('',#137314);
#34776=VERTEX_POINT('',#137315);
#34777=VERTEX_POINT('',#137320);
#34778=VERTEX_POINT('',#137322);
#34779=VERTEX_POINT('',#137326);
#34780=VERTEX_POINT('',#137327);
#34781=VERTEX_POINT('',#137332);
#34782=VERTEX_POINT('',#137334);
#34783=VERTEX_POINT('',#137338);
#34784=VERTEX_POINT('',#137343);
#34785=VERTEX_POINT('',#137367);
#34786=VERTEX_POINT('',#137369);
#34787=VERTEX_POINT('',#137373);
#34788=VERTEX_POINT('',#137377);
#34789=VERTEX_POINT('',#137378);
#34790=VERTEX_POINT('',#137380);
#34791=VERTEX_POINT('',#137382);
#34792=VERTEX_POINT('',#137389);
#34793=VERTEX_POINT('',#137391);
#34794=VERTEX_POINT('',#137398);
#34795=VERTEX_POINT('',#137400);
#34796=VERTEX_POINT('',#137402);
#34797=VERTEX_POINT('',#137404);
#34798=VERTEX_POINT('',#137411);
#34799=VERTEX_POINT('',#137413);
#34800=VERTEX_POINT('',#137420);
#34801=VERTEX_POINT('',#137422);
#34802=VERTEX_POINT('',#137424);
#34803=VERTEX_POINT('',#137426);
#34804=VERTEX_POINT('',#137433);
#34805=VERTEX_POINT('',#137435);
#34806=VERTEX_POINT('',#137442);
#34807=VERTEX_POINT('',#137444);
#34808=VERTEX_POINT('',#137446);
#34809=VERTEX_POINT('',#137448);
#34810=VERTEX_POINT('',#137455);
#34811=VERTEX_POINT('',#137457);
#34812=VERTEX_POINT('',#137464);
#34813=VERTEX_POINT('',#137466);
#34814=VERTEX_POINT('',#137468);
#34815=VERTEX_POINT('',#137470);
#34816=VERTEX_POINT('',#137477);
#34817=VERTEX_POINT('',#137479);
#34818=VERTEX_POINT('',#137486);
#34819=VERTEX_POINT('',#137488);
#34820=VERTEX_POINT('',#137490);
#34821=VERTEX_POINT('',#137492);
#34822=VERTEX_POINT('',#137499);
#34823=VERTEX_POINT('',#137501);
#34824=VERTEX_POINT('',#137508);
#34825=VERTEX_POINT('',#137510);
#34826=VERTEX_POINT('',#137512);
#34827=VERTEX_POINT('',#137514);
#34828=VERTEX_POINT('',#137521);
#34829=VERTEX_POINT('',#137523);
#34830=VERTEX_POINT('',#137530);
#34831=VERTEX_POINT('',#137532);
#34832=VERTEX_POINT('',#137534);
#34833=VERTEX_POINT('',#137536);
#34834=VERTEX_POINT('',#137543);
#34835=VERTEX_POINT('',#137545);
#34836=VERTEX_POINT('',#137552);
#34837=VERTEX_POINT('',#137554);
#34838=VERTEX_POINT('',#137556);
#34839=VERTEX_POINT('',#137558);
#34840=VERTEX_POINT('',#137565);
#34841=VERTEX_POINT('',#137567);
#34842=VERTEX_POINT('',#137574);
#34843=VERTEX_POINT('',#137576);
#34844=VERTEX_POINT('',#137578);
#34845=VERTEX_POINT('',#137580);
#34846=VERTEX_POINT('',#137587);
#34847=VERTEX_POINT('',#137589);
#34848=VERTEX_POINT('',#137599);
#34849=VERTEX_POINT('',#137600);
#34850=VERTEX_POINT('',#137602);
#34851=VERTEX_POINT('',#137604);
#34852=VERTEX_POINT('',#137611);
#34853=VERTEX_POINT('',#137613);
#34854=VERTEX_POINT('',#137620);
#34855=VERTEX_POINT('',#137622);
#34856=VERTEX_POINT('',#137624);
#34857=VERTEX_POINT('',#137626);
#34858=VERTEX_POINT('',#137633);
#34859=VERTEX_POINT('',#137635);
#34860=VERTEX_POINT('',#137642);
#34861=VERTEX_POINT('',#137644);
#34862=VERTEX_POINT('',#137646);
#34863=VERTEX_POINT('',#137648);
#34864=VERTEX_POINT('',#137655);
#34865=VERTEX_POINT('',#137657);
#34866=VERTEX_POINT('',#137664);
#34867=VERTEX_POINT('',#137666);
#34868=VERTEX_POINT('',#137668);
#34869=VERTEX_POINT('',#137670);
#34870=VERTEX_POINT('',#137677);
#34871=VERTEX_POINT('',#137679);
#34872=VERTEX_POINT('',#137686);
#34873=VERTEX_POINT('',#137688);
#34874=VERTEX_POINT('',#137690);
#34875=VERTEX_POINT('',#137692);
#34876=VERTEX_POINT('',#137699);
#34877=VERTEX_POINT('',#137701);
#34878=VERTEX_POINT('',#137708);
#34879=VERTEX_POINT('',#137710);
#34880=VERTEX_POINT('',#137712);
#34881=VERTEX_POINT('',#137714);
#34882=VERTEX_POINT('',#137721);
#34883=VERTEX_POINT('',#137723);
#34884=VERTEX_POINT('',#137730);
#34885=VERTEX_POINT('',#137732);
#34886=VERTEX_POINT('',#137734);
#34887=VERTEX_POINT('',#137736);
#34888=VERTEX_POINT('',#137743);
#34889=VERTEX_POINT('',#137745);
#34890=VERTEX_POINT('',#137752);
#34891=VERTEX_POINT('',#137754);
#34892=VERTEX_POINT('',#137756);
#34893=VERTEX_POINT('',#137758);
#34894=VERTEX_POINT('',#137765);
#34895=VERTEX_POINT('',#137767);
#34896=VERTEX_POINT('',#137774);
#34897=VERTEX_POINT('',#137776);
#34898=VERTEX_POINT('',#137778);
#34899=VERTEX_POINT('',#137780);
#34900=VERTEX_POINT('',#137787);
#34901=VERTEX_POINT('',#137789);
#34902=VERTEX_POINT('',#137796);
#34903=VERTEX_POINT('',#137798);
#34904=VERTEX_POINT('',#137800);
#34905=VERTEX_POINT('',#137802);
#34906=VERTEX_POINT('',#137809);
#34907=VERTEX_POINT('',#137811);
#34908=VERTEX_POINT('',#137819);
#34909=VERTEX_POINT('',#138162);
#34910=VERTEX_POINT('',#138163);
#34911=VERTEX_POINT('',#138165);
#34912=VERTEX_POINT('',#138170);
#34913=VERTEX_POINT('',#138171);
#34914=VERTEX_POINT('',#138176);
#34915=VERTEX_POINT('',#138178);
#34916=VERTEX_POINT('',#138184);
#34917=VERTEX_POINT('',#138185);
#34918=VERTEX_POINT('',#138187);
#34919=VERTEX_POINT('',#138194);
#34920=VERTEX_POINT('',#138196);
#34921=VERTEX_POINT('',#138200);
#34922=VERTEX_POINT('',#138201);
#34923=VERTEX_POINT('',#138203);
#34924=VERTEX_POINT('',#138210);
#34925=VERTEX_POINT('',#138212);
#34926=VERTEX_POINT('',#138216);
#34927=VERTEX_POINT('',#138217);
#34928=VERTEX_POINT('',#138219);
#34929=VERTEX_POINT('',#138226);
#34930=VERTEX_POINT('',#138228);
#34931=VERTEX_POINT('',#138232);
#34932=VERTEX_POINT('',#138233);
#34933=VERTEX_POINT('',#138235);
#34934=VERTEX_POINT('',#138242);
#34935=VERTEX_POINT('',#138244);
#34936=VERTEX_POINT('',#138248);
#34937=VERTEX_POINT('',#138249);
#34938=VERTEX_POINT('',#138251);
#34939=VERTEX_POINT('',#138258);
#34940=VERTEX_POINT('',#138260);
#34941=VERTEX_POINT('',#138264);
#34942=VERTEX_POINT('',#138265);
#34943=VERTEX_POINT('',#138267);
#34944=VERTEX_POINT('',#138274);
#34945=VERTEX_POINT('',#138276);
#34946=VERTEX_POINT('',#138280);
#34947=VERTEX_POINT('',#138281);
#34948=VERTEX_POINT('',#138283);
#34949=VERTEX_POINT('',#138290);
#34950=VERTEX_POINT('',#138292);
#34951=VERTEX_POINT('',#138296);
#34952=VERTEX_POINT('',#138297);
#34953=VERTEX_POINT('',#138299);
#34954=VERTEX_POINT('',#138306);
#34955=VERTEX_POINT('',#138308);
#34956=VERTEX_POINT('',#138312);
#34957=VERTEX_POINT('',#138313);
#34958=VERTEX_POINT('',#138315);
#34959=VERTEX_POINT('',#138322);
#34960=VERTEX_POINT('',#138324);
#34961=VERTEX_POINT('',#138328);
#34962=VERTEX_POINT('',#138329);
#34963=VERTEX_POINT('',#138331);
#34964=VERTEX_POINT('',#138338);
#34965=VERTEX_POINT('',#138340);
#34966=VERTEX_POINT('',#138344);
#34967=VERTEX_POINT('',#138345);
#34968=VERTEX_POINT('',#138347);
#34969=VERTEX_POINT('',#138354);
#34970=VERTEX_POINT('',#138356);
#34971=VERTEX_POINT('',#138360);
#34972=VERTEX_POINT('',#138361);
#34973=VERTEX_POINT('',#138363);
#34974=VERTEX_POINT('',#138370);
#34975=VERTEX_POINT('',#138372);
#34976=VERTEX_POINT('',#138376);
#34977=VERTEX_POINT('',#138377);
#34978=VERTEX_POINT('',#138379);
#34979=VERTEX_POINT('',#138387);
#34980=VERTEX_POINT('',#138389);
#34981=VERTEX_POINT('',#138393);
#34982=VERTEX_POINT('',#138394);
#34983=VERTEX_POINT('',#138397);
#43516=EDGE_CURVE('',#34651,#34652,#27047,.T.);
#43517=EDGE_CURVE('',#34652,#34653,#23498,.T.);
#43518=EDGE_CURVE('',#34653,#34654,#23499,.T.);
#43519=EDGE_CURVE('',#34655,#34654,#18132,.F.);
#43520=EDGE_CURVE('',#34655,#34651,#23500,.T.);
#43521=EDGE_CURVE('',#34656,#34657,#27048,.T.);
#43522=EDGE_CURVE('',#34657,#34658,#23501,.T.);
#43523=EDGE_CURVE('',#34658,#34652,#23502,.T.);
#43524=EDGE_CURVE('',#34651,#34656,#23503,.T.);
#43525=EDGE_CURVE('',#34659,#34660,#27049,.T.);
#43526=EDGE_CURVE('',#34660,#34661,#23504,.T.);
#43527=EDGE_CURVE('',#34661,#34657,#23505,.T.);
#43528=EDGE_CURVE('',#34656,#34659,#23506,.T.);
#43529=EDGE_CURVE('',#34662,#34663,#27050,.T.);
#43530=EDGE_CURVE('',#34662,#34664,#23507,.T.);
#43531=EDGE_CURVE('',#34664,#34665,#18133,.F.);
#43532=EDGE_CURVE('',#34665,#34663,#23508,.T.);
#43533=EDGE_CURVE('',#34666,#34667,#27051,.T.);
#43534=EDGE_CURVE('',#34667,#34668,#23509,.T.);
#43535=EDGE_CURVE('',#34668,#34669,#23510,.T.);
#43536=EDGE_CURVE('',#34670,#34669,#18134,.F.);
#43537=EDGE_CURVE('',#34670,#34666,#23511,.T.);
#43538=EDGE_CURVE('',#34671,#34672,#27052,.T.);
#43539=EDGE_CURVE('',#34672,#34673,#23512,.T.);
#43540=EDGE_CURVE('',#34673,#34667,#23513,.T.);
#43541=EDGE_CURVE('',#34666,#34671,#23514,.T.);
#43542=EDGE_CURVE('',#34674,#34675,#27053,.T.);
#43543=EDGE_CURVE('',#34675,#34676,#23515,.T.);
#43544=EDGE_CURVE('',#34676,#34672,#23516,.T.);
#43545=EDGE_CURVE('',#34671,#34674,#23517,.T.);
#43546=EDGE_CURVE('',#34677,#34678,#27054,.T.);
#43547=EDGE_CURVE('',#34677,#34679,#23518,.T.);
#43548=EDGE_CURVE('',#34679,#34680,#18135,.F.);
#43549=EDGE_CURVE('',#34680,#34678,#23519,.T.);
#43550=EDGE_CURVE('',#34681,#34682,#27055,.T.);
#43551=EDGE_CURVE('',#34682,#34683,#23520,.T.);
#43552=EDGE_CURVE('',#34684,#34683,#18136,.T.);
#43553=EDGE_CURVE('',#34681,#34684,#23521,.F.);
#43554=EDGE_CURVE('',#34685,#34686,#27056,.T.);
#43555=EDGE_CURVE('',#34686,#34687,#23522,.T.);
#43556=EDGE_CURVE('',#34687,#34682,#23523,.T.);
#43557=EDGE_CURVE('',#34688,#34681,#23524,.F.);
#43558=EDGE_CURVE('',#34685,#34688,#23525,.F.);
#43559=EDGE_CURVE('',#34689,#34690,#27057,.T.);
#43560=EDGE_CURVE('',#34690,#34691,#23526,.T.);
#43561=EDGE_CURVE('',#34691,#34686,#23527,.T.);
#43562=EDGE_CURVE('',#34692,#34685,#23528,.F.);
#43563=EDGE_CURVE('',#34689,#34692,#23529,.F.);
#43564=EDGE_CURVE('',#34693,#34694,#27058,.T.);
#43565=EDGE_CURVE('',#34695,#34693,#23530,.F.);
#43566=EDGE_CURVE('',#34696,#34695,#23531,.T.);
#43567=EDGE_CURVE('',#34697,#34696,#18137,.T.);
#43568=EDGE_CURVE('',#34697,#34694,#23532,.T.);
#43569=EDGE_CURVE('',#34698,#34699,#27059,.T.);
#43570=EDGE_CURVE('',#34699,#34700,#23533,.T.);
#43571=EDGE_CURVE('',#34701,#34700,#18138,.T.);
#43572=EDGE_CURVE('',#34698,#34701,#23534,.F.);
#43573=EDGE_CURVE('',#34702,#34703,#27060,.T.);
#43574=EDGE_CURVE('',#34703,#34704,#23535,.T.);
#43575=EDGE_CURVE('',#34704,#34699,#23536,.T.);
#43576=EDGE_CURVE('',#34705,#34698,#23537,.F.);
#43577=EDGE_CURVE('',#34702,#34705,#23538,.F.);
#43578=EDGE_CURVE('',#34706,#34707,#27061,.T.);
#43579=EDGE_CURVE('',#34707,#34708,#23539,.T.);
#43580=EDGE_CURVE('',#34708,#34703,#23540,.T.);
#43581=EDGE_CURVE('',#34709,#34702,#23541,.F.);
#43582=EDGE_CURVE('',#34706,#34709,#23542,.F.);
#43583=EDGE_CURVE('',#34710,#34711,#27062,.T.);
#43584=EDGE_CURVE('',#34712,#34710,#23543,.F.);
#43585=EDGE_CURVE('',#34713,#34712,#23544,.T.);
#43586=EDGE_CURVE('',#34714,#34713,#18139,.T.);
#43587=EDGE_CURVE('',#34714,#34711,#23545,.T.);
#43588=EDGE_CURVE('',#34711,#34707,#23546,.T.);
#43589=EDGE_CURVE('',#34710,#34706,#23547,.F.);
#43590=EDGE_CURVE('',#34694,#34690,#23548,.T.);
#43591=EDGE_CURVE('',#34693,#34689,#23549,.F.);
#43592=EDGE_CURVE('',#34678,#34715,#23550,.T.);
#43593=EDGE_CURVE('',#34715,#34675,#23551,.T.);
#43594=EDGE_CURVE('',#34674,#34677,#23552,.T.);
#43595=EDGE_CURVE('',#34663,#34716,#23553,.T.);
#43596=EDGE_CURVE('',#34716,#34660,#23554,.T.);
#43597=EDGE_CURVE('',#34659,#34662,#23555,.T.);
#43598=EDGE_CURVE('',#34700,#34655,#23556,.T.);
#43599=EDGE_CURVE('',#34664,#34714,#23557,.T.);
#43600=EDGE_CURVE('',#34654,#34701,#23558,.T.);
#43601=EDGE_CURVE('',#34665,#34717,#23559,.T.);
#43602=EDGE_CURVE('',#34713,#34717,#23560,.T.);
#43603=EDGE_CURVE('',#34718,#34719,#18140,.T.);
#43604=EDGE_CURVE('',#34720,#34718,#27063,.T.);
#43605=EDGE_CURVE('',#34721,#34720,#18141,.T.);
#43606=EDGE_CURVE('',#34722,#34721,#27064,.T.);
#43607=EDGE_CURVE('',#34723,#34722,#18142,.T.);
#43608=EDGE_CURVE('',#34719,#34723,#18143,.T.);
#43609=EDGE_CURVE('',#34683,#34670,#23561,.T.);
#43610=EDGE_CURVE('',#34679,#34697,#23562,.T.);
#43611=EDGE_CURVE('',#34669,#34684,#23563,.T.);
#43612=EDGE_CURVE('',#34680,#34724,#23564,.T.);
#43613=EDGE_CURVE('',#34696,#34724,#23565,.T.);
#43614=EDGE_CURVE('',#34725,#34726,#18144,.T.);
#43615=EDGE_CURVE('',#34727,#34725,#27065,.T.);
#43616=EDGE_CURVE('',#34728,#34727,#18145,.T.);
#43617=EDGE_CURVE('',#34729,#34728,#27066,.T.);
#43618=EDGE_CURVE('',#34730,#34729,#18146,.T.);
#43619=EDGE_CURVE('',#34731,#34730,#18147,.T.);
#43620=EDGE_CURVE('',#34726,#34731,#18148,.T.);
#43621=EDGE_CURVE('',#34732,#34732,#18149,.T.);
#43622=EDGE_CURVE('',#34732,#34733,#27067,.T.);
#43623=EDGE_CURVE('',#34733,#34733,#18150,.T.);
#43624=EDGE_CURVE('',#34732,#34734,#27068,.T.);
#43625=EDGE_CURVE('',#34734,#34734,#18151,.T.);
#43626=EDGE_CURVE('',#34735,#34735,#18152,.T.);
#43627=EDGE_CURVE('',#34736,#34737,#18153,.T.);
#43628=EDGE_CURVE('',#34737,#34738,#27069,.T.);
#43629=EDGE_CURVE('',#34738,#34738,#18154,.T.);
#43630=EDGE_CURVE('',#34737,#34736,#18155,.T.);
#43631=EDGE_CURVE('',#34736,#34731,#27070,.T.);
#43632=EDGE_CURVE('',#34739,#34730,#23566,.T.);
#43633=EDGE_CURVE('',#34740,#34739,#27071,.T.);
#43634=EDGE_CURVE('',#34741,#34740,#18156,.T.);
#43635=EDGE_CURVE('',#34742,#34741,#27072,.T.);
#43636=EDGE_CURVE('',#34719,#34742,#23567,.T.);
#43637=EDGE_CURVE('',#34743,#34723,#23568,.T.);
#43638=EDGE_CURVE('',#34744,#34743,#27073,.T.);
#43639=EDGE_CURVE('',#34745,#34744,#18157,.T.);
#43640=EDGE_CURVE('',#34746,#34745,#27074,.T.);
#43641=EDGE_CURVE('',#34726,#34746,#23569,.T.);
#43642=EDGE_CURVE('',#34747,#34747,#18158,.T.);
#43643=EDGE_CURVE('',#34748,#34749,#18159,.T.);
#43644=EDGE_CURVE('',#34749,#34750,#27075,.T.);
#43645=EDGE_CURVE('',#34750,#34750,#18160,.T.);
#43646=EDGE_CURVE('',#34749,#34748,#18161,.T.);
#43647=EDGE_CURVE('',#34751,#34751,#18162,.T.);
#43648=EDGE_CURVE('',#34751,#34748,#27076,.T.);
#43649=EDGE_CURVE('',#34752,#34752,#18163,.T.);
#43650=EDGE_CURVE('',#34753,#34753,#18164,.T.);
#43651=EDGE_CURVE('',#34753,#34754,#27077,.T.);
#43652=EDGE_CURVE('',#34754,#34754,#18165,.T.);
#43653=EDGE_CURVE('',#34755,#34755,#18166,.T.);
#43654=EDGE_CURVE('',#34753,#34756,#27078,.T.);
#43655=EDGE_CURVE('',#34756,#34756,#18167,.T.);
#43656=EDGE_CURVE('',#34751,#34755,#27079,.T.);
#43657=EDGE_CURVE('',#34722,#34757,#27080,.T.);
#43658=EDGE_CURVE('',#34757,#34743,#18168,.T.);
#43659=EDGE_CURVE('',#34721,#34758,#27081,.T.);
#43660=EDGE_CURVE('',#34758,#34757,#27082,.T.);
#43661=EDGE_CURVE('',#34720,#34759,#27083,.T.);
#43662=EDGE_CURVE('',#34759,#34758,#18169,.T.);
#43663=EDGE_CURVE('',#34718,#34760,#27084,.T.);
#43664=EDGE_CURVE('',#34760,#34759,#27085,.T.);
#43665=EDGE_CURVE('',#34742,#34760,#18170,.T.);
#43666=EDGE_CURVE('',#34729,#34761,#27086,.T.);
#43667=EDGE_CURVE('',#34761,#34739,#18171,.T.);
#43668=EDGE_CURVE('',#34728,#34762,#27087,.T.);
#43669=EDGE_CURVE('',#34762,#34761,#27088,.T.);
#43670=EDGE_CURVE('',#34727,#34763,#27089,.T.);
#43671=EDGE_CURVE('',#34763,#34762,#18172,.T.);
#43672=EDGE_CURVE('',#34725,#34764,#27090,.T.);
#43673=EDGE_CURVE('',#34764,#34763,#27091,.T.);
#43674=EDGE_CURVE('',#34746,#34764,#18173,.T.);
#43675=EDGE_CURVE('',#34765,#34766,#27092,.T.);
#43676=EDGE_CURVE('',#34766,#34767,#27093,.T.);
#43677=EDGE_CURVE('',#34767,#34768,#27094,.T.);
#43678=EDGE_CURVE('',#34768,#34765,#27095,.T.);
#43679=EDGE_CURVE('',#34769,#34770,#27096,.T.);
#43680=EDGE_CURVE('',#34770,#34766,#18174,.T.);
#43681=EDGE_CURVE('',#34765,#34769,#18175,.T.);
#43682=EDGE_CURVE('',#34771,#34772,#27097,.T.);
#43683=EDGE_CURVE('',#34772,#34770,#27098,.T.);
#43684=EDGE_CURVE('',#34769,#34771,#27099,.T.);
#43685=EDGE_CURVE('',#34773,#34740,#27100,.T.);
#43686=EDGE_CURVE('',#34740,#34772,#18176,.T.);
#43687=EDGE_CURVE('',#34771,#34773,#18177,.T.);
#43688=EDGE_CURVE('',#34774,#34741,#27101,.T.);
#43689=EDGE_CURVE('',#34773,#34774,#18178,.T.);
#43690=EDGE_CURVE('',#34775,#34776,#27102,.T.);
#43691=EDGE_CURVE('',#34776,#34741,#18179,.T.);
#43692=EDGE_CURVE('',#34774,#34775,#18180,.T.);
#43693=EDGE_CURVE('',#34775,#34777,#27103,.T.);
#43694=EDGE_CURVE('',#34777,#34778,#27104,.T.);
#43695=EDGE_CURVE('',#34778,#34776,#27105,.T.);
#43696=EDGE_CURVE('',#34779,#34780,#27106,.T.);
#43697=EDGE_CURVE('',#34780,#34778,#18181,.T.);
#43698=EDGE_CURVE('',#34777,#34779,#18182,.T.);
#43699=EDGE_CURVE('',#34779,#34781,#27107,.T.);
#43700=EDGE_CURVE('',#34781,#34782,#27108,.T.);
#43701=EDGE_CURVE('',#34782,#34780,#27109,.T.);
#43702=EDGE_CURVE('',#34783,#34744,#27110,.T.);
#43703=EDGE_CURVE('',#34744,#34782,#18183,.T.);
#43704=EDGE_CURVE('',#34781,#34783,#18184,.T.);
#43705=EDGE_CURVE('',#34784,#34745,#27111,.T.);
#43706=EDGE_CURVE('',#34783,#34784,#18185,.T.);
#43707=EDGE_CURVE('',#34767,#34745,#18186,.T.);
#43708=EDGE_CURVE('',#34784,#34768,#18187,.T.);
#43709=EDGE_CURVE('',#34778,#34759,#27112,.T.);
#43710=EDGE_CURVE('',#34780,#34758,#27113,.T.);
#43711=EDGE_CURVE('',#34757,#34782,#27114,.T.);
#43712=EDGE_CURVE('',#34767,#34764,#27115,.T.);
#43713=EDGE_CURVE('',#34766,#34763,#27116,.T.);
#43714=EDGE_CURVE('',#34776,#34760,#27117,.T.);
#43715=EDGE_CURVE('',#34761,#34772,#27118,.T.);
#43716=EDGE_CURVE('',#34770,#34762,#27119,.T.);
#43717=EDGE_CURVE('',#34785,#34785,#18188,.T.);
#43718=EDGE_CURVE('',#34785,#34786,#27120,.T.);
#43719=EDGE_CURVE('',#34786,#34786,#18189,.T.);
#43720=EDGE_CURVE('',#34785,#34787,#27121,.T.);
#43721=EDGE_CURVE('',#34787,#34787,#18190,.T.);
#43722=EDGE_CURVE('',#34788,#34789,#18191,.T.);
#43723=EDGE_CURVE('',#34789,#34790,#27122,.T.);
#43724=EDGE_CURVE('',#34790,#34791,#23570,.T.);
#43725=EDGE_CURVE('',#34792,#34791,#18192,.T.);
#43726=EDGE_CURVE('',#34792,#34793,#23571,.T.);
#43727=EDGE_CURVE('',#34793,#34794,#27123,.T.);
#43728=EDGE_CURVE('',#34794,#34795,#18193,.T.);
#43729=EDGE_CURVE('',#34795,#34796,#27124,.T.);
#43730=EDGE_CURVE('',#34796,#34797,#23572,.T.);
#43731=EDGE_CURVE('',#34798,#34797,#18194,.T.);
#43732=EDGE_CURVE('',#34798,#34799,#23573,.T.);
#43733=EDGE_CURVE('',#34799,#34800,#27125,.T.);
#43734=EDGE_CURVE('',#34800,#34801,#18195,.T.);
#43735=EDGE_CURVE('',#34801,#34802,#27126,.T.);
#43736=EDGE_CURVE('',#34802,#34803,#23574,.T.);
#43737=EDGE_CURVE('',#34804,#34803,#18196,.T.);
#43738=EDGE_CURVE('',#34804,#34805,#23575,.T.);
#43739=EDGE_CURVE('',#34805,#34806,#27127,.T.);
#43740=EDGE_CURVE('',#34806,#34807,#18197,.T.);
#43741=EDGE_CURVE('',#34807,#34808,#27128,.T.);
#43742=EDGE_CURVE('',#34808,#34809,#23576,.T.);
#43743=EDGE_CURVE('',#34810,#34809,#18198,.T.);
#43744=EDGE_CURVE('',#34810,#34811,#23577,.T.);
#43745=EDGE_CURVE('',#34811,#34812,#27129,.T.);
#43746=EDGE_CURVE('',#34812,#34813,#18199,.T.);
#43747=EDGE_CURVE('',#34813,#34814,#27130,.T.);
#43748=EDGE_CURVE('',#34814,#34815,#23578,.T.);
#43749=EDGE_CURVE('',#34816,#34815,#18200,.T.);
#43750=EDGE_CURVE('',#34816,#34817,#23579,.T.);
#43751=EDGE_CURVE('',#34817,#34818,#27131,.T.);
#43752=EDGE_CURVE('',#34818,#34819,#18201,.T.);
#43753=EDGE_CURVE('',#34819,#34820,#27132,.T.);
#43754=EDGE_CURVE('',#34820,#34821,#23580,.T.);
#43755=EDGE_CURVE('',#34822,#34821,#18202,.T.);
#43756=EDGE_CURVE('',#34822,#34823,#23581,.T.);
#43757=EDGE_CURVE('',#34823,#34824,#27133,.T.);
#43758=EDGE_CURVE('',#34824,#34825,#18203,.T.);
#43759=EDGE_CURVE('',#34825,#34826,#27134,.T.);
#43760=EDGE_CURVE('',#34826,#34827,#23582,.T.);
#43761=EDGE_CURVE('',#34828,#34827,#18204,.T.);
#43762=EDGE_CURVE('',#34828,#34829,#23583,.T.);
#43763=EDGE_CURVE('',#34829,#34830,#27135,.T.);
#43764=EDGE_CURVE('',#34830,#34831,#18205,.T.);
#43765=EDGE_CURVE('',#34831,#34832,#27136,.T.);
#43766=EDGE_CURVE('',#34832,#34833,#23584,.T.);
#43767=EDGE_CURVE('',#34834,#34833,#18206,.T.);
#43768=EDGE_CURVE('',#34834,#34835,#23585,.T.);
#43769=EDGE_CURVE('',#34835,#34836,#27137,.T.);
#43770=EDGE_CURVE('',#34836,#34837,#18207,.T.);
#43771=EDGE_CURVE('',#34837,#34838,#27138,.T.);
#43772=EDGE_CURVE('',#34838,#34839,#23586,.T.);
#43773=EDGE_CURVE('',#34840,#34839,#18208,.T.);
#43774=EDGE_CURVE('',#34840,#34841,#23587,.T.);
#43775=EDGE_CURVE('',#34841,#34842,#27139,.T.);
#43776=EDGE_CURVE('',#34842,#34843,#18209,.T.);
#43777=EDGE_CURVE('',#34843,#34844,#27140,.T.);
#43778=EDGE_CURVE('',#34844,#34845,#23588,.T.);
#43779=EDGE_CURVE('',#34846,#34845,#18210,.T.);
#43780=EDGE_CURVE('',#34846,#34847,#23589,.T.);
#43781=EDGE_CURVE('',#34847,#34788,#27141,.T.);
#43782=EDGE_CURVE('',#34848,#34849,#18211,.T.);
#43783=EDGE_CURVE('',#34850,#34848,#27142,.T.);
#43784=EDGE_CURVE('',#34851,#34850,#23590,.T.);
#43785=EDGE_CURVE('',#34852,#34851,#18212,.T.);
#43786=EDGE_CURVE('',#34853,#34852,#23591,.T.);
#43787=EDGE_CURVE('',#34854,#34853,#27143,.T.);
#43788=EDGE_CURVE('',#34855,#34854,#18213,.T.);
#43789=EDGE_CURVE('',#34856,#34855,#27144,.T.);
#43790=EDGE_CURVE('',#34857,#34856,#23592,.T.);
#43791=EDGE_CURVE('',#34858,#34857,#18214,.T.);
#43792=EDGE_CURVE('',#34859,#34858,#23593,.T.);
#43793=EDGE_CURVE('',#34860,#34859,#27145,.T.);
#43794=EDGE_CURVE('',#34861,#34860,#18215,.T.);
#43795=EDGE_CURVE('',#34862,#34861,#27146,.T.);
#43796=EDGE_CURVE('',#34863,#34862,#23594,.T.);
#43797=EDGE_CURVE('',#34864,#34863,#18216,.T.);
#43798=EDGE_CURVE('',#34865,#34864,#23595,.T.);
#43799=EDGE_CURVE('',#34866,#34865,#27147,.T.);
#43800=EDGE_CURVE('',#34867,#34866,#18217,.T.);
#43801=EDGE_CURVE('',#34868,#34867,#27148,.T.);
#43802=EDGE_CURVE('',#34869,#34868,#23596,.T.);
#43803=EDGE_CURVE('',#34870,#34869,#18218,.T.);
#43804=EDGE_CURVE('',#34871,#34870,#23597,.T.);
#43805=EDGE_CURVE('',#34872,#34871,#27149,.T.);
#43806=EDGE_CURVE('',#34873,#34872,#18219,.T.);
#43807=EDGE_CURVE('',#34874,#34873,#27150,.T.);
#43808=EDGE_CURVE('',#34875,#34874,#23598,.T.);
#43809=EDGE_CURVE('',#34876,#34875,#18220,.T.);
#43810=EDGE_CURVE('',#34877,#34876,#23599,.T.);
#43811=EDGE_CURVE('',#34878,#34877,#27151,.T.);
#43812=EDGE_CURVE('',#34879,#34878,#18221,.T.);
#43813=EDGE_CURVE('',#34880,#34879,#27152,.T.);
#43814=EDGE_CURVE('',#34881,#34880,#23600,.T.);
#43815=EDGE_CURVE('',#34882,#34881,#18222,.T.);
#43816=EDGE_CURVE('',#34883,#34882,#23601,.T.);
#43817=EDGE_CURVE('',#34884,#34883,#27153,.T.);
#43818=EDGE_CURVE('',#34885,#34884,#18223,.T.);
#43819=EDGE_CURVE('',#34886,#34885,#27154,.T.);
#43820=EDGE_CURVE('',#34887,#34886,#23602,.T.);
#43821=EDGE_CURVE('',#34888,#34887,#18224,.T.);
#43822=EDGE_CURVE('',#34889,#34888,#23603,.T.);
#43823=EDGE_CURVE('',#34890,#34889,#27155,.T.);
#43824=EDGE_CURVE('',#34891,#34890,#18225,.T.);
#43825=EDGE_CURVE('',#34892,#34891,#27156,.T.);
#43826=EDGE_CURVE('',#34893,#34892,#23604,.T.);
#43827=EDGE_CURVE('',#34894,#34893,#18226,.T.);
#43828=EDGE_CURVE('',#34895,#34894,#23605,.T.);
#43829=EDGE_CURVE('',#34896,#34895,#27157,.T.);
#43830=EDGE_CURVE('',#34897,#34896,#18227,.T.);
#43831=EDGE_CURVE('',#34898,#34897,#27158,.T.);
#43832=EDGE_CURVE('',#34899,#34898,#23606,.T.);
#43833=EDGE_CURVE('',#34900,#34899,#18228,.T.);
#43834=EDGE_CURVE('',#34901,#34900,#23607,.T.);
#43835=EDGE_CURVE('',#34902,#34901,#27159,.T.);
#43836=EDGE_CURVE('',#34903,#34902,#18229,.T.);
#43837=EDGE_CURVE('',#34904,#34903,#27160,.T.);
#43838=EDGE_CURVE('',#34905,#34904,#23608,.T.);
#43839=EDGE_CURVE('',#34906,#34905,#18230,.T.);
#43840=EDGE_CURVE('',#34907,#34906,#23609,.T.);
#43841=EDGE_CURVE('',#34849,#34907,#27161,.T.);
#43842=EDGE_CURVE('',#34908,#34908,#18231,.T.);
#43843=EDGE_CURVE('',#34849,#34843,#27162,.T.);
#43844=EDGE_CURVE('',#34907,#34844,#27163,.T.);
#43845=EDGE_CURVE('',#34845,#34906,#27164,.T.);
#43846=EDGE_CURVE('',#34905,#34846,#27165,.T.);
#43847=EDGE_CURVE('',#34904,#34847,#27166,.T.);
#43848=EDGE_CURVE('',#34788,#34903,#27167,.T.);
#43849=EDGE_CURVE('',#34842,#34848,#27168,.T.);
#43850=EDGE_CURVE('',#34902,#34789,#27169,.T.);
#43851=EDGE_CURVE('',#34854,#34837,#27170,.T.);
#43852=EDGE_CURVE('',#34853,#34838,#27171,.T.);
#43853=EDGE_CURVE('',#34839,#34852,#27172,.T.);
#43854=EDGE_CURVE('',#34851,#34840,#27173,.T.);
#43855=EDGE_CURVE('',#34850,#34841,#27174,.T.);
#43856=EDGE_CURVE('',#34836,#34855,#27175,.T.);
#43857=EDGE_CURVE('',#34860,#34831,#27176,.T.);
#43858=EDGE_CURVE('',#34859,#34832,#27177,.T.);
#43859=EDGE_CURVE('',#34833,#34858,#27178,.T.);
#43860=EDGE_CURVE('',#34857,#34834,#27179,.T.);
#43861=EDGE_CURVE('',#34856,#34835,#27180,.T.);
#43862=EDGE_CURVE('',#34830,#34861,#27181,.T.);
#43863=EDGE_CURVE('',#34866,#34825,#27182,.T.);
#43864=EDGE_CURVE('',#34865,#34826,#27183,.T.);
#43865=EDGE_CURVE('',#34827,#34864,#27184,.T.);
#43866=EDGE_CURVE('',#34863,#34828,#27185,.T.);
#43867=EDGE_CURVE('',#34862,#34829,#27186,.T.);
#43868=EDGE_CURVE('',#34824,#34867,#27187,.T.);
#43869=EDGE_CURVE('',#34872,#34819,#27188,.T.);
#43870=EDGE_CURVE('',#34871,#34820,#27189,.T.);
#43871=EDGE_CURVE('',#34821,#34870,#27190,.T.);
#43872=EDGE_CURVE('',#34869,#34822,#27191,.T.);
#43873=EDGE_CURVE('',#34868,#34823,#27192,.T.);
#43874=EDGE_CURVE('',#34818,#34873,#27193,.T.);
#43875=EDGE_CURVE('',#34878,#34813,#27194,.T.);
#43876=EDGE_CURVE('',#34877,#34814,#27195,.T.);
#43877=EDGE_CURVE('',#34815,#34876,#27196,.T.);
#43878=EDGE_CURVE('',#34875,#34816,#27197,.T.);
#43879=EDGE_CURVE('',#34874,#34817,#27198,.T.);
#43880=EDGE_CURVE('',#34812,#34879,#27199,.T.);
#43881=EDGE_CURVE('',#34884,#34807,#27200,.T.);
#43882=EDGE_CURVE('',#34883,#34808,#27201,.T.);
#43883=EDGE_CURVE('',#34809,#34882,#27202,.T.);
#43884=EDGE_CURVE('',#34881,#34810,#27203,.T.);
#43885=EDGE_CURVE('',#34880,#34811,#27204,.T.);
#43886=EDGE_CURVE('',#34806,#34885,#27205,.T.);
#43887=EDGE_CURVE('',#34890,#34801,#27206,.T.);
#43888=EDGE_CURVE('',#34889,#34802,#27207,.T.);
#43889=EDGE_CURVE('',#34803,#34888,#27208,.T.);
#43890=EDGE_CURVE('',#34887,#34804,#27209,.T.);
#43891=EDGE_CURVE('',#34886,#34805,#27210,.T.);
#43892=EDGE_CURVE('',#34800,#34891,#27211,.T.);
#43893=EDGE_CURVE('',#34896,#34795,#27212,.T.);
#43894=EDGE_CURVE('',#34895,#34796,#27213,.T.);
#43895=EDGE_CURVE('',#34797,#34894,#27214,.T.);
#43896=EDGE_CURVE('',#34893,#34798,#27215,.T.);
#43897=EDGE_CURVE('',#34892,#34799,#27216,.T.);
#43898=EDGE_CURVE('',#34794,#34897,#27217,.T.);
#43899=EDGE_CURVE('',#34901,#34790,#27218,.T.);
#43900=EDGE_CURVE('',#34791,#34900,#27219,.T.);
#43901=EDGE_CURVE('',#34899,#34792,#27220,.T.);
#43902=EDGE_CURVE('',#34898,#34793,#27221,.T.);
#43903=EDGE_CURVE('',#34909,#34910,#18232,.T.);
#43904=EDGE_CURVE('',#34910,#34911,#27222,.T.);
#43905=EDGE_CURVE('',#34911,#34911,#18233,.T.);
#43906=EDGE_CURVE('',#34910,#34909,#18234,.T.);
#43907=EDGE_CURVE('',#34912,#34913,#18235,.T.);
#43908=EDGE_CURVE('',#34913,#34911,#27223,.T.);
#43909=EDGE_CURVE('',#34913,#34912,#18236,.T.);
#43910=EDGE_CURVE('',#34909,#34914,#27224,.T.);
#43911=EDGE_CURVE('',#34915,#34914,#18237,.T.);
#43912=EDGE_CURVE('',#34914,#34915,#18238,.T.);
#43913=EDGE_CURVE('',#34752,#34912,#27225,.T.);
#43914=EDGE_CURVE('',#34916,#34917,#18239,.T.);
#43915=EDGE_CURVE('',#34917,#34918,#27226,.T.);
#43916=EDGE_CURVE('',#34918,#34918,#18240,.T.);
#43917=EDGE_CURVE('',#34917,#34916,#18241,.T.);
#43918=EDGE_CURVE('',#34915,#34918,#27227,.T.);
#43919=EDGE_CURVE('',#34916,#34919,#27228,.T.);
#43920=EDGE_CURVE('',#34920,#34919,#18242,.T.);
#43921=EDGE_CURVE('',#34919,#34920,#18243,.T.);
#43922=EDGE_CURVE('',#34921,#34922,#18244,.T.);
#43923=EDGE_CURVE('',#34922,#34923,#27229,.T.);
#43924=EDGE_CURVE('',#34923,#34923,#18245,.T.);
#43925=EDGE_CURVE('',#34922,#34921,#18246,.T.);
#43926=EDGE_CURVE('',#34920,#34923,#27230,.T.);
#43927=EDGE_CURVE('',#34921,#34924,#27231,.T.);
#43928=EDGE_CURVE('',#34925,#34924,#18247,.T.);
#43929=EDGE_CURVE('',#34924,#34925,#18248,.T.);
#43930=EDGE_CURVE('',#34926,#34927,#18249,.T.);
#43931=EDGE_CURVE('',#34927,#34928,#27232,.T.);
#43932=EDGE_CURVE('',#34928,#34928,#18250,.T.);
#43933=EDGE_CURVE('',#34927,#34926,#18251,.T.);
#43934=EDGE_CURVE('',#34925,#34928,#27233,.T.);
#43935=EDGE_CURVE('',#34926,#34929,#27234,.T.);
#43936=EDGE_CURVE('',#34930,#34929,#18252,.T.);
#43937=EDGE_CURVE('',#34929,#34930,#18253,.T.);
#43938=EDGE_CURVE('',#34931,#34932,#18254,.T.);
#43939=EDGE_CURVE('',#34932,#34933,#27235,.T.);
#43940=EDGE_CURVE('',#34933,#34933,#18255,.T.);
#43941=EDGE_CURVE('',#34932,#34931,#18256,.T.);
#43942=EDGE_CURVE('',#34930,#34933,#27236,.T.);
#43943=EDGE_CURVE('',#34931,#34934,#27237,.T.);
#43944=EDGE_CURVE('',#34935,#34934,#18257,.T.);
#43945=EDGE_CURVE('',#34934,#34935,#18258,.T.);
#43946=EDGE_CURVE('',#34936,#34937,#18259,.T.);
#43947=EDGE_CURVE('',#34937,#34938,#27238,.T.);
#43948=EDGE_CURVE('',#34938,#34938,#18260,.T.);
#43949=EDGE_CURVE('',#34937,#34936,#18261,.T.);
#43950=EDGE_CURVE('',#34935,#34938,#27239,.T.);
#43951=EDGE_CURVE('',#34936,#34939,#27240,.T.);
#43952=EDGE_CURVE('',#34940,#34939,#18262,.T.);
#43953=EDGE_CURVE('',#34939,#34940,#18263,.T.);
#43954=EDGE_CURVE('',#34941,#34942,#18264,.T.);
#43955=EDGE_CURVE('',#34942,#34943,#27241,.T.);
#43956=EDGE_CURVE('',#34943,#34943,#18265,.T.);
#43957=EDGE_CURVE('',#34942,#34941,#18266,.T.);
#43958=EDGE_CURVE('',#34940,#34943,#27242,.T.);
#43959=EDGE_CURVE('',#34941,#34944,#27243,.T.);
#43960=EDGE_CURVE('',#34945,#34944,#18267,.T.);
#43961=EDGE_CURVE('',#34944,#34945,#18268,.T.);
#43962=EDGE_CURVE('',#34946,#34947,#18269,.T.);
#43963=EDGE_CURVE('',#34947,#34948,#27244,.T.);
#43964=EDGE_CURVE('',#34948,#34948,#18270,.T.);
#43965=EDGE_CURVE('',#34947,#34946,#18271,.T.);
#43966=EDGE_CURVE('',#34945,#34948,#27245,.T.);
#43967=EDGE_CURVE('',#34946,#34949,#27246,.T.);
#43968=EDGE_CURVE('',#34950,#34949,#18272,.T.);
#43969=EDGE_CURVE('',#34949,#34950,#18273,.T.);
#43970=EDGE_CURVE('',#34951,#34952,#18274,.T.);
#43971=EDGE_CURVE('',#34952,#34953,#27247,.T.);
#43972=EDGE_CURVE('',#34953,#34953,#18275,.T.);
#43973=EDGE_CURVE('',#34952,#34951,#18276,.T.);
#43974=EDGE_CURVE('',#34950,#34953,#27248,.T.);
#43975=EDGE_CURVE('',#34951,#34954,#27249,.T.);
#43976=EDGE_CURVE('',#34955,#34954,#18277,.T.);
#43977=EDGE_CURVE('',#34954,#34955,#18278,.T.);
#43978=EDGE_CURVE('',#34956,#34957,#18279,.T.);
#43979=EDGE_CURVE('',#34957,#34958,#27250,.T.);
#43980=EDGE_CURVE('',#34958,#34958,#18280,.T.);
#43981=EDGE_CURVE('',#34957,#34956,#18281,.T.);
#43982=EDGE_CURVE('',#34955,#34958,#27251,.T.);
#43983=EDGE_CURVE('',#34956,#34959,#27252,.T.);
#43984=EDGE_CURVE('',#34960,#34959,#18282,.T.);
#43985=EDGE_CURVE('',#34959,#34960,#18283,.T.);
#43986=EDGE_CURVE('',#34961,#34962,#18284,.T.);
#43987=EDGE_CURVE('',#34962,#34963,#27253,.T.);
#43988=EDGE_CURVE('',#34963,#34963,#18285,.T.);
#43989=EDGE_CURVE('',#34962,#34961,#18286,.T.);
#43990=EDGE_CURVE('',#34960,#34963,#27254,.T.);
#43991=EDGE_CURVE('',#34961,#34964,#27255,.T.);
#43992=EDGE_CURVE('',#34965,#34964,#18287,.T.);
#43993=EDGE_CURVE('',#34964,#34965,#18288,.T.);
#43994=EDGE_CURVE('',#34966,#34967,#18289,.T.);
#43995=EDGE_CURVE('',#34967,#34968,#27256,.T.);
#43996=EDGE_CURVE('',#34968,#34968,#18290,.T.);
#43997=EDGE_CURVE('',#34967,#34966,#18291,.T.);
#43998=EDGE_CURVE('',#34965,#34968,#27257,.T.);
#43999=EDGE_CURVE('',#34966,#34969,#27258,.T.);
#44000=EDGE_CURVE('',#34970,#34969,#18292,.T.);
#44001=EDGE_CURVE('',#34969,#34970,#18293,.T.);
#44002=EDGE_CURVE('',#34971,#34972,#18294,.T.);
#44003=EDGE_CURVE('',#34972,#34973,#27259,.T.);
#44004=EDGE_CURVE('',#34973,#34973,#18295,.T.);
#44005=EDGE_CURVE('',#34972,#34971,#18296,.T.);
#44006=EDGE_CURVE('',#34970,#34973,#27260,.T.);
#44007=EDGE_CURVE('',#34971,#34974,#27261,.T.);
#44008=EDGE_CURVE('',#34975,#34974,#18297,.T.);
#44009=EDGE_CURVE('',#34974,#34975,#18298,.T.);
#44010=EDGE_CURVE('',#34976,#34977,#18299,.T.);
#44011=EDGE_CURVE('',#34977,#34978,#27262,.T.);
#44012=EDGE_CURVE('',#34978,#34978,#18300,.T.);
#44013=EDGE_CURVE('',#34977,#34976,#18301,.T.);
#44014=EDGE_CURVE('',#34975,#34978,#27263,.T.);
#44015=EDGE_CURVE('',#34976,#34979,#27264,.T.);
#44016=EDGE_CURVE('',#34979,#34980,#18302,.T.);
#44017=EDGE_CURVE('',#34980,#34979,#18303,.T.);
#44018=EDGE_CURVE('',#34981,#34982,#18304,.T.);
#44019=EDGE_CURVE('',#34982,#34981,#18305,.T.);
#44020=EDGE_CURVE('',#34982,#34983,#27265,.T.);
#44021=EDGE_CURVE('',#34983,#34983,#18306,.T.);
#44022=EDGE_CURVE('',#34980,#34983,#27266,.T.);
#44023=EDGE_CURVE('',#34981,#34747,#27267,.T.);
#44024=EDGE_CURVE('',#34735,#34908,#27268,.T.);
#58028=ORIENTED_EDGE('',*,*,#43516,.T.);
#58029=ORIENTED_EDGE('',*,*,#43517,.T.);
#58030=ORIENTED_EDGE('',*,*,#43518,.T.);
#58031=ORIENTED_EDGE('',*,*,#43519,.F.);
#58032=ORIENTED_EDGE('',*,*,#43520,.T.);
#58033=ORIENTED_EDGE('',*,*,#43521,.T.);
#58034=ORIENTED_EDGE('',*,*,#43522,.T.);
#58035=ORIENTED_EDGE('',*,*,#43523,.T.);
#58036=ORIENTED_EDGE('',*,*,#43516,.F.);
#58037=ORIENTED_EDGE('',*,*,#43524,.T.);
#58038=ORIENTED_EDGE('',*,*,#43525,.T.);
#58039=ORIENTED_EDGE('',*,*,#43526,.T.);
#58040=ORIENTED_EDGE('',*,*,#43527,.T.);
#58041=ORIENTED_EDGE('',*,*,#43521,.F.);
#58042=ORIENTED_EDGE('',*,*,#43528,.T.);
#58043=ORIENTED_EDGE('',*,*,#43529,.F.);
#58044=ORIENTED_EDGE('',*,*,#43530,.T.);
#58045=ORIENTED_EDGE('',*,*,#43531,.T.);
#58046=ORIENTED_EDGE('',*,*,#43532,.T.);
#58047=ORIENTED_EDGE('',*,*,#43533,.T.);
#58048=ORIENTED_EDGE('',*,*,#43534,.T.);
#58049=ORIENTED_EDGE('',*,*,#43535,.T.);
#58050=ORIENTED_EDGE('',*,*,#43536,.F.);
#58051=ORIENTED_EDGE('',*,*,#43537,.T.);
#58052=ORIENTED_EDGE('',*,*,#43538,.T.);
#58053=ORIENTED_EDGE('',*,*,#43539,.T.);
#58054=ORIENTED_EDGE('',*,*,#43540,.T.);
#58055=ORIENTED_EDGE('',*,*,#43533,.F.);
#58056=ORIENTED_EDGE('',*,*,#43541,.T.);
#58057=ORIENTED_EDGE('',*,*,#43542,.T.);
#58058=ORIENTED_EDGE('',*,*,#43543,.T.);
#58059=ORIENTED_EDGE('',*,*,#43544,.T.);
#58060=ORIENTED_EDGE('',*,*,#43538,.F.);
#58061=ORIENTED_EDGE('',*,*,#43545,.T.);
#58062=ORIENTED_EDGE('',*,*,#43546,.F.);
#58063=ORIENTED_EDGE('',*,*,#43547,.T.);
#58064=ORIENTED_EDGE('',*,*,#43548,.T.);
#58065=ORIENTED_EDGE('',*,*,#43549,.T.);
#58066=ORIENTED_EDGE('',*,*,#43550,.T.);
#58067=ORIENTED_EDGE('',*,*,#43551,.T.);
#58068=ORIENTED_EDGE('',*,*,#43552,.F.);
#58069=ORIENTED_EDGE('',*,*,#43553,.F.);
#58070=ORIENTED_EDGE('',*,*,#43554,.T.);
#58071=ORIENTED_EDGE('',*,*,#43555,.T.);
#58072=ORIENTED_EDGE('',*,*,#43556,.T.);
#58073=ORIENTED_EDGE('',*,*,#43550,.F.);
#58074=ORIENTED_EDGE('',*,*,#43557,.F.);
#58075=ORIENTED_EDGE('',*,*,#43558,.F.);
#58076=ORIENTED_EDGE('',*,*,#43559,.T.);
#58077=ORIENTED_EDGE('',*,*,#43560,.T.);
#58078=ORIENTED_EDGE('',*,*,#43561,.T.);
#58079=ORIENTED_EDGE('',*,*,#43554,.F.);
#58080=ORIENTED_EDGE('',*,*,#43562,.F.);
#58081=ORIENTED_EDGE('',*,*,#43563,.F.);
#58082=ORIENTED_EDGE('',*,*,#43564,.F.);
#58083=ORIENTED_EDGE('',*,*,#43565,.F.);
#58084=ORIENTED_EDGE('',*,*,#43566,.F.);
#58085=ORIENTED_EDGE('',*,*,#43567,.F.);
#58086=ORIENTED_EDGE('',*,*,#43568,.T.);
#58087=ORIENTED_EDGE('',*,*,#43569,.T.);
#58088=ORIENTED_EDGE('',*,*,#43570,.T.);
#58089=ORIENTED_EDGE('',*,*,#43571,.F.);
#58090=ORIENTED_EDGE('',*,*,#43572,.F.);
#58091=ORIENTED_EDGE('',*,*,#43573,.T.);
#58092=ORIENTED_EDGE('',*,*,#43574,.T.);
#58093=ORIENTED_EDGE('',*,*,#43575,.T.);
#58094=ORIENTED_EDGE('',*,*,#43569,.F.);
#58095=ORIENTED_EDGE('',*,*,#43576,.F.);
#58096=ORIENTED_EDGE('',*,*,#43577,.F.);
#58097=ORIENTED_EDGE('',*,*,#43578,.T.);
#58098=ORIENTED_EDGE('',*,*,#43579,.T.);
#58099=ORIENTED_EDGE('',*,*,#43580,.T.);
#58100=ORIENTED_EDGE('',*,*,#43573,.F.);
#58101=ORIENTED_EDGE('',*,*,#43581,.F.);
#58102=ORIENTED_EDGE('',*,*,#43582,.F.);
#58103=ORIENTED_EDGE('',*,*,#43583,.F.);
#58104=ORIENTED_EDGE('',*,*,#43584,.F.);
#58105=ORIENTED_EDGE('',*,*,#43585,.F.);
#58106=ORIENTED_EDGE('',*,*,#43586,.F.);
#58107=ORIENTED_EDGE('',*,*,#43587,.T.);
#58108=ORIENTED_EDGE('',*,*,#43583,.T.);
#58109=ORIENTED_EDGE('',*,*,#43588,.T.);
#58110=ORIENTED_EDGE('',*,*,#43578,.F.);
#58111=ORIENTED_EDGE('',*,*,#43589,.F.);
#58112=ORIENTED_EDGE('',*,*,#43564,.T.);
#58113=ORIENTED_EDGE('',*,*,#43590,.T.);
#58114=ORIENTED_EDGE('',*,*,#43559,.F.);
#58115=ORIENTED_EDGE('',*,*,#43591,.F.);
#58116=ORIENTED_EDGE('',*,*,#43546,.T.);
#58117=ORIENTED_EDGE('',*,*,#43592,.T.);
#58118=ORIENTED_EDGE('',*,*,#43593,.T.);
#58119=ORIENTED_EDGE('',*,*,#43542,.F.);
#58120=ORIENTED_EDGE('',*,*,#43594,.T.);
#58121=ORIENTED_EDGE('',*,*,#43529,.T.);
#58122=ORIENTED_EDGE('',*,*,#43595,.T.);
#58123=ORIENTED_EDGE('',*,*,#43596,.T.);
#58124=ORIENTED_EDGE('',*,*,#43525,.F.);
#58125=ORIENTED_EDGE('',*,*,#43597,.T.);
#58126=ORIENTED_EDGE('',*,*,#43598,.F.);
#58127=ORIENTED_EDGE('',*,*,#43570,.F.);
#58128=ORIENTED_EDGE('',*,*,#43575,.F.);
#58129=ORIENTED_EDGE('',*,*,#43574,.F.);
#58130=ORIENTED_EDGE('',*,*,#43580,.F.);
#58131=ORIENTED_EDGE('',*,*,#43579,.F.);
#58132=ORIENTED_EDGE('',*,*,#43588,.F.);
#58133=ORIENTED_EDGE('',*,*,#43587,.F.);
#58134=ORIENTED_EDGE('',*,*,#43599,.F.);
#58135=ORIENTED_EDGE('',*,*,#43530,.F.);
#58136=ORIENTED_EDGE('',*,*,#43597,.F.);
#58137=ORIENTED_EDGE('',*,*,#43528,.F.);
#58138=ORIENTED_EDGE('',*,*,#43524,.F.);
#58139=ORIENTED_EDGE('',*,*,#43520,.F.);
#58140=ORIENTED_EDGE('',*,*,#43600,.F.);
#58141=ORIENTED_EDGE('',*,*,#43518,.F.);
#58142=ORIENTED_EDGE('',*,*,#43517,.F.);
#58143=ORIENTED_EDGE('',*,*,#43523,.F.);
#58144=ORIENTED_EDGE('',*,*,#43522,.F.);
#58145=ORIENTED_EDGE('',*,*,#43527,.F.);
#58146=ORIENTED_EDGE('',*,*,#43526,.F.);
#58147=ORIENTED_EDGE('',*,*,#43596,.F.);
#58148=ORIENTED_EDGE('',*,*,#43595,.F.);
#58149=ORIENTED_EDGE('',*,*,#43532,.F.);
#58150=ORIENTED_EDGE('',*,*,#43601,.T.);
#58151=ORIENTED_EDGE('',*,*,#43602,.F.);
#58152=ORIENTED_EDGE('',*,*,#43585,.T.);
#58153=ORIENTED_EDGE('',*,*,#43584,.T.);
#58154=ORIENTED_EDGE('',*,*,#43589,.T.);
#58155=ORIENTED_EDGE('',*,*,#43582,.T.);
#58156=ORIENTED_EDGE('',*,*,#43581,.T.);
#58157=ORIENTED_EDGE('',*,*,#43577,.T.);
#58158=ORIENTED_EDGE('',*,*,#43576,.T.);
#58159=ORIENTED_EDGE('',*,*,#43572,.T.);
#58160=ORIENTED_EDGE('',*,*,#43603,.F.);
#58161=ORIENTED_EDGE('',*,*,#43604,.F.);
#58162=ORIENTED_EDGE('',*,*,#43605,.F.);
#58163=ORIENTED_EDGE('',*,*,#43606,.F.);
#58164=ORIENTED_EDGE('',*,*,#43607,.F.);
#58165=ORIENTED_EDGE('',*,*,#43608,.F.);
#58166=ORIENTED_EDGE('',*,*,#43600,.T.);
#58167=ORIENTED_EDGE('',*,*,#43571,.T.);
#58168=ORIENTED_EDGE('',*,*,#43598,.T.);
#58169=ORIENTED_EDGE('',*,*,#43519,.T.);
#58170=ORIENTED_EDGE('',*,*,#43609,.F.);
#58171=ORIENTED_EDGE('',*,*,#43551,.F.);
#58172=ORIENTED_EDGE('',*,*,#43556,.F.);
#58173=ORIENTED_EDGE('',*,*,#43555,.F.);
#58174=ORIENTED_EDGE('',*,*,#43561,.F.);
#58175=ORIENTED_EDGE('',*,*,#43560,.F.);
#58176=ORIENTED_EDGE('',*,*,#43590,.F.);
#58177=ORIENTED_EDGE('',*,*,#43568,.F.);
#58178=ORIENTED_EDGE('',*,*,#43610,.F.);
#58179=ORIENTED_EDGE('',*,*,#43547,.F.);
#58180=ORIENTED_EDGE('',*,*,#43594,.F.);
#58181=ORIENTED_EDGE('',*,*,#43545,.F.);
#58182=ORIENTED_EDGE('',*,*,#43541,.F.);
#58183=ORIENTED_EDGE('',*,*,#43537,.F.);
#58184=ORIENTED_EDGE('',*,*,#43611,.F.);
#58185=ORIENTED_EDGE('',*,*,#43535,.F.);
#58186=ORIENTED_EDGE('',*,*,#43534,.F.);
#58187=ORIENTED_EDGE('',*,*,#43540,.F.);
#58188=ORIENTED_EDGE('',*,*,#43539,.F.);
#58189=ORIENTED_EDGE('',*,*,#43544,.F.);
#58190=ORIENTED_EDGE('',*,*,#43543,.F.);
#58191=ORIENTED_EDGE('',*,*,#43593,.F.);
#58192=ORIENTED_EDGE('',*,*,#43592,.F.);
#58193=ORIENTED_EDGE('',*,*,#43549,.F.);
#58194=ORIENTED_EDGE('',*,*,#43612,.T.);
#58195=ORIENTED_EDGE('',*,*,#43613,.F.);
#58196=ORIENTED_EDGE('',*,*,#43566,.T.);
#58197=ORIENTED_EDGE('',*,*,#43565,.T.);
#58198=ORIENTED_EDGE('',*,*,#43591,.T.);
#58199=ORIENTED_EDGE('',*,*,#43563,.T.);
#58200=ORIENTED_EDGE('',*,*,#43562,.T.);
#58201=ORIENTED_EDGE('',*,*,#43558,.T.);
#58202=ORIENTED_EDGE('',*,*,#43557,.T.);
#58203=ORIENTED_EDGE('',*,*,#43553,.T.);
#58204=ORIENTED_EDGE('',*,*,#43614,.F.);
#58205=ORIENTED_EDGE('',*,*,#43615,.F.);
#58206=ORIENTED_EDGE('',*,*,#43616,.F.);
#58207=ORIENTED_EDGE('',*,*,#43617,.F.);
#58208=ORIENTED_EDGE('',*,*,#43618,.F.);
#58209=ORIENTED_EDGE('',*,*,#43619,.F.);
#58210=ORIENTED_EDGE('',*,*,#43620,.F.);
#58211=ORIENTED_EDGE('',*,*,#43611,.T.);
#58212=ORIENTED_EDGE('',*,*,#43552,.T.);
#58213=ORIENTED_EDGE('',*,*,#43609,.T.);
#58214=ORIENTED_EDGE('',*,*,#43536,.T.);
#58215=ORIENTED_EDGE('',*,*,#43621,.T.);
#58216=ORIENTED_EDGE('',*,*,#43622,.T.);
#58217=ORIENTED_EDGE('',*,*,#43623,.T.);
#58218=ORIENTED_EDGE('',*,*,#43622,.F.);
#58219=ORIENTED_EDGE('',*,*,#43621,.F.);
#58220=ORIENTED_EDGE('',*,*,#43624,.T.);
#58221=ORIENTED_EDGE('',*,*,#43625,.F.);
#58222=ORIENTED_EDGE('',*,*,#43624,.F.);
#58223=ORIENTED_EDGE('',*,*,#43623,.F.);
#58224=ORIENTED_EDGE('',*,*,#43626,.T.);
#58225=ORIENTED_EDGE('',*,*,#43627,.T.);
#58226=ORIENTED_EDGE('',*,*,#43628,.T.);
#58227=ORIENTED_EDGE('',*,*,#43629,.T.);
#58228=ORIENTED_EDGE('',*,*,#43628,.F.);
#58229=ORIENTED_EDGE('',*,*,#43630,.T.);
#58230=ORIENTED_EDGE('',*,*,#43627,.F.);
#58231=ORIENTED_EDGE('',*,*,#43631,.T.);
#58232=ORIENTED_EDGE('',*,*,#43619,.T.);
#58233=ORIENTED_EDGE('',*,*,#43632,.F.);
#58234=ORIENTED_EDGE('',*,*,#43633,.F.);
#58235=ORIENTED_EDGE('',*,*,#43634,.F.);
#58236=ORIENTED_EDGE('',*,*,#43635,.F.);
#58237=ORIENTED_EDGE('',*,*,#43636,.F.);
#58238=ORIENTED_EDGE('',*,*,#43608,.T.);
#58239=ORIENTED_EDGE('',*,*,#43637,.F.);
#58240=ORIENTED_EDGE('',*,*,#43638,.F.);
#58241=ORIENTED_EDGE('',*,*,#43639,.F.);
#58242=ORIENTED_EDGE('',*,*,#43640,.F.);
#58243=ORIENTED_EDGE('',*,*,#43641,.F.);
#58244=ORIENTED_EDGE('',*,*,#43620,.T.);
#58245=ORIENTED_EDGE('',*,*,#43631,.F.);
#58246=ORIENTED_EDGE('',*,*,#43630,.F.);
#58247=ORIENTED_EDGE('',*,*,#43629,.F.);
#58248=ORIENTED_EDGE('',*,*,#43642,.F.);
#58249=ORIENTED_EDGE('',*,*,#43643,.T.);
#58250=ORIENTED_EDGE('',*,*,#43644,.T.);
#58251=ORIENTED_EDGE('',*,*,#43645,.T.);
#58252=ORIENTED_EDGE('',*,*,#43644,.F.);
#58253=ORIENTED_EDGE('',*,*,#43646,.T.);
#58254=ORIENTED_EDGE('',*,*,#43647,.F.);
#58255=ORIENTED_EDGE('',*,*,#43648,.T.);
#58256=ORIENTED_EDGE('',*,*,#43646,.F.);
#58257=ORIENTED_EDGE('',*,*,#43643,.F.);
#58258=ORIENTED_EDGE('',*,*,#43648,.F.);
#58259=ORIENTED_EDGE('',*,*,#43645,.F.);
#58260=ORIENTED_EDGE('',*,*,#43649,.F.);
#58261=ORIENTED_EDGE('',*,*,#43650,.T.);
#58262=ORIENTED_EDGE('',*,*,#43651,.T.);
#58263=ORIENTED_EDGE('',*,*,#43652,.T.);
#58264=ORIENTED_EDGE('',*,*,#43651,.F.);
#58265=ORIENTED_EDGE('',*,*,#43653,.F.);
#58266=ORIENTED_EDGE('',*,*,#43652,.F.);
#58267=ORIENTED_EDGE('',*,*,#43650,.F.);
#58268=ORIENTED_EDGE('',*,*,#43654,.T.);
#58269=ORIENTED_EDGE('',*,*,#43655,.T.);
#58270=ORIENTED_EDGE('',*,*,#43654,.F.);
#58271=ORIENTED_EDGE('',*,*,#43647,.T.);
#58272=ORIENTED_EDGE('',*,*,#43656,.T.);
#58273=ORIENTED_EDGE('',*,*,#43653,.T.);
#58274=ORIENTED_EDGE('',*,*,#43656,.F.);
#58275=ORIENTED_EDGE('',*,*,#43637,.T.);
#58276=ORIENTED_EDGE('',*,*,#43607,.T.);
#58277=ORIENTED_EDGE('',*,*,#43657,.T.);
#58278=ORIENTED_EDGE('',*,*,#43658,.T.);
#58279=ORIENTED_EDGE('',*,*,#43657,.F.);
#58280=ORIENTED_EDGE('',*,*,#43606,.T.);
#58281=ORIENTED_EDGE('',*,*,#43659,.T.);
#58282=ORIENTED_EDGE('',*,*,#43660,.T.);
#58283=ORIENTED_EDGE('',*,*,#43659,.F.);
#58284=ORIENTED_EDGE('',*,*,#43605,.T.);
#58285=ORIENTED_EDGE('',*,*,#43661,.T.);
#58286=ORIENTED_EDGE('',*,*,#43662,.T.);
#58287=ORIENTED_EDGE('',*,*,#43661,.F.);
#58288=ORIENTED_EDGE('',*,*,#43604,.T.);
#58289=ORIENTED_EDGE('',*,*,#43663,.T.);
#58290=ORIENTED_EDGE('',*,*,#43664,.T.);
#58291=ORIENTED_EDGE('',*,*,#43636,.T.);
#58292=ORIENTED_EDGE('',*,*,#43665,.T.);
#58293=ORIENTED_EDGE('',*,*,#43663,.F.);
#58294=ORIENTED_EDGE('',*,*,#43603,.T.);
#58295=ORIENTED_EDGE('',*,*,#43632,.T.);
#58296=ORIENTED_EDGE('',*,*,#43618,.T.);
#58297=ORIENTED_EDGE('',*,*,#43666,.T.);
#58298=ORIENTED_EDGE('',*,*,#43667,.T.);
#58299=ORIENTED_EDGE('',*,*,#43666,.F.);
#58300=ORIENTED_EDGE('',*,*,#43617,.T.);
#58301=ORIENTED_EDGE('',*,*,#43668,.T.);
#58302=ORIENTED_EDGE('',*,*,#43669,.T.);
#58303=ORIENTED_EDGE('',*,*,#43668,.F.);
#58304=ORIENTED_EDGE('',*,*,#43616,.T.);
#58305=ORIENTED_EDGE('',*,*,#43670,.T.);
#58306=ORIENTED_EDGE('',*,*,#43671,.T.);
#58307=ORIENTED_EDGE('',*,*,#43670,.F.);
#58308=ORIENTED_EDGE('',*,*,#43615,.T.);
#58309=ORIENTED_EDGE('',*,*,#43672,.T.);
#58310=ORIENTED_EDGE('',*,*,#43673,.T.);
#58311=ORIENTED_EDGE('',*,*,#43641,.T.);
#58312=ORIENTED_EDGE('',*,*,#43674,.T.);
#58313=ORIENTED_EDGE('',*,*,#43672,.F.);
#58314=ORIENTED_EDGE('',*,*,#43614,.T.);
#58315=ORIENTED_EDGE('',*,*,#43675,.T.);
#58316=ORIENTED_EDGE('',*,*,#43676,.T.);
#58317=ORIENTED_EDGE('',*,*,#43677,.T.);
#58318=ORIENTED_EDGE('',*,*,#43678,.T.);
#58319=ORIENTED_EDGE('',*,*,#43679,.T.);
#58320=ORIENTED_EDGE('',*,*,#43680,.T.);
#58321=ORIENTED_EDGE('',*,*,#43675,.F.);
#58322=ORIENTED_EDGE('',*,*,#43681,.T.);
#58323=ORIENTED_EDGE('',*,*,#43682,.T.);
#58324=ORIENTED_EDGE('',*,*,#43683,.T.);
#58325=ORIENTED_EDGE('',*,*,#43679,.F.);
#58326=ORIENTED_EDGE('',*,*,#43684,.T.);
#58327=ORIENTED_EDGE('',*,*,#43685,.T.);
#58328=ORIENTED_EDGE('',*,*,#43686,.T.);
#58329=ORIENTED_EDGE('',*,*,#43682,.F.);
#58330=ORIENTED_EDGE('',*,*,#43687,.T.);
#58331=ORIENTED_EDGE('',*,*,#43688,.T.);
#58332=ORIENTED_EDGE('',*,*,#43634,.T.);
#58333=ORIENTED_EDGE('',*,*,#43685,.F.);
#58334=ORIENTED_EDGE('',*,*,#43689,.T.);
#58335=ORIENTED_EDGE('',*,*,#43690,.T.);
#58336=ORIENTED_EDGE('',*,*,#43691,.T.);
#58337=ORIENTED_EDGE('',*,*,#43688,.F.);
#58338=ORIENTED_EDGE('',*,*,#43692,.T.);
#58339=ORIENTED_EDGE('',*,*,#43690,.F.);
#58340=ORIENTED_EDGE('',*,*,#43693,.T.);
#58341=ORIENTED_EDGE('',*,*,#43694,.T.);
#58342=ORIENTED_EDGE('',*,*,#43695,.T.);
#58343=ORIENTED_EDGE('',*,*,#43696,.T.);
#58344=ORIENTED_EDGE('',*,*,#43697,.T.);
#58345=ORIENTED_EDGE('',*,*,#43694,.F.);
#58346=ORIENTED_EDGE('',*,*,#43698,.T.);
#58347=ORIENTED_EDGE('',*,*,#43696,.F.);
#58348=ORIENTED_EDGE('',*,*,#43699,.T.);
#58349=ORIENTED_EDGE('',*,*,#43700,.T.);
#58350=ORIENTED_EDGE('',*,*,#43701,.T.);
#58351=ORIENTED_EDGE('',*,*,#43702,.T.);
#58352=ORIENTED_EDGE('',*,*,#43703,.T.);
#58353=ORIENTED_EDGE('',*,*,#43700,.F.);
#58354=ORIENTED_EDGE('',*,*,#43704,.T.);
#58355=ORIENTED_EDGE('',*,*,#43705,.T.);
#58356=ORIENTED_EDGE('',*,*,#43639,.T.);
#58357=ORIENTED_EDGE('',*,*,#43702,.F.);
#58358=ORIENTED_EDGE('',*,*,#43706,.T.);
#58359=ORIENTED_EDGE('',*,*,#43677,.F.);
#58360=ORIENTED_EDGE('',*,*,#43707,.T.);
#58361=ORIENTED_EDGE('',*,*,#43705,.F.);
#58362=ORIENTED_EDGE('',*,*,#43708,.T.);
#58363=ORIENTED_EDGE('',*,*,#43662,.F.);
#58364=ORIENTED_EDGE('',*,*,#43709,.F.);
#58365=ORIENTED_EDGE('',*,*,#43697,.F.);
#58366=ORIENTED_EDGE('',*,*,#43710,.T.);
#58367=ORIENTED_EDGE('',*,*,#43660,.F.);
#58368=ORIENTED_EDGE('',*,*,#43710,.F.);
#58369=ORIENTED_EDGE('',*,*,#43701,.F.);
#58370=ORIENTED_EDGE('',*,*,#43711,.F.);
#58371=ORIENTED_EDGE('',*,*,#43658,.F.);
#58372=ORIENTED_EDGE('',*,*,#43711,.T.);
#58373=ORIENTED_EDGE('',*,*,#43703,.F.);
#58374=ORIENTED_EDGE('',*,*,#43638,.T.);
#58375=ORIENTED_EDGE('',*,*,#43674,.F.);
#58376=ORIENTED_EDGE('',*,*,#43640,.T.);
#58377=ORIENTED_EDGE('',*,*,#43707,.F.);
#58378=ORIENTED_EDGE('',*,*,#43712,.T.);
#58379=ORIENTED_EDGE('',*,*,#43673,.F.);
#58380=ORIENTED_EDGE('',*,*,#43712,.F.);
#58381=ORIENTED_EDGE('',*,*,#43676,.F.);
#58382=ORIENTED_EDGE('',*,*,#43713,.T.);
#58383=ORIENTED_EDGE('',*,*,#43678,.F.);
#58384=ORIENTED_EDGE('',*,*,#43708,.F.);
#58385=ORIENTED_EDGE('',*,*,#43706,.F.);
#58386=ORIENTED_EDGE('',*,*,#43704,.F.);
#58387=ORIENTED_EDGE('',*,*,#43699,.F.);
#58388=ORIENTED_EDGE('',*,*,#43698,.F.);
#58389=ORIENTED_EDGE('',*,*,#43693,.F.);
#58390=ORIENTED_EDGE('',*,*,#43692,.F.);
#58391=ORIENTED_EDGE('',*,*,#43689,.F.);
#58392=ORIENTED_EDGE('',*,*,#43687,.F.);
#58393=ORIENTED_EDGE('',*,*,#43684,.F.);
#58394=ORIENTED_EDGE('',*,*,#43681,.F.);
#58395=ORIENTED_EDGE('',*,*,#43602,.T.);
#58396=ORIENTED_EDGE('',*,*,#43601,.F.);
#58397=ORIENTED_EDGE('',*,*,#43531,.F.);
#58398=ORIENTED_EDGE('',*,*,#43599,.T.);
#58399=ORIENTED_EDGE('',*,*,#43586,.T.);
#58400=ORIENTED_EDGE('',*,*,#43613,.T.);
#58401=ORIENTED_EDGE('',*,*,#43612,.F.);
#58402=ORIENTED_EDGE('',*,*,#43548,.F.);
#58403=ORIENTED_EDGE('',*,*,#43610,.T.);
#58404=ORIENTED_EDGE('',*,*,#43567,.T.);
#58405=ORIENTED_EDGE('',*,*,#43625,.T.);
#58406=ORIENTED_EDGE('',*,*,#43665,.F.);
#58407=ORIENTED_EDGE('',*,*,#43635,.T.);
#58408=ORIENTED_EDGE('',*,*,#43691,.F.);
#58409=ORIENTED_EDGE('',*,*,#43714,.T.);
#58410=ORIENTED_EDGE('',*,*,#43667,.F.);
#58411=ORIENTED_EDGE('',*,*,#43715,.T.);
#58412=ORIENTED_EDGE('',*,*,#43686,.F.);
#58413=ORIENTED_EDGE('',*,*,#43633,.T.);
#58414=ORIENTED_EDGE('',*,*,#43669,.F.);
#58415=ORIENTED_EDGE('',*,*,#43716,.F.);
#58416=ORIENTED_EDGE('',*,*,#43683,.F.);
#58417=ORIENTED_EDGE('',*,*,#43715,.F.);
#58418=ORIENTED_EDGE('',*,*,#43717,.T.);
#58419=ORIENTED_EDGE('',*,*,#43718,.T.);
#58420=ORIENTED_EDGE('',*,*,#43719,.T.);
#58421=ORIENTED_EDGE('',*,*,#43718,.F.);
#58422=ORIENTED_EDGE('',*,*,#43717,.F.);
#58423=ORIENTED_EDGE('',*,*,#43720,.T.);
#58424=ORIENTED_EDGE('',*,*,#43721,.T.);
#58425=ORIENTED_EDGE('',*,*,#43720,.F.);
#58426=ORIENTED_EDGE('',*,*,#43722,.T.);
#58427=ORIENTED_EDGE('',*,*,#43723,.T.);
#58428=ORIENTED_EDGE('',*,*,#43724,.T.);
#58429=ORIENTED_EDGE('',*,*,#43725,.F.);
#58430=ORIENTED_EDGE('',*,*,#43726,.T.);
#58431=ORIENTED_EDGE('',*,*,#43727,.T.);
#58432=ORIENTED_EDGE('',*,*,#43728,.T.);
#58433=ORIENTED_EDGE('',*,*,#43729,.T.);
#58434=ORIENTED_EDGE('',*,*,#43730,.T.);
#58435=ORIENTED_EDGE('',*,*,#43731,.F.);
#58436=ORIENTED_EDGE('',*,*,#43732,.T.);
#58437=ORIENTED_EDGE('',*,*,#43733,.T.);
#58438=ORIENTED_EDGE('',*,*,#43734,.T.);
#58439=ORIENTED_EDGE('',*,*,#43735,.T.);
#58440=ORIENTED_EDGE('',*,*,#43736,.T.);
#58441=ORIENTED_EDGE('',*,*,#43737,.F.);
#58442=ORIENTED_EDGE('',*,*,#43738,.T.);
#58443=ORIENTED_EDGE('',*,*,#43739,.T.);
#58444=ORIENTED_EDGE('',*,*,#43740,.T.);
#58445=ORIENTED_EDGE('',*,*,#43741,.T.);
#58446=ORIENTED_EDGE('',*,*,#43742,.T.);
#58447=ORIENTED_EDGE('',*,*,#43743,.F.);
#58448=ORIENTED_EDGE('',*,*,#43744,.T.);
#58449=ORIENTED_EDGE('',*,*,#43745,.T.);
#58450=ORIENTED_EDGE('',*,*,#43746,.T.);
#58451=ORIENTED_EDGE('',*,*,#43747,.T.);
#58452=ORIENTED_EDGE('',*,*,#43748,.T.);
#58453=ORIENTED_EDGE('',*,*,#43749,.F.);
#58454=ORIENTED_EDGE('',*,*,#43750,.T.);
#58455=ORIENTED_EDGE('',*,*,#43751,.T.);
#58456=ORIENTED_EDGE('',*,*,#43752,.T.);
#58457=ORIENTED_EDGE('',*,*,#43753,.T.);
#58458=ORIENTED_EDGE('',*,*,#43754,.T.);
#58459=ORIENTED_EDGE('',*,*,#43755,.F.);
#58460=ORIENTED_EDGE('',*,*,#43756,.T.);
#58461=ORIENTED_EDGE('',*,*,#43757,.T.);
#58462=ORIENTED_EDGE('',*,*,#43758,.T.);
#58463=ORIENTED_EDGE('',*,*,#43759,.T.);
#58464=ORIENTED_EDGE('',*,*,#43760,.T.);
#58465=ORIENTED_EDGE('',*,*,#43761,.F.);
#58466=ORIENTED_EDGE('',*,*,#43762,.T.);
#58467=ORIENTED_EDGE('',*,*,#43763,.T.);
#58468=ORIENTED_EDGE('',*,*,#43764,.T.);
#58469=ORIENTED_EDGE('',*,*,#43765,.T.);
#58470=ORIENTED_EDGE('',*,*,#43766,.T.);
#58471=ORIENTED_EDGE('',*,*,#43767,.F.);
#58472=ORIENTED_EDGE('',*,*,#43768,.T.);
#58473=ORIENTED_EDGE('',*,*,#43769,.T.);
#58474=ORIENTED_EDGE('',*,*,#43770,.T.);
#58475=ORIENTED_EDGE('',*,*,#43771,.T.);
#58476=ORIENTED_EDGE('',*,*,#43772,.T.);
#58477=ORIENTED_EDGE('',*,*,#43773,.F.);
#58478=ORIENTED_EDGE('',*,*,#43774,.T.);
#58479=ORIENTED_EDGE('',*,*,#43775,.T.);
#58480=ORIENTED_EDGE('',*,*,#43776,.T.);
#58481=ORIENTED_EDGE('',*,*,#43777,.T.);
#58482=ORIENTED_EDGE('',*,*,#43778,.T.);
#58483=ORIENTED_EDGE('',*,*,#43779,.F.);
#58484=ORIENTED_EDGE('',*,*,#43780,.T.);
#58485=ORIENTED_EDGE('',*,*,#43781,.T.);
#58486=ORIENTED_EDGE('',*,*,#43719,.F.);
#58487=ORIENTED_EDGE('',*,*,#43721,.F.);
#58488=ORIENTED_EDGE('',*,*,#43782,.F.);
#58489=ORIENTED_EDGE('',*,*,#43783,.F.);
#58490=ORIENTED_EDGE('',*,*,#43784,.F.);
#58491=ORIENTED_EDGE('',*,*,#43785,.F.);
#58492=ORIENTED_EDGE('',*,*,#43786,.F.);
#58493=ORIENTED_EDGE('',*,*,#43787,.F.);
#58494=ORIENTED_EDGE('',*,*,#43788,.F.);
#58495=ORIENTED_EDGE('',*,*,#43789,.F.);
#58496=ORIENTED_EDGE('',*,*,#43790,.F.);
#58497=ORIENTED_EDGE('',*,*,#43791,.F.);
#58498=ORIENTED_EDGE('',*,*,#43792,.F.);
#58499=ORIENTED_EDGE('',*,*,#43793,.F.);
#58500=ORIENTED_EDGE('',*,*,#43794,.F.);
#58501=ORIENTED_EDGE('',*,*,#43795,.F.);
#58502=ORIENTED_EDGE('',*,*,#43796,.F.);
#58503=ORIENTED_EDGE('',*,*,#43797,.F.);
#58504=ORIENTED_EDGE('',*,*,#43798,.F.);
#58505=ORIENTED_EDGE('',*,*,#43799,.F.);
#58506=ORIENTED_EDGE('',*,*,#43800,.F.);
#58507=ORIENTED_EDGE('',*,*,#43801,.F.);
#58508=ORIENTED_EDGE('',*,*,#43802,.F.);
#58509=ORIENTED_EDGE('',*,*,#43803,.F.);
#58510=ORIENTED_EDGE('',*,*,#43804,.F.);
#58511=ORIENTED_EDGE('',*,*,#43805,.F.);
#58512=ORIENTED_EDGE('',*,*,#43806,.F.);
#58513=ORIENTED_EDGE('',*,*,#43807,.F.);
#58514=ORIENTED_EDGE('',*,*,#43808,.F.);
#58515=ORIENTED_EDGE('',*,*,#43809,.F.);
#58516=ORIENTED_EDGE('',*,*,#43810,.F.);
#58517=ORIENTED_EDGE('',*,*,#43811,.F.);
#58518=ORIENTED_EDGE('',*,*,#43812,.F.);
#58519=ORIENTED_EDGE('',*,*,#43813,.F.);
#58520=ORIENTED_EDGE('',*,*,#43814,.F.);
#58521=ORIENTED_EDGE('',*,*,#43815,.F.);
#58522=ORIENTED_EDGE('',*,*,#43816,.F.);
#58523=ORIENTED_EDGE('',*,*,#43817,.F.);
#58524=ORIENTED_EDGE('',*,*,#43818,.F.);
#58525=ORIENTED_EDGE('',*,*,#43819,.F.);
#58526=ORIENTED_EDGE('',*,*,#43820,.F.);
#58527=ORIENTED_EDGE('',*,*,#43821,.F.);
#58528=ORIENTED_EDGE('',*,*,#43822,.F.);
#58529=ORIENTED_EDGE('',*,*,#43823,.F.);
#58530=ORIENTED_EDGE('',*,*,#43824,.F.);
#58531=ORIENTED_EDGE('',*,*,#43825,.F.);
#58532=ORIENTED_EDGE('',*,*,#43826,.F.);
#58533=ORIENTED_EDGE('',*,*,#43827,.F.);
#58534=ORIENTED_EDGE('',*,*,#43828,.F.);
#58535=ORIENTED_EDGE('',*,*,#43829,.F.);
#58536=ORIENTED_EDGE('',*,*,#43830,.F.);
#58537=ORIENTED_EDGE('',*,*,#43831,.F.);
#58538=ORIENTED_EDGE('',*,*,#43832,.F.);
#58539=ORIENTED_EDGE('',*,*,#43833,.F.);
#58540=ORIENTED_EDGE('',*,*,#43834,.F.);
#58541=ORIENTED_EDGE('',*,*,#43835,.F.);
#58542=ORIENTED_EDGE('',*,*,#43836,.F.);
#58543=ORIENTED_EDGE('',*,*,#43837,.F.);
#58544=ORIENTED_EDGE('',*,*,#43838,.F.);
#58545=ORIENTED_EDGE('',*,*,#43839,.F.);
#58546=ORIENTED_EDGE('',*,*,#43840,.F.);
#58547=ORIENTED_EDGE('',*,*,#43841,.F.);
#58548=ORIENTED_EDGE('',*,*,#43842,.F.);
#58549=ORIENTED_EDGE('',*,*,#43843,.F.);
#58550=ORIENTED_EDGE('',*,*,#43841,.T.);
#58551=ORIENTED_EDGE('',*,*,#43844,.T.);
#58552=ORIENTED_EDGE('',*,*,#43777,.F.);
#58553=ORIENTED_EDGE('',*,*,#43840,.T.);
#58554=ORIENTED_EDGE('',*,*,#43845,.F.);
#58555=ORIENTED_EDGE('',*,*,#43778,.F.);
#58556=ORIENTED_EDGE('',*,*,#43844,.F.);
#58557=ORIENTED_EDGE('',*,*,#43839,.T.);
#58558=ORIENTED_EDGE('',*,*,#43846,.T.);
#58559=ORIENTED_EDGE('',*,*,#43779,.T.);
#58560=ORIENTED_EDGE('',*,*,#43845,.T.);
#58561=ORIENTED_EDGE('',*,*,#43838,.T.);
#58562=ORIENTED_EDGE('',*,*,#43847,.T.);
#58563=ORIENTED_EDGE('',*,*,#43780,.F.);
#58564=ORIENTED_EDGE('',*,*,#43846,.F.);
#58565=ORIENTED_EDGE('',*,*,#43848,.F.);
#58566=ORIENTED_EDGE('',*,*,#43781,.F.);
#58567=ORIENTED_EDGE('',*,*,#43847,.F.);
#58568=ORIENTED_EDGE('',*,*,#43837,.T.);
#58569=ORIENTED_EDGE('',*,*,#43843,.T.);
#58570=ORIENTED_EDGE('',*,*,#43776,.F.);
#58571=ORIENTED_EDGE('',*,*,#43849,.T.);
#58572=ORIENTED_EDGE('',*,*,#43782,.T.);
#58573=ORIENTED_EDGE('',*,*,#43848,.T.);
#58574=ORIENTED_EDGE('',*,*,#43836,.T.);
#58575=ORIENTED_EDGE('',*,*,#43850,.T.);
#58576=ORIENTED_EDGE('',*,*,#43722,.F.);
#58577=ORIENTED_EDGE('',*,*,#43851,.F.);
#58578=ORIENTED_EDGE('',*,*,#43787,.T.);
#58579=ORIENTED_EDGE('',*,*,#43852,.T.);
#58580=ORIENTED_EDGE('',*,*,#43771,.F.);
#58581=ORIENTED_EDGE('',*,*,#43786,.T.);
#58582=ORIENTED_EDGE('',*,*,#43853,.F.);
#58583=ORIENTED_EDGE('',*,*,#43772,.F.);
#58584=ORIENTED_EDGE('',*,*,#43852,.F.);
#58585=ORIENTED_EDGE('',*,*,#43785,.T.);
#58586=ORIENTED_EDGE('',*,*,#43854,.T.);
#58587=ORIENTED_EDGE('',*,*,#43773,.T.);
#58588=ORIENTED_EDGE('',*,*,#43853,.T.);
#58589=ORIENTED_EDGE('',*,*,#43784,.T.);
#58590=ORIENTED_EDGE('',*,*,#43855,.T.);
#58591=ORIENTED_EDGE('',*,*,#43774,.F.);
#58592=ORIENTED_EDGE('',*,*,#43854,.F.);
#58593=ORIENTED_EDGE('',*,*,#43849,.F.);
#58594=ORIENTED_EDGE('',*,*,#43775,.F.);
#58595=ORIENTED_EDGE('',*,*,#43855,.F.);
#58596=ORIENTED_EDGE('',*,*,#43783,.T.);
#58597=ORIENTED_EDGE('',*,*,#43851,.T.);
#58598=ORIENTED_EDGE('',*,*,#43770,.F.);
#58599=ORIENTED_EDGE('',*,*,#43856,.T.);
#58600=ORIENTED_EDGE('',*,*,#43788,.T.);
#58601=ORIENTED_EDGE('',*,*,#43857,.F.);
#58602=ORIENTED_EDGE('',*,*,#43793,.T.);
#58603=ORIENTED_EDGE('',*,*,#43858,.T.);
#58604=ORIENTED_EDGE('',*,*,#43765,.F.);
#58605=ORIENTED_EDGE('',*,*,#43792,.T.);
#58606=ORIENTED_EDGE('',*,*,#43859,.F.);
#58607=ORIENTED_EDGE('',*,*,#43766,.F.);
#58608=ORIENTED_EDGE('',*,*,#43858,.F.);
#58609=ORIENTED_EDGE('',*,*,#43791,.T.);
#58610=ORIENTED_EDGE('',*,*,#43860,.T.);
#58611=ORIENTED_EDGE('',*,*,#43767,.T.);
#58612=ORIENTED_EDGE('',*,*,#43859,.T.);
#58613=ORIENTED_EDGE('',*,*,#43790,.T.);
#58614=ORIENTED_EDGE('',*,*,#43861,.T.);
#58615=ORIENTED_EDGE('',*,*,#43768,.F.);
#58616=ORIENTED_EDGE('',*,*,#43860,.F.);
#58617=ORIENTED_EDGE('',*,*,#43856,.F.);
#58618=ORIENTED_EDGE('',*,*,#43769,.F.);
#58619=ORIENTED_EDGE('',*,*,#43861,.F.);
#58620=ORIENTED_EDGE('',*,*,#43789,.T.);
#58621=ORIENTED_EDGE('',*,*,#43857,.T.);
#58622=ORIENTED_EDGE('',*,*,#43764,.F.);
#58623=ORIENTED_EDGE('',*,*,#43862,.T.);
#58624=ORIENTED_EDGE('',*,*,#43794,.T.);
#58625=ORIENTED_EDGE('',*,*,#43863,.F.);
#58626=ORIENTED_EDGE('',*,*,#43799,.T.);
#58627=ORIENTED_EDGE('',*,*,#43864,.T.);
#58628=ORIENTED_EDGE('',*,*,#43759,.F.);
#58629=ORIENTED_EDGE('',*,*,#43798,.T.);
#58630=ORIENTED_EDGE('',*,*,#43865,.F.);
#58631=ORIENTED_EDGE('',*,*,#43760,.F.);
#58632=ORIENTED_EDGE('',*,*,#43864,.F.);
#58633=ORIENTED_EDGE('',*,*,#43797,.T.);
#58634=ORIENTED_EDGE('',*,*,#43866,.T.);
#58635=ORIENTED_EDGE('',*,*,#43761,.T.);
#58636=ORIENTED_EDGE('',*,*,#43865,.T.);
#58637=ORIENTED_EDGE('',*,*,#43796,.T.);
#58638=ORIENTED_EDGE('',*,*,#43867,.T.);
#58639=ORIENTED_EDGE('',*,*,#43762,.F.);
#58640=ORIENTED_EDGE('',*,*,#43866,.F.);
#58641=ORIENTED_EDGE('',*,*,#43862,.F.);
#58642=ORIENTED_EDGE('',*,*,#43763,.F.);
#58643=ORIENTED_EDGE('',*,*,#43867,.F.);
#58644=ORIENTED_EDGE('',*,*,#43795,.T.);
#58645=ORIENTED_EDGE('',*,*,#43863,.T.);
#58646=ORIENTED_EDGE('',*,*,#43758,.F.);
#58647=ORIENTED_EDGE('',*,*,#43868,.T.);
#58648=ORIENTED_EDGE('',*,*,#43800,.T.);
#58649=ORIENTED_EDGE('',*,*,#43869,.F.);
#58650=ORIENTED_EDGE('',*,*,#43805,.T.);
#58651=ORIENTED_EDGE('',*,*,#43870,.T.);
#58652=ORIENTED_EDGE('',*,*,#43753,.F.);
#58653=ORIENTED_EDGE('',*,*,#43804,.T.);
#58654=ORIENTED_EDGE('',*,*,#43871,.F.);
#58655=ORIENTED_EDGE('',*,*,#43754,.F.);
#58656=ORIENTED_EDGE('',*,*,#43870,.F.);
#58657=ORIENTED_EDGE('',*,*,#43803,.T.);
#58658=ORIENTED_EDGE('',*,*,#43872,.T.);
#58659=ORIENTED_EDGE('',*,*,#43755,.T.);
#58660=ORIENTED_EDGE('',*,*,#43871,.T.);
#58661=ORIENTED_EDGE('',*,*,#43802,.T.);
#58662=ORIENTED_EDGE('',*,*,#43873,.T.);
#58663=ORIENTED_EDGE('',*,*,#43756,.F.);
#58664=ORIENTED_EDGE('',*,*,#43872,.F.);
#58665=ORIENTED_EDGE('',*,*,#43868,.F.);
#58666=ORIENTED_EDGE('',*,*,#43757,.F.);
#58667=ORIENTED_EDGE('',*,*,#43873,.F.);
#58668=ORIENTED_EDGE('',*,*,#43801,.T.);
#58669=ORIENTED_EDGE('',*,*,#43869,.T.);
#58670=ORIENTED_EDGE('',*,*,#43752,.F.);
#58671=ORIENTED_EDGE('',*,*,#43874,.T.);
#58672=ORIENTED_EDGE('',*,*,#43806,.T.);
#58673=ORIENTED_EDGE('',*,*,#43875,.F.);
#58674=ORIENTED_EDGE('',*,*,#43811,.T.);
#58675=ORIENTED_EDGE('',*,*,#43876,.T.);
#58676=ORIENTED_EDGE('',*,*,#43747,.F.);
#58677=ORIENTED_EDGE('',*,*,#43810,.T.);
#58678=ORIENTED_EDGE('',*,*,#43877,.F.);
#58679=ORIENTED_EDGE('',*,*,#43748,.F.);
#58680=ORIENTED_EDGE('',*,*,#43876,.F.);
#58681=ORIENTED_EDGE('',*,*,#43809,.T.);
#58682=ORIENTED_EDGE('',*,*,#43878,.T.);
#58683=ORIENTED_EDGE('',*,*,#43749,.T.);
#58684=ORIENTED_EDGE('',*,*,#43877,.T.);
#58685=ORIENTED_EDGE('',*,*,#43808,.T.);
#58686=ORIENTED_EDGE('',*,*,#43879,.T.);
#58687=ORIENTED_EDGE('',*,*,#43750,.F.);
#58688=ORIENTED_EDGE('',*,*,#43878,.F.);
#58689=ORIENTED_EDGE('',*,*,#43874,.F.);
#58690=ORIENTED_EDGE('',*,*,#43751,.F.);
#58691=ORIENTED_EDGE('',*,*,#43879,.F.);
#58692=ORIENTED_EDGE('',*,*,#43807,.T.);
#58693=ORIENTED_EDGE('',*,*,#43875,.T.);
#58694=ORIENTED_EDGE('',*,*,#43746,.F.);
#58695=ORIENTED_EDGE('',*,*,#43880,.T.);
#58696=ORIENTED_EDGE('',*,*,#43812,.T.);
#58697=ORIENTED_EDGE('',*,*,#43881,.F.);
#58698=ORIENTED_EDGE('',*,*,#43817,.T.);
#58699=ORIENTED_EDGE('',*,*,#43882,.T.);
#58700=ORIENTED_EDGE('',*,*,#43741,.F.);
#58701=ORIENTED_EDGE('',*,*,#43816,.T.);
#58702=ORIENTED_EDGE('',*,*,#43883,.F.);
#58703=ORIENTED_EDGE('',*,*,#43742,.F.);
#58704=ORIENTED_EDGE('',*,*,#43882,.F.);
#58705=ORIENTED_EDGE('',*,*,#43815,.T.);
#58706=ORIENTED_EDGE('',*,*,#43884,.T.);
#58707=ORIENTED_EDGE('',*,*,#43743,.T.);
#58708=ORIENTED_EDGE('',*,*,#43883,.T.);
#58709=ORIENTED_EDGE('',*,*,#43814,.T.);
#58710=ORIENTED_EDGE('',*,*,#43885,.T.);
#58711=ORIENTED_EDGE('',*,*,#43744,.F.);
#58712=ORIENTED_EDGE('',*,*,#43884,.F.);
#58713=ORIENTED_EDGE('',*,*,#43880,.F.);
#58714=ORIENTED_EDGE('',*,*,#43745,.F.);
#58715=ORIENTED_EDGE('',*,*,#43885,.F.);
#58716=ORIENTED_EDGE('',*,*,#43813,.T.);
#58717=ORIENTED_EDGE('',*,*,#43881,.T.);
#58718=ORIENTED_EDGE('',*,*,#43740,.F.);
#58719=ORIENTED_EDGE('',*,*,#43886,.T.);
#58720=ORIENTED_EDGE('',*,*,#43818,.T.);
#58721=ORIENTED_EDGE('',*,*,#43887,.F.);
#58722=ORIENTED_EDGE('',*,*,#43823,.T.);
#58723=ORIENTED_EDGE('',*,*,#43888,.T.);
#58724=ORIENTED_EDGE('',*,*,#43735,.F.);
#58725=ORIENTED_EDGE('',*,*,#43822,.T.);
#58726=ORIENTED_EDGE('',*,*,#43889,.F.);
#58727=ORIENTED_EDGE('',*,*,#43736,.F.);
#58728=ORIENTED_EDGE('',*,*,#43888,.F.);
#58729=ORIENTED_EDGE('',*,*,#43821,.T.);
#58730=ORIENTED_EDGE('',*,*,#43890,.T.);
#58731=ORIENTED_EDGE('',*,*,#43737,.T.);
#58732=ORIENTED_EDGE('',*,*,#43889,.T.);
#58733=ORIENTED_EDGE('',*,*,#43820,.T.);
#58734=ORIENTED_EDGE('',*,*,#43891,.T.);
#58735=ORIENTED_EDGE('',*,*,#43738,.F.);
#58736=ORIENTED_EDGE('',*,*,#43890,.F.);
#58737=ORIENTED_EDGE('',*,*,#43886,.F.);
#58738=ORIENTED_EDGE('',*,*,#43739,.F.);
#58739=ORIENTED_EDGE('',*,*,#43891,.F.);
#58740=ORIENTED_EDGE('',*,*,#43819,.T.);
#58741=ORIENTED_EDGE('',*,*,#43887,.T.);
#58742=ORIENTED_EDGE('',*,*,#43734,.F.);
#58743=ORIENTED_EDGE('',*,*,#43892,.T.);
#58744=ORIENTED_EDGE('',*,*,#43824,.T.);
#58745=ORIENTED_EDGE('',*,*,#43893,.F.);
#58746=ORIENTED_EDGE('',*,*,#43829,.T.);
#58747=ORIENTED_EDGE('',*,*,#43894,.T.);
#58748=ORIENTED_EDGE('',*,*,#43729,.F.);
#58749=ORIENTED_EDGE('',*,*,#43828,.T.);
#58750=ORIENTED_EDGE('',*,*,#43895,.F.);
#58751=ORIENTED_EDGE('',*,*,#43730,.F.);
#58752=ORIENTED_EDGE('',*,*,#43894,.F.);
#58753=ORIENTED_EDGE('',*,*,#43827,.T.);
#58754=ORIENTED_EDGE('',*,*,#43896,.T.);
#58755=ORIENTED_EDGE('',*,*,#43731,.T.);
#58756=ORIENTED_EDGE('',*,*,#43895,.T.);
#58757=ORIENTED_EDGE('',*,*,#43826,.T.);
#58758=ORIENTED_EDGE('',*,*,#43897,.T.);
#58759=ORIENTED_EDGE('',*,*,#43732,.F.);
#58760=ORIENTED_EDGE('',*,*,#43896,.F.);
#58761=ORIENTED_EDGE('',*,*,#43892,.F.);
#58762=ORIENTED_EDGE('',*,*,#43733,.F.);
#58763=ORIENTED_EDGE('',*,*,#43897,.F.);
#58764=ORIENTED_EDGE('',*,*,#43825,.T.);
#58765=ORIENTED_EDGE('',*,*,#43893,.T.);
#58766=ORIENTED_EDGE('',*,*,#43728,.F.);
#58767=ORIENTED_EDGE('',*,*,#43898,.T.);
#58768=ORIENTED_EDGE('',*,*,#43830,.T.);
#58769=ORIENTED_EDGE('',*,*,#43850,.F.);
#58770=ORIENTED_EDGE('',*,*,#43835,.T.);
#58771=ORIENTED_EDGE('',*,*,#43899,.T.);
#58772=ORIENTED_EDGE('',*,*,#43723,.F.);
#58773=ORIENTED_EDGE('',*,*,#43834,.T.);
#58774=ORIENTED_EDGE('',*,*,#43900,.F.);
#58775=ORIENTED_EDGE('',*,*,#43724,.F.);
#58776=ORIENTED_EDGE('',*,*,#43899,.F.);
#58777=ORIENTED_EDGE('',*,*,#43833,.T.);
#58778=ORIENTED_EDGE('',*,*,#43901,.T.);
#58779=ORIENTED_EDGE('',*,*,#43725,.T.);
#58780=ORIENTED_EDGE('',*,*,#43900,.T.);
#58781=ORIENTED_EDGE('',*,*,#43832,.T.);
#58782=ORIENTED_EDGE('',*,*,#43902,.T.);
#58783=ORIENTED_EDGE('',*,*,#43726,.F.);
#58784=ORIENTED_EDGE('',*,*,#43901,.F.);
#58785=ORIENTED_EDGE('',*,*,#43898,.F.);
#58786=ORIENTED_EDGE('',*,*,#43727,.F.);
#58787=ORIENTED_EDGE('',*,*,#43902,.F.);
#58788=ORIENTED_EDGE('',*,*,#43831,.T.);
#58789=ORIENTED_EDGE('',*,*,#43903,.T.);
#58790=ORIENTED_EDGE('',*,*,#43904,.T.);
#58791=ORIENTED_EDGE('',*,*,#43905,.F.);
#58792=ORIENTED_EDGE('',*,*,#43904,.F.);
#58793=ORIENTED_EDGE('',*,*,#43906,.T.);
#58794=ORIENTED_EDGE('',*,*,#43907,.T.);
#58795=ORIENTED_EDGE('',*,*,#43908,.T.);
#58796=ORIENTED_EDGE('',*,*,#43905,.T.);
#58797=ORIENTED_EDGE('',*,*,#43908,.F.);
#58798=ORIENTED_EDGE('',*,*,#43909,.T.);
#58799=ORIENTED_EDGE('',*,*,#43903,.F.);
#58800=ORIENTED_EDGE('',*,*,#43910,.T.);
#58801=ORIENTED_EDGE('',*,*,#43911,.F.);
#58802=ORIENTED_EDGE('',*,*,#43912,.F.);
#58803=ORIENTED_EDGE('',*,*,#43910,.F.);
#58804=ORIENTED_EDGE('',*,*,#43906,.F.);
#58805=ORIENTED_EDGE('',*,*,#43649,.T.);
#58806=ORIENTED_EDGE('',*,*,#43913,.T.);
#58807=ORIENTED_EDGE('',*,*,#43909,.F.);
#58808=ORIENTED_EDGE('',*,*,#43907,.F.);
#58809=ORIENTED_EDGE('',*,*,#43913,.F.);
#58810=ORIENTED_EDGE('',*,*,#43914,.T.);
#58811=ORIENTED_EDGE('',*,*,#43915,.T.);
#58812=ORIENTED_EDGE('',*,*,#43916,.F.);
#58813=ORIENTED_EDGE('',*,*,#43915,.F.);
#58814=ORIENTED_EDGE('',*,*,#43917,.T.);
#58815=ORIENTED_EDGE('',*,*,#43911,.T.);
#58816=ORIENTED_EDGE('',*,*,#43912,.T.);
#58817=ORIENTED_EDGE('',*,*,#43918,.T.);
#58818=ORIENTED_EDGE('',*,*,#43916,.T.);
#58819=ORIENTED_EDGE('',*,*,#43918,.F.);
#58820=ORIENTED_EDGE('',*,*,#43914,.F.);
#58821=ORIENTED_EDGE('',*,*,#43919,.T.);
#58822=ORIENTED_EDGE('',*,*,#43920,.F.);
#58823=ORIENTED_EDGE('',*,*,#43921,.F.);
#58824=ORIENTED_EDGE('',*,*,#43919,.F.);
#58825=ORIENTED_EDGE('',*,*,#43917,.F.);
#58826=ORIENTED_EDGE('',*,*,#43922,.T.);
#58827=ORIENTED_EDGE('',*,*,#43923,.T.);
#58828=ORIENTED_EDGE('',*,*,#43924,.F.);
#58829=ORIENTED_EDGE('',*,*,#43923,.F.);
#58830=ORIENTED_EDGE('',*,*,#43925,.T.);
#58831=ORIENTED_EDGE('',*,*,#43920,.T.);
#58832=ORIENTED_EDGE('',*,*,#43921,.T.);
#58833=ORIENTED_EDGE('',*,*,#43926,.T.);
#58834=ORIENTED_EDGE('',*,*,#43924,.T.);
#58835=ORIENTED_EDGE('',*,*,#43926,.F.);
#58836=ORIENTED_EDGE('',*,*,#43922,.F.);
#58837=ORIENTED_EDGE('',*,*,#43927,.T.);
#58838=ORIENTED_EDGE('',*,*,#43928,.F.);
#58839=ORIENTED_EDGE('',*,*,#43929,.F.);
#58840=ORIENTED_EDGE('',*,*,#43927,.F.);
#58841=ORIENTED_EDGE('',*,*,#43925,.F.);
#58842=ORIENTED_EDGE('',*,*,#43930,.T.);
#58843=ORIENTED_EDGE('',*,*,#43931,.T.);
#58844=ORIENTED_EDGE('',*,*,#43932,.F.);
#58845=ORIENTED_EDGE('',*,*,#43931,.F.);
#58846=ORIENTED_EDGE('',*,*,#43933,.T.);
#58847=ORIENTED_EDGE('',*,*,#43928,.T.);
#58848=ORIENTED_EDGE('',*,*,#43929,.T.);
#58849=ORIENTED_EDGE('',*,*,#43934,.T.);
#58850=ORIENTED_EDGE('',*,*,#43932,.T.);
#58851=ORIENTED_EDGE('',*,*,#43934,.F.);
#58852=ORIENTED_EDGE('',*,*,#43930,.F.);
#58853=ORIENTED_EDGE('',*,*,#43935,.T.);
#58854=ORIENTED_EDGE('',*,*,#43936,.F.);
#58855=ORIENTED_EDGE('',*,*,#43937,.F.);
#58856=ORIENTED_EDGE('',*,*,#43935,.F.);
#58857=ORIENTED_EDGE('',*,*,#43933,.F.);
#58858=ORIENTED_EDGE('',*,*,#43938,.T.);
#58859=ORIENTED_EDGE('',*,*,#43939,.T.);
#58860=ORIENTED_EDGE('',*,*,#43940,.F.);
#58861=ORIENTED_EDGE('',*,*,#43939,.F.);
#58862=ORIENTED_EDGE('',*,*,#43941,.T.);
#58863=ORIENTED_EDGE('',*,*,#43936,.T.);
#58864=ORIENTED_EDGE('',*,*,#43937,.T.);
#58865=ORIENTED_EDGE('',*,*,#43942,.T.);
#58866=ORIENTED_EDGE('',*,*,#43940,.T.);
#58867=ORIENTED_EDGE('',*,*,#43942,.F.);
#58868=ORIENTED_EDGE('',*,*,#43938,.F.);
#58869=ORIENTED_EDGE('',*,*,#43943,.T.);
#58870=ORIENTED_EDGE('',*,*,#43944,.F.);
#58871=ORIENTED_EDGE('',*,*,#43945,.F.);
#58872=ORIENTED_EDGE('',*,*,#43943,.F.);
#58873=ORIENTED_EDGE('',*,*,#43941,.F.);
#58874=ORIENTED_EDGE('',*,*,#43946,.T.);
#58875=ORIENTED_EDGE('',*,*,#43947,.T.);
#58876=ORIENTED_EDGE('',*,*,#43948,.F.);
#58877=ORIENTED_EDGE('',*,*,#43947,.F.);
#58878=ORIENTED_EDGE('',*,*,#43949,.T.);
#58879=ORIENTED_EDGE('',*,*,#43944,.T.);
#58880=ORIENTED_EDGE('',*,*,#43945,.T.);
#58881=ORIENTED_EDGE('',*,*,#43950,.T.);
#58882=ORIENTED_EDGE('',*,*,#43948,.T.);
#58883=ORIENTED_EDGE('',*,*,#43950,.F.);
#58884=ORIENTED_EDGE('',*,*,#43946,.F.);
#58885=ORIENTED_EDGE('',*,*,#43951,.T.);
#58886=ORIENTED_EDGE('',*,*,#43952,.F.);
#58887=ORIENTED_EDGE('',*,*,#43953,.F.);
#58888=ORIENTED_EDGE('',*,*,#43951,.F.);
#58889=ORIENTED_EDGE('',*,*,#43949,.F.);
#58890=ORIENTED_EDGE('',*,*,#43954,.T.);
#58891=ORIENTED_EDGE('',*,*,#43955,.T.);
#58892=ORIENTED_EDGE('',*,*,#43956,.F.);
#58893=ORIENTED_EDGE('',*,*,#43955,.F.);
#58894=ORIENTED_EDGE('',*,*,#43957,.T.);
#58895=ORIENTED_EDGE('',*,*,#43952,.T.);
#58896=ORIENTED_EDGE('',*,*,#43953,.T.);
#58897=ORIENTED_EDGE('',*,*,#43958,.T.);
#58898=ORIENTED_EDGE('',*,*,#43956,.T.);
#58899=ORIENTED_EDGE('',*,*,#43958,.F.);
#58900=ORIENTED_EDGE('',*,*,#43954,.F.);
#58901=ORIENTED_EDGE('',*,*,#43959,.T.);
#58902=ORIENTED_EDGE('',*,*,#43960,.F.);
#58903=ORIENTED_EDGE('',*,*,#43961,.F.);
#58904=ORIENTED_EDGE('',*,*,#43959,.F.);
#58905=ORIENTED_EDGE('',*,*,#43957,.F.);
#58906=ORIENTED_EDGE('',*,*,#43962,.T.);
#58907=ORIENTED_EDGE('',*,*,#43963,.T.);
#58908=ORIENTED_EDGE('',*,*,#43964,.F.);
#58909=ORIENTED_EDGE('',*,*,#43963,.F.);
#58910=ORIENTED_EDGE('',*,*,#43965,.T.);
#58911=ORIENTED_EDGE('',*,*,#43960,.T.);
#58912=ORIENTED_EDGE('',*,*,#43961,.T.);
#58913=ORIENTED_EDGE('',*,*,#43966,.T.);
#58914=ORIENTED_EDGE('',*,*,#43964,.T.);
#58915=ORIENTED_EDGE('',*,*,#43966,.F.);
#58916=ORIENTED_EDGE('',*,*,#43962,.F.);
#58917=ORIENTED_EDGE('',*,*,#43967,.T.);
#58918=ORIENTED_EDGE('',*,*,#43968,.F.);
#58919=ORIENTED_EDGE('',*,*,#43969,.F.);
#58920=ORIENTED_EDGE('',*,*,#43967,.F.);
#58921=ORIENTED_EDGE('',*,*,#43965,.F.);
#58922=ORIENTED_EDGE('',*,*,#43970,.T.);
#58923=ORIENTED_EDGE('',*,*,#43971,.T.);
#58924=ORIENTED_EDGE('',*,*,#43972,.F.);
#58925=ORIENTED_EDGE('',*,*,#43971,.F.);
#58926=ORIENTED_EDGE('',*,*,#43973,.T.);
#58927=ORIENTED_EDGE('',*,*,#43968,.T.);
#58928=ORIENTED_EDGE('',*,*,#43969,.T.);
#58929=ORIENTED_EDGE('',*,*,#43974,.T.);
#58930=ORIENTED_EDGE('',*,*,#43972,.T.);
#58931=ORIENTED_EDGE('',*,*,#43974,.F.);
#58932=ORIENTED_EDGE('',*,*,#43970,.F.);
#58933=ORIENTED_EDGE('',*,*,#43975,.T.);
#58934=ORIENTED_EDGE('',*,*,#43976,.F.);
#58935=ORIENTED_EDGE('',*,*,#43977,.F.);
#58936=ORIENTED_EDGE('',*,*,#43975,.F.);
#58937=ORIENTED_EDGE('',*,*,#43973,.F.);
#58938=ORIENTED_EDGE('',*,*,#43978,.T.);
#58939=ORIENTED_EDGE('',*,*,#43979,.T.);
#58940=ORIENTED_EDGE('',*,*,#43980,.F.);
#58941=ORIENTED_EDGE('',*,*,#43979,.F.);
#58942=ORIENTED_EDGE('',*,*,#43981,.T.);
#58943=ORIENTED_EDGE('',*,*,#43976,.T.);
#58944=ORIENTED_EDGE('',*,*,#43977,.T.);
#58945=ORIENTED_EDGE('',*,*,#43982,.T.);
#58946=ORIENTED_EDGE('',*,*,#43980,.T.);
#58947=ORIENTED_EDGE('',*,*,#43982,.F.);
#58948=ORIENTED_EDGE('',*,*,#43978,.F.);
#58949=ORIENTED_EDGE('',*,*,#43983,.T.);
#58950=ORIENTED_EDGE('',*,*,#43984,.F.);
#58951=ORIENTED_EDGE('',*,*,#43985,.F.);
#58952=ORIENTED_EDGE('',*,*,#43983,.F.);
#58953=ORIENTED_EDGE('',*,*,#43981,.F.);
#58954=ORIENTED_EDGE('',*,*,#43986,.T.);
#58955=ORIENTED_EDGE('',*,*,#43987,.T.);
#58956=ORIENTED_EDGE('',*,*,#43988,.F.);
#58957=ORIENTED_EDGE('',*,*,#43987,.F.);
#58958=ORIENTED_EDGE('',*,*,#43989,.T.);
#58959=ORIENTED_EDGE('',*,*,#43984,.T.);
#58960=ORIENTED_EDGE('',*,*,#43985,.T.);
#58961=ORIENTED_EDGE('',*,*,#43990,.T.);
#58962=ORIENTED_EDGE('',*,*,#43988,.T.);
#58963=ORIENTED_EDGE('',*,*,#43990,.F.);
#58964=ORIENTED_EDGE('',*,*,#43986,.F.);
#58965=ORIENTED_EDGE('',*,*,#43991,.T.);
#58966=ORIENTED_EDGE('',*,*,#43992,.F.);
#58967=ORIENTED_EDGE('',*,*,#43993,.F.);
#58968=ORIENTED_EDGE('',*,*,#43991,.F.);
#58969=ORIENTED_EDGE('',*,*,#43989,.F.);
#58970=ORIENTED_EDGE('',*,*,#43994,.T.);
#58971=ORIENTED_EDGE('',*,*,#43995,.T.);
#58972=ORIENTED_EDGE('',*,*,#43996,.F.);
#58973=ORIENTED_EDGE('',*,*,#43995,.F.);
#58974=ORIENTED_EDGE('',*,*,#43997,.T.);
#58975=ORIENTED_EDGE('',*,*,#43992,.T.);
#58976=ORIENTED_EDGE('',*,*,#43993,.T.);
#58977=ORIENTED_EDGE('',*,*,#43998,.T.);
#58978=ORIENTED_EDGE('',*,*,#43996,.T.);
#58979=ORIENTED_EDGE('',*,*,#43998,.F.);
#58980=ORIENTED_EDGE('',*,*,#43994,.F.);
#58981=ORIENTED_EDGE('',*,*,#43999,.T.);
#58982=ORIENTED_EDGE('',*,*,#44000,.F.);
#58983=ORIENTED_EDGE('',*,*,#44001,.F.);
#58984=ORIENTED_EDGE('',*,*,#43999,.F.);
#58985=ORIENTED_EDGE('',*,*,#43997,.F.);
#58986=ORIENTED_EDGE('',*,*,#44002,.T.);
#58987=ORIENTED_EDGE('',*,*,#44003,.T.);
#58988=ORIENTED_EDGE('',*,*,#44004,.F.);
#58989=ORIENTED_EDGE('',*,*,#44003,.F.);
#58990=ORIENTED_EDGE('',*,*,#44005,.T.);
#58991=ORIENTED_EDGE('',*,*,#44000,.T.);
#58992=ORIENTED_EDGE('',*,*,#44001,.T.);
#58993=ORIENTED_EDGE('',*,*,#44006,.T.);
#58994=ORIENTED_EDGE('',*,*,#44004,.T.);
#58995=ORIENTED_EDGE('',*,*,#44006,.F.);
#58996=ORIENTED_EDGE('',*,*,#44002,.F.);
#58997=ORIENTED_EDGE('',*,*,#44007,.T.);
#58998=ORIENTED_EDGE('',*,*,#44008,.F.);
#58999=ORIENTED_EDGE('',*,*,#44009,.F.);
#59000=ORIENTED_EDGE('',*,*,#44007,.F.);
#59001=ORIENTED_EDGE('',*,*,#44005,.F.);
#59002=ORIENTED_EDGE('',*,*,#44010,.T.);
#59003=ORIENTED_EDGE('',*,*,#44011,.T.);
#59004=ORIENTED_EDGE('',*,*,#44012,.F.);
#59005=ORIENTED_EDGE('',*,*,#44011,.F.);
#59006=ORIENTED_EDGE('',*,*,#44013,.T.);
#59007=ORIENTED_EDGE('',*,*,#44008,.T.);
#59008=ORIENTED_EDGE('',*,*,#44009,.T.);
#59009=ORIENTED_EDGE('',*,*,#44014,.T.);
#59010=ORIENTED_EDGE('',*,*,#44012,.T.);
#59011=ORIENTED_EDGE('',*,*,#44014,.F.);
#59012=ORIENTED_EDGE('',*,*,#43671,.F.);
#59013=ORIENTED_EDGE('',*,*,#43713,.F.);
#59014=ORIENTED_EDGE('',*,*,#43680,.F.);
#59015=ORIENTED_EDGE('',*,*,#43716,.T.);
#59016=ORIENTED_EDGE('',*,*,#44010,.F.);
#59017=ORIENTED_EDGE('',*,*,#44015,.T.);
#59018=ORIENTED_EDGE('',*,*,#44016,.T.);
#59019=ORIENTED_EDGE('',*,*,#44017,.T.);
#59020=ORIENTED_EDGE('',*,*,#44015,.F.);
#59021=ORIENTED_EDGE('',*,*,#44013,.F.);
#59022=ORIENTED_EDGE('',*,*,#44018,.F.);
#59023=ORIENTED_EDGE('',*,*,#44019,.F.);
#59024=ORIENTED_EDGE('',*,*,#44020,.T.);
#59025=ORIENTED_EDGE('',*,*,#44021,.F.);
#59026=ORIENTED_EDGE('',*,*,#44020,.F.);
#59027=ORIENTED_EDGE('',*,*,#44017,.F.);
#59028=ORIENTED_EDGE('',*,*,#44022,.T.);
#59029=ORIENTED_EDGE('',*,*,#44021,.T.);
#59030=ORIENTED_EDGE('',*,*,#44022,.F.);
#59031=ORIENTED_EDGE('',*,*,#44016,.F.);
#59032=ORIENTED_EDGE('',*,*,#44018,.T.);
#59033=ORIENTED_EDGE('',*,*,#44019,.T.);
#59034=ORIENTED_EDGE('',*,*,#44023,.T.);
#59035=ORIENTED_EDGE('',*,*,#43642,.T.);
#59036=ORIENTED_EDGE('',*,*,#44023,.F.);
#59037=ORIENTED_EDGE('',*,*,#43626,.F.);
#59038=ORIENTED_EDGE('',*,*,#44024,.T.);
#59039=ORIENTED_EDGE('',*,*,#43842,.T.);
#59040=ORIENTED_EDGE('',*,*,#44024,.F.);
#59041=ORIENTED_EDGE('',*,*,#43664,.F.);
#59042=ORIENTED_EDGE('',*,*,#43714,.F.);
#59043=ORIENTED_EDGE('',*,*,#43695,.F.);
#59044=ORIENTED_EDGE('',*,*,#43709,.T.);
#59045=ORIENTED_EDGE('',*,*,#43655,.F.);
#87052=CYLINDRICAL_SURFACE('',#94907,1.2645);
#87053=CYLINDRICAL_SURFACE('',#94909,1.2645);
#87054=CYLINDRICAL_SURFACE('',#94910,1.2645);
#87055=CYLINDRICAL_SURFACE('',#94911,1.2645);
#87056=CYLINDRICAL_SURFACE('',#94913,1.2645);
#87057=CYLINDRICAL_SURFACE('',#94915,1.2645);
#87058=CYLINDRICAL_SURFACE('',#94916,1.2645);
#87059=CYLINDRICAL_SURFACE('',#94917,1.2645);
#87060=CYLINDRICAL_SURFACE('',#94919,1.543);
#87061=CYLINDRICAL_SURFACE('',#94921,1.543);
#87062=CYLINDRICAL_SURFACE('',#94922,1.543);
#87063=CYLINDRICAL_SURFACE('',#94923,1.543);
#87064=CYLINDRICAL_SURFACE('',#94925,1.543);
#87065=CYLINDRICAL_SURFACE('',#94927,1.543);
#87066=CYLINDRICAL_SURFACE('',#94928,1.543);
#87067=CYLINDRICAL_SURFACE('',#94929,1.543);
#87068=CYLINDRICAL_SURFACE('',#94931,1.543);
#87069=CYLINDRICAL_SURFACE('',#94932,1.543);
#87070=CYLINDRICAL_SURFACE('',#94933,1.2645);
#87071=CYLINDRICAL_SURFACE('',#94934,1.2645);
#87072=CYLINDRICAL_SURFACE('',#94949,8.);
#87073=CYLINDRICAL_SURFACE('',#94957,18.25);
#87074=CYLINDRICAL_SURFACE('',#94966,18.25);
#87075=CYLINDRICAL_SURFACE('',#94975,2.5);
#87076=CYLINDRICAL_SURFACE('',#95020,3.50000000056584);
#87077=CYLINDRICAL_SURFACE('',#95022,1.);
#87078=CYLINDRICAL_SURFACE('',#95023,1.);
#87079=CYLINDRICAL_SURFACE('',#95026,1.);
#87080=CYLINDRICAL_SURFACE('',#95027,1.);
#87081=CYLINDRICAL_SURFACE('',#95032,1.);
#87082=CYLINDRICAL_SURFACE('',#95079,3.);
#87083=CYLINDRICAL_SURFACE('',#95081,1.875);
#87084=CYLINDRICAL_SURFACE('',#95082,1.875);
#87085=CYLINDRICAL_SURFACE('',#95084,3.);
#87086=CYLINDRICAL_SURFACE('',#95086,1.875);
#87087=CYLINDRICAL_SURFACE('',#95088,3.);
#87088=CYLINDRICAL_SURFACE('',#95090,1.875);
#87089=CYLINDRICAL_SURFACE('',#95092,3.);
#87090=CYLINDRICAL_SURFACE('',#95094,1.875);
#87091=CYLINDRICAL_SURFACE('',#95096,3.);
#87092=CYLINDRICAL_SURFACE('',#95098,1.875);
#87093=CYLINDRICAL_SURFACE('',#95100,3.);
#87094=CYLINDRICAL_SURFACE('',#95102,1.875);
#87095=CYLINDRICAL_SURFACE('',#95104,3.);
#87096=CYLINDRICAL_SURFACE('',#95106,1.875);
#87097=CYLINDRICAL_SURFACE('',#95108,3.);
#87098=CYLINDRICAL_SURFACE('',#95110,1.875);
#87099=CYLINDRICAL_SURFACE('',#95112,3.);
#87100=CYLINDRICAL_SURFACE('',#95114,1.875);
#87101=CYLINDRICAL_SURFACE('',#95116,3.);
#87102=CYLINDRICAL_SURFACE('',#95125,17.5);
#87103=CYLINDRICAL_SURFACE('',#95128,17.5);
#87104=CYLINDRICAL_SURFACE('',#95134,17.5);
#87105=CYLINDRICAL_SURFACE('',#95142,17.5);
#87106=CYLINDRICAL_SURFACE('',#95150,17.5);
#87107=CYLINDRICAL_SURFACE('',#95158,17.5);
#87108=CYLINDRICAL_SURFACE('',#95166,17.5);
#87109=CYLINDRICAL_SURFACE('',#95174,17.5);
#87110=CYLINDRICAL_SURFACE('',#95182,17.5);
#87111=CYLINDRICAL_SURFACE('',#95190,17.5);
#87112=CYLINDRICAL_SURFACE('',#95198,17.5);
#87113=CYLINDRICAL_SURFACE('',#95206,17.5);
#87114=CYLINDRICAL_SURFACE('',#95214,17.5);
#87115=CYLINDRICAL_SURFACE('',#95222,17.5);
#87116=CYLINDRICAL_SURFACE('',#95230,3.49999999943895);
#87117=CYLINDRICAL_SURFACE('',#95231,17.5);
#87118=CYLINDRICAL_SURFACE('',#95239,17.5);
#87119=CYLINDRICAL_SURFACE('',#95240,1.5);
#88815=ADVANCED_FACE('',(#6351),#87052,.F.);
#88816=ADVANCED_FACE('',(#6352),#87053,.F.);
#88817=ADVANCED_FACE('',(#6353),#87054,.F.);
#88818=ADVANCED_FACE('',(#6354),#87055,.F.);
#88819=ADVANCED_FACE('',(#6355),#87056,.F.);
#88820=ADVANCED_FACE('',(#6356),#87057,.F.);
#88821=ADVANCED_FACE('',(#6357),#87058,.F.);
#88822=ADVANCED_FACE('',(#6358),#87059,.F.);
#88823=ADVANCED_FACE('',(#6359),#87060,.F.);
#88824=ADVANCED_FACE('',(#6360),#87061,.F.);
#88825=ADVANCED_FACE('',(#6361),#87062,.F.);
#88826=ADVANCED_FACE('',(#6362),#87063,.F.);
#88827=ADVANCED_FACE('',(#6363),#87064,.F.);
#88828=ADVANCED_FACE('',(#6364),#87065,.F.);
#88829=ADVANCED_FACE('',(#6365),#87066,.F.);
#88830=ADVANCED_FACE('',(#6366),#87067,.F.);
#88831=ADVANCED_FACE('',(#6367),#87068,.F.);
#88832=ADVANCED_FACE('',(#6368),#87069,.F.);
#88833=ADVANCED_FACE('',(#6369),#87070,.F.);
#88834=ADVANCED_FACE('',(#6370),#87071,.F.);
#88835=ADVANCED_FACE('',(#6371),#6181,.F.);
#88836=ADVANCED_FACE('',(#6372),#6182,.F.);
#88837=ADVANCED_FACE('',(#6373,#5113),#5278,.T.);
#88838=ADVANCED_FACE('',(#6374),#6183,.F.);
#88839=ADVANCED_FACE('',(#6375),#6184,.F.);
#88840=ADVANCED_FACE('',(#6376,#5114),#5279,.T.);
#88841=ADVANCED_FACE('',(#6377),#4614,.T.);
#88842=ADVANCED_FACE('',(#6378),#87072,.T.);
#88843=ADVANCED_FACE('',(#6379,#5115),#5280,.F.);
#88844=ADVANCED_FACE('',(#6380),#4615,.T.);
#88845=ADVANCED_FACE('',(#6381),#87073,.T.);
#88846=ADVANCED_FACE('',(#6382,#5116),#5281,.F.);
#88847=ADVANCED_FACE('',(#6383),#4616,.T.);
#88848=ADVANCED_FACE('',(#6384),#87074,.T.);
#88849=ADVANCED_FACE('',(#6385,#5117),#5282,.T.);
#88850=ADVANCED_FACE('',(#6386),#4617,.F.);
#88851=ADVANCED_FACE('',(#6387,#5118),#5283,.T.);
#88852=ADVANCED_FACE('',(#6388),#87075,.F.);
#88853=ADVANCED_FACE('',(#6389),#4618,.T.);
#88854=ADVANCED_FACE('',(#6390),#4619,.F.);
#88855=ADVANCED_FACE('',(#6391),#5284,.T.);
#88856=ADVANCED_FACE('',(#6392),#4620,.T.);
#88857=ADVANCED_FACE('',(#6393),#5285,.T.);
#88858=ADVANCED_FACE('',(#6394),#4621,.F.);
#88859=ADVANCED_FACE('',(#6395),#4622,.F.);
#88860=ADVANCED_FACE('',(#6396),#5286,.T.);
#88861=ADVANCED_FACE('',(#6397),#4623,.T.);
#88862=ADVANCED_FACE('',(#6398),#5287,.T.);
#88863=ADVANCED_FACE('',(#6399),#4624,.F.);
#88864=ADVANCED_FACE('',(#6400),#5288,.T.);
#88865=ADVANCED_FACE('',(#6401),#4625,.T.);
#88866=ADVANCED_FACE('',(#6402),#5289,.T.);
#88867=ADVANCED_FACE('',(#6403),#4626,.F.);
#88868=ADVANCED_FACE('',(#6404),#4627,.T.);
#88869=ADVANCED_FACE('',(#6405),#4628,.F.);
#88870=ADVANCED_FACE('',(#6406),#5290,.T.);
#88871=ADVANCED_FACE('',(#6407),#4629,.T.);
#88872=ADVANCED_FACE('',(#6408),#5291,.T.);
#88873=ADVANCED_FACE('',(#6409),#4630,.F.);
#88874=ADVANCED_FACE('',(#6410),#4631,.T.);
#88875=ADVANCED_FACE('',(#6411),#4632,.F.);
#88876=ADVANCED_FACE('',(#6412),#87076,.T.);
#88877=ADVANCED_FACE('',(#6413),#5292,.T.);
#88878=ADVANCED_FACE('',(#6414),#87077,.F.);
#88879=ADVANCED_FACE('',(#6415),#87078,.F.);
#88880=ADVANCED_FACE('',(#6416),#5293,.T.);
#88881=ADVANCED_FACE('',(#6417,#5119,#5120,#5121),#5294,.F.);
#88882=ADVANCED_FACE('',(#6418),#87079,.F.);
#88883=ADVANCED_FACE('',(#6419),#87080,.F.);
#88884=ADVANCED_FACE('',(#6420),#5295,.T.);
#88885=ADVANCED_FACE('',(#6421),#4633,.F.);
#88886=ADVANCED_FACE('',(#6422),#87081,.F.);
#88887=ADVANCED_FACE('',(#6423,#5122),#5296,.T.);
#88888=ADVANCED_FACE('',(#6424),#5297,.T.);
#88889=ADVANCED_FACE('',(#6425,#5123),#5298,.F.);
#88890=ADVANCED_FACE('',(#6426),#5299,.T.);
#88891=ADVANCED_FACE('',(#6427),#6185,.T.);
#88892=ADVANCED_FACE('',(#6428),#87082,.T.);
#88893=ADVANCED_FACE('',(#6429),#6186,.T.);
#88894=ADVANCED_FACE('',(#6430),#5300,.T.);
#88895=ADVANCED_FACE('',(#6431),#87083,.T.);
#88896=ADVANCED_FACE('',(#6432),#87084,.T.);
#88897=ADVANCED_FACE('',(#6433),#5301,.T.);
#88898=ADVANCED_FACE('',(#6434),#6187,.T.);
#88899=ADVANCED_FACE('',(#6435),#87085,.T.);
#88900=ADVANCED_FACE('',(#6436),#6188,.T.);
#88901=ADVANCED_FACE('',(#6437),#5302,.T.);
#88902=ADVANCED_FACE('',(#6438),#87086,.T.);
#88903=ADVANCED_FACE('',(#6439),#5303,.T.);
#88904=ADVANCED_FACE('',(#6440),#6189,.T.);
#88905=ADVANCED_FACE('',(#6441),#87087,.T.);
#88906=ADVANCED_FACE('',(#6442),#6190,.T.);
#88907=ADVANCED_FACE('',(#6443),#5304,.T.);
#88908=ADVANCED_FACE('',(#6444),#87088,.T.);
#88909=ADVANCED_FACE('',(#6445),#5305,.T.);
#88910=ADVANCED_FACE('',(#6446),#6191,.T.);
#88911=ADVANCED_FACE('',(#6447),#87089,.T.);
#88912=ADVANCED_FACE('',(#6448),#6192,.T.);
#88913=ADVANCED_FACE('',(#6449),#5306,.T.);
#88914=ADVANCED_FACE('',(#6450),#87090,.T.);
#88915=ADVANCED_FACE('',(#6451),#5307,.T.);
#88916=ADVANCED_FACE('',(#6452),#6193,.T.);
#88917=ADVANCED_FACE('',(#6453),#87091,.T.);
#88918=ADVANCED_FACE('',(#6454),#6194,.T.);
#88919=ADVANCED_FACE('',(#6455),#5308,.T.);
#88920=ADVANCED_FACE('',(#6456),#87092,.T.);
#88921=ADVANCED_FACE('',(#6457),#5309,.T.);
#88922=ADVANCED_FACE('',(#6458),#6195,.T.);
#88923=ADVANCED_FACE('',(#6459),#87093,.T.);
#88924=ADVANCED_FACE('',(#6460),#6196,.T.);
#88925=ADVANCED_FACE('',(#6461),#5310,.T.);
#88926=ADVANCED_FACE('',(#6462),#87094,.T.);
#88927=ADVANCED_FACE('',(#6463),#5311,.T.);
#88928=ADVANCED_FACE('',(#6464),#6197,.T.);
#88929=ADVANCED_FACE('',(#6465),#87095,.T.);
#88930=ADVANCED_FACE('',(#6466),#6198,.T.);
#88931=ADVANCED_FACE('',(#6467),#5312,.T.);
#88932=ADVANCED_FACE('',(#6468),#87096,.T.);
#88933=ADVANCED_FACE('',(#6469),#5313,.T.);
#88934=ADVANCED_FACE('',(#6470),#6199,.T.);
#88935=ADVANCED_FACE('',(#6471),#87097,.T.);
#88936=ADVANCED_FACE('',(#6472),#6200,.T.);
#88937=ADVANCED_FACE('',(#6473),#5314,.T.);
#88938=ADVANCED_FACE('',(#6474),#87098,.T.);
#88939=ADVANCED_FACE('',(#6475),#5315,.T.);
#88940=ADVANCED_FACE('',(#6476),#6201,.T.);
#88941=ADVANCED_FACE('',(#6477),#87099,.T.);
#88942=ADVANCED_FACE('',(#6478),#6202,.T.);
#88943=ADVANCED_FACE('',(#6479),#5316,.T.);
#88944=ADVANCED_FACE('',(#6480),#87100,.T.);
#88945=ADVANCED_FACE('',(#6481),#5317,.T.);
#88946=ADVANCED_FACE('',(#6482),#6203,.T.);
#88947=ADVANCED_FACE('',(#6483),#87101,.T.);
#88948=ADVANCED_FACE('',(#6484),#6204,.T.);
#88949=ADVANCED_FACE('',(#6485),#5318,.T.);
#88950=ADVANCED_FACE('',(#6486),#4634,.T.);
#88951=ADVANCED_FACE('',(#6487),#4635,.T.);
#88952=ADVANCED_FACE('',(#6488),#87102,.T.);
#88953=ADVANCED_FACE('',(#6489),#87103,.T.);
#88954=ADVANCED_FACE('',(#6490),#4636,.T.);
#88955=ADVANCED_FACE('',(#6491),#4637,.T.);
#88956=ADVANCED_FACE('',(#6492),#87104,.T.);
#88957=ADVANCED_FACE('',(#6493),#4638,.T.);
#88958=ADVANCED_FACE('',(#6494),#4639,.T.);
#88959=ADVANCED_FACE('',(#6495),#87105,.T.);
#88960=ADVANCED_FACE('',(#6496),#4640,.T.);
#88961=ADVANCED_FACE('',(#6497),#4641,.T.);
#88962=ADVANCED_FACE('',(#6498),#87106,.T.);
#88963=ADVANCED_FACE('',(#6499),#4642,.T.);
#88964=ADVANCED_FACE('',(#6500),#4643,.T.);
#88965=ADVANCED_FACE('',(#6501),#87107,.T.);
#88966=ADVANCED_FACE('',(#6502),#4644,.T.);
#88967=ADVANCED_FACE('',(#6503),#4645,.T.);
#88968=ADVANCED_FACE('',(#6504),#87108,.T.);
#88969=ADVANCED_FACE('',(#6505),#4646,.T.);
#88970=ADVANCED_FACE('',(#6506),#4647,.T.);
#88971=ADVANCED_FACE('',(#6507),#87109,.T.);
#88972=ADVANCED_FACE('',(#6508),#4648,.T.);
#88973=ADVANCED_FACE('',(#6509),#4649,.T.);
#88974=ADVANCED_FACE('',(#6510),#87110,.T.);
#88975=ADVANCED_FACE('',(#6511),#4650,.T.);
#88976=ADVANCED_FACE('',(#6512),#4651,.T.);
#88977=ADVANCED_FACE('',(#6513),#87111,.T.);
#88978=ADVANCED_FACE('',(#6514),#4652,.T.);
#88979=ADVANCED_FACE('',(#6515),#4653,.T.);
#88980=ADVANCED_FACE('',(#6516),#87112,.T.);
#88981=ADVANCED_FACE('',(#6517),#4654,.T.);
#88982=ADVANCED_FACE('',(#6518),#4655,.T.);
#88983=ADVANCED_FACE('',(#6519),#87113,.T.);
#88984=ADVANCED_FACE('',(#6520),#4656,.T.);
#88985=ADVANCED_FACE('',(#6521),#4657,.T.);
#88986=ADVANCED_FACE('',(#6522),#87114,.T.);
#88987=ADVANCED_FACE('',(#6523),#4658,.T.);
#88988=ADVANCED_FACE('',(#6524),#4659,.T.);
#88989=ADVANCED_FACE('',(#6525),#87115,.T.);
#88990=ADVANCED_FACE('',(#6526),#4660,.T.);
#88991=ADVANCED_FACE('',(#6527),#4661,.T.);
#88992=ADVANCED_FACE('',(#6528),#87116,.T.);
#88993=ADVANCED_FACE('',(#6529),#87117,.T.);
#88994=ADVANCED_FACE('',(#6530),#4662,.T.);
#88995=ADVANCED_FACE('',(#6531),#4663,.T.);
#88996=ADVANCED_FACE('',(#6532),#87118,.T.);
#88997=ADVANCED_FACE('',(#6533),#87119,.T.);
#88998=ADVANCED_FACE('',(#6534),#5319,.T.);
#88999=ADVANCED_FACE('',(#6535),#5320,.T.);
#94623=CLOSED_SHELL('',(#88815,#88816,#88817,#88818,#88819,#88820,#88821,
#88822,#88823,#88824,#88825,#88826,#88827,#88828,#88829,#88830,#88831,#88832,
#88833,#88834,#88835,#88836,#88837,#88838,#88839,#88840,#88841,#88842,#88843,
#88844,#88845,#88846,#88847,#88848,#88849,#88850,#88851,#88852,#88853,#88854,
#88855,#88856,#88857,#88858,#88859,#88860,#88861,#88862,#88863,#88864,#88865,
#88866,#88867,#88868,#88869,#88870,#88871,#88872,#88873,#88874,#88875,#88876,
#88877,#88878,#88879,#88880,#88881,#88882,#88883,#88884,#88885,#88886,#88887,
#88888,#88889,#88890,#88891,#88892,#88893,#88894,#88895,#88896,#88897,#88898,
#88899,#88900,#88901,#88902,#88903,#88904,#88905,#88906,#88907,#88908,#88909,
#88910,#88911,#88912,#88913,#88914,#88915,#88916,#88917,#88918,#88919,#88920,
#88921,#88922,#88923,#88924,#88925,#88926,#88927,#88928,#88929,#88930,#88931,
#88932,#88933,#88934,#88935,#88936,#88937,#88938,#88939,#88940,#88941,#88942,
#88943,#88944,#88945,#88946,#88947,#88948,#88949,#88950,#88951,#88952,#88953,
#88954,#88955,#88956,#88957,#88958,#88959,#88960,#88961,#88962,#88963,#88964,
#88965,#88966,#88967,#88968,#88969,#88970,#88971,#88972,#88973,#88974,#88975,
#88976,#88977,#88978,#88979,#88980,#88981,#88982,#88983,#88984,#88985,#88986,
#88987,#88988,#88989,#88990,#88991,#88992,#88993,#88994,#88995,#88996,#88997,
#88998,#88999));
#94906=AXIS2_PLACEMENT_3D('',#130721,#105579,#105580);
#94907=AXIS2_PLACEMENT_3D('',#130722,#105581,#105582);
#94908=AXIS2_PLACEMENT_3D('',#130818,#105584,#105585);
#94909=AXIS2_PLACEMENT_3D('',#130903,#105586,#105587);
#94910=AXIS2_PLACEMENT_3D('',#131279,#105589,#105590);
#94911=AXIS2_PLACEMENT_3D('',#131637,#105592,#105593);
#94912=AXIS2_PLACEMENT_3D('',#131685,#105595,#105596);
#94913=AXIS2_PLACEMENT_3D('',#131810,#105597,#105598);
#94914=AXIS2_PLACEMENT_3D('',#131906,#105600,#105601);
#94915=AXIS2_PLACEMENT_3D('',#131993,#105602,#105603);
#94916=AXIS2_PLACEMENT_3D('',#132365,#105605,#105606);
#94917=AXIS2_PLACEMENT_3D('',#132723,#105608,#105609);
#94918=AXIS2_PLACEMENT_3D('',#132769,#105611,#105612);
#94919=AXIS2_PLACEMENT_3D('',#132894,#105613,#105614);
#94920=AXIS2_PLACEMENT_3D('',#132952,#105616,#105617);
#94921=AXIS2_PLACEMENT_3D('',#133011,#105618,#105619);
#94922=AXIS2_PLACEMENT_3D('',#133305,#105621,#105622);
#94923=AXIS2_PLACEMENT_3D('',#133658,#105624,#105625);
#94924=AXIS2_PLACEMENT_3D('',#133756,#105627,#105628);
#94925=AXIS2_PLACEMENT_3D('',#133849,#105629,#105630);
#94926=AXIS2_PLACEMENT_3D('',#133907,#105632,#105633);
#94927=AXIS2_PLACEMENT_3D('',#133968,#105634,#105635);
#94928=AXIS2_PLACEMENT_3D('',#134264,#105637,#105638);
#94929=AXIS2_PLACEMENT_3D('',#134617,#105640,#105641);
#94930=AXIS2_PLACEMENT_3D('',#134715,#105643,#105644);
#94931=AXIS2_PLACEMENT_3D('',#134808,#105645,#105646);
#94932=AXIS2_PLACEMENT_3D('',#135097,#105647,#105648);
#94933=AXIS2_PLACEMENT_3D('',#135386,#105649,#105650);
#94934=AXIS2_PLACEMENT_3D('',#135751,#105651,#105652);
#94935=AXIS2_PLACEMENT_3D('',#136626,#105653,#105654);
#94936=AXIS2_PLACEMENT_3D('',#136629,#105655,#105656);
#94937=AXIS2_PLACEMENT_3D('',#136633,#105658,#105659);
#94938=AXIS2_PLACEMENT_3D('',#136637,#105661,#105662);
#94939=AXIS2_PLACEMENT_3D('',#136638,#105663,#105664);
#94940=AXIS2_PLACEMENT_3D('',#137146,#105665,#105666);
#94941=AXIS2_PLACEMENT_3D('',#137149,#105667,#105668);
#94942=AXIS2_PLACEMENT_3D('',#137153,#105670,#105671);
#94943=AXIS2_PLACEMENT_3D('',#137157,#105673,#105674);
#94944=AXIS2_PLACEMENT_3D('',#137159,#105675,#105676);
#94945=AXIS2_PLACEMENT_3D('',#137160,#105677,#105678);
#94946=AXIS2_PLACEMENT_3D('',#137161,#105679,#105680);
#94947=AXIS2_PLACEMENT_3D('',#137163,#105681,#105682);
#94948=AXIS2_PLACEMENT_3D('',#137166,#105684,#105685);
#94949=AXIS2_PLACEMENT_3D('',#137167,#105686,#105687);
#94950=AXIS2_PLACEMENT_3D('',#137170,#105689,#105690);
#94951=AXIS2_PLACEMENT_3D('',#137171,#105691,#105692);
#94952=AXIS2_PLACEMENT_3D('',#137173,#105693,#105694);
#94953=AXIS2_PLACEMENT_3D('',#137174,#105695,#105696);
#94954=AXIS2_PLACEMENT_3D('',#137177,#105697,#105698);
#94955=AXIS2_PLACEMENT_3D('',#137180,#105700,#105701);
#94956=AXIS2_PLACEMENT_3D('',#137181,#105702,#105703);
#94957=AXIS2_PLACEMENT_3D('',#137182,#105704,#105705);
#94958=AXIS2_PLACEMENT_3D('',#137192,#105708,#105709);
#94959=AXIS2_PLACEMENT_3D('',#137207,#105712,#105713);
#94960=AXIS2_PLACEMENT_3D('',#137214,#105715,#105716);
#94961=AXIS2_PLACEMENT_3D('',#137216,#105717,#105718);
#94962=AXIS2_PLACEMENT_3D('',#137217,#105719,#105720);
#94963=AXIS2_PLACEMENT_3D('',#137220,#105721,#105722);
#94964=AXIS2_PLACEMENT_3D('',#137223,#105724,#105725);
#94965=AXIS2_PLACEMENT_3D('',#137224,#105726,#105727);
#94966=AXIS2_PLACEMENT_3D('',#137225,#105728,#105729);
#94967=AXIS2_PLACEMENT_3D('',#137227,#105730,#105731);
#94968=AXIS2_PLACEMENT_3D('',#137229,#105733,#105734);
#94969=AXIS2_PLACEMENT_3D('',#137231,#105735,#105736);
#94970=AXIS2_PLACEMENT_3D('',#137232,#105737,#105738);
#94971=AXIS2_PLACEMENT_3D('',#137234,#105739,#105740);
#94972=AXIS2_PLACEMENT_3D('',#137237,#105742,#105743);
#94973=AXIS2_PLACEMENT_3D('',#137238,#105744,#105745);
#94974=AXIS2_PLACEMENT_3D('',#137240,#105746,#105747);
#94975=AXIS2_PLACEMENT_3D('',#137241,#105748,#105749);
#94976=AXIS2_PLACEMENT_3D('',#137244,#105751,#105752);
#94977=AXIS2_PLACEMENT_3D('',#137245,#105753,#105754);
#94978=AXIS2_PLACEMENT_3D('',#137247,#105756,#105757);
#94979=AXIS2_PLACEMENT_3D('',#137250,#105759,#105760);
#94980=AXIS2_PLACEMENT_3D('',#137251,#105761,#105762);
#94981=AXIS2_PLACEMENT_3D('',#137255,#105765,#105766);
#94982=AXIS2_PLACEMENT_3D('',#137258,#105768,#105769);
#94983=AXIS2_PLACEMENT_3D('',#137259,#105770,#105771);
#94984=AXIS2_PLACEMENT_3D('',#137263,#105774,#105775);
#94985=AXIS2_PLACEMENT_3D('',#137264,#105776,#105777);
#94986=AXIS2_PLACEMENT_3D('',#137265,#105778,#105779);
#94987=AXIS2_PLACEMENT_3D('',#137268,#105781,#105782);
#94988=AXIS2_PLACEMENT_3D('',#137269,#105783,#105784);
#94989=AXIS2_PLACEMENT_3D('',#137273,#105787,#105788);
#94990=AXIS2_PLACEMENT_3D('',#137276,#105790,#105791);
#94991=AXIS2_PLACEMENT_3D('',#137277,#105792,#105793);
#94992=AXIS2_PLACEMENT_3D('',#137281,#105796,#105797);
#94993=AXIS2_PLACEMENT_3D('',#137282,#105798,#105799);
#94994=AXIS2_PLACEMENT_3D('',#137283,#105800,#105801);
#94995=AXIS2_PLACEMENT_3D('',#137292,#105806,#105807);
#94996=AXIS2_PLACEMENT_3D('',#137296,#105809,#105810);
#94997=AXIS2_PLACEMENT_3D('',#137297,#105811,#105812);
#94998=AXIS2_PLACEMENT_3D('',#137298,#105813,#105814);
#94999=AXIS2_PLACEMENT_3D('',#137304,#105818,#105819);
#95000=AXIS2_PLACEMENT_3D('',#137307,#105821,#105822);
#95001=AXIS2_PLACEMENT_3D('',#137308,#105823,#105824);
#95002=AXIS2_PLACEMENT_3D('',#137309,#105825,#105826);
#95003=AXIS2_PLACEMENT_3D('',#137312,#105828,#105829);
#95004=AXIS2_PLACEMENT_3D('',#137313,#105830,#105831);
#95005=AXIS2_PLACEMENT_3D('',#137317,#105833,#105834);
#95006=AXIS2_PLACEMENT_3D('',#137318,#105835,#105836);
#95007=AXIS2_PLACEMENT_3D('',#137319,#105837,#105838);
#95008=AXIS2_PLACEMENT_3D('',#137325,#105842,#105843);
#95009=AXIS2_PLACEMENT_3D('',#137329,#105845,#105846);
#95010=AXIS2_PLACEMENT_3D('',#137330,#105847,#105848);
#95011=AXIS2_PLACEMENT_3D('',#137331,#105849,#105850);
#95012=AXIS2_PLACEMENT_3D('',#137337,#105854,#105855);
#95013=AXIS2_PLACEMENT_3D('',#137340,#105857,#105858);
#95014=AXIS2_PLACEMENT_3D('',#137341,#105859,#105860);
#95015=AXIS2_PLACEMENT_3D('',#137342,#105861,#105862);
#95016=AXIS2_PLACEMENT_3D('',#137345,#105864,#105865);
#95017=AXIS2_PLACEMENT_3D('',#137346,#105866,#105867);
#95018=AXIS2_PLACEMENT_3D('',#137347,#105868,#105869);
#95019=AXIS2_PLACEMENT_3D('',#137348,#105870,#105871);
#95020=AXIS2_PLACEMENT_3D('',#137349,#105872,#105873);
#95021=AXIS2_PLACEMENT_3D('',#137352,#105876,#105877);
#95022=AXIS2_PLACEMENT_3D('',#137354,#105879,#105880);
#95023=AXIS2_PLACEMENT_3D('',#137355,#105881,#105882);
#95024=AXIS2_PLACEMENT_3D('',#137357,#105884,#105885);
#95025=AXIS2_PLACEMENT_3D('',#137359,#105887,#105888);
#95026=AXIS2_PLACEMENT_3D('',#137360,#105889,#105890);
#95027=AXIS2_PLACEMENT_3D('',#137362,#105892,#105893);
#95028=AXIS2_PLACEMENT_3D('',#137364,#105895,#105896);
#95029=AXIS2_PLACEMENT_3D('',#137366,#105898,#105899);
#95030=AXIS2_PLACEMENT_3D('',#137368,#105900,#105901);
#95031=AXIS2_PLACEMENT_3D('',#137371,#105903,#105904);
#95032=AXIS2_PLACEMENT_3D('',#137372,#105905,#105906);
#95033=AXIS2_PLACEMENT_3D('',#137375,#105908,#105909);
#95034=AXIS2_PLACEMENT_3D('',#137376,#105910,#105911);
#95035=AXIS2_PLACEMENT_3D('',#137379,#105912,#105913);
#95036=AXIS2_PLACEMENT_3D('',#137390,#105915,#105916);
#95037=AXIS2_PLACEMENT_3D('',#137401,#105918,#105919);
#95038=AXIS2_PLACEMENT_3D('',#137412,#105921,#105922);
#95039=AXIS2_PLACEMENT_3D('',#137423,#105924,#105925);
#95040=AXIS2_PLACEMENT_3D('',#137434,#105927,#105928);
#95041=AXIS2_PLACEMENT_3D('',#137445,#105930,#105931);
#95042=AXIS2_PLACEMENT_3D('',#137456,#105933,#105934);
#95043=AXIS2_PLACEMENT_3D('',#137467,#105936,#105937);
#95044=AXIS2_PLACEMENT_3D('',#137478,#105939,#105940);
#95045=AXIS2_PLACEMENT_3D('',#137489,#105942,#105943);
#95046=AXIS2_PLACEMENT_3D('',#137500,#105945,#105946);
#95047=AXIS2_PLACEMENT_3D('',#137511,#105948,#105949);
#95048=AXIS2_PLACEMENT_3D('',#137522,#105951,#105952);
#95049=AXIS2_PLACEMENT_3D('',#137533,#105954,#105955);
#95050=AXIS2_PLACEMENT_3D('',#137544,#105957,#105958);
#95051=AXIS2_PLACEMENT_3D('',#137555,#105960,#105961);
#95052=AXIS2_PLACEMENT_3D('',#137566,#105963,#105964);
#95053=AXIS2_PLACEMENT_3D('',#137577,#105966,#105967);
#95054=AXIS2_PLACEMENT_3D('',#137588,#105969,#105970);
#95055=AXIS2_PLACEMENT_3D('',#137597,#105972,#105973);
#95056=AXIS2_PLACEMENT_3D('',#137598,#105974,#105975);
#95057=AXIS2_PLACEMENT_3D('',#137601,#105976,#105977);
#95058=AXIS2_PLACEMENT_3D('',#137612,#105979,#105980);
#95059=AXIS2_PLACEMENT_3D('',#137623,#105982,#105983);
#95060=AXIS2_PLACEMENT_3D('',#137634,#105985,#105986);
#95061=AXIS2_PLACEMENT_3D('',#137645,#105988,#105989);
#95062=AXIS2_PLACEMENT_3D('',#137656,#105991,#105992);
#95063=AXIS2_PLACEMENT_3D('',#137667,#105994,#105995);
#95064=AXIS2_PLACEMENT_3D('',#137678,#105997,#105998);
#95065=AXIS2_PLACEMENT_3D('',#137689,#106000,#106001);
#95066=AXIS2_PLACEMENT_3D('',#137700,#106003,#106004);
#95067=AXIS2_PLACEMENT_3D('',#137711,#106006,#106007);
#95068=AXIS2_PLACEMENT_3D('',#137722,#106009,#106010);
#95069=AXIS2_PLACEMENT_3D('',#137733,#106012,#106013);
#95070=AXIS2_PLACEMENT_3D('',#137744,#106015,#106016);
#95071=AXIS2_PLACEMENT_3D('',#137755,#106018,#106019);
#95072=AXIS2_PLACEMENT_3D('',#137766,#106021,#106022);
#95073=AXIS2_PLACEMENT_3D('',#137777,#106024,#106025);
#95074=AXIS2_PLACEMENT_3D('',#137788,#106027,#106028);
#95075=AXIS2_PLACEMENT_3D('',#137799,#106030,#106031);
#95076=AXIS2_PLACEMENT_3D('',#137810,#106033,#106034);
#95077=AXIS2_PLACEMENT_3D('',#137820,#106036,#106037);
#95078=AXIS2_PLACEMENT_3D('',#137821,#106038,#106039);
#95079=AXIS2_PLACEMENT_3D('',#137837,#106043,#106044);
#95080=AXIS2_PLACEMENT_3D('',#137852,#106047,#106048);
#95081=AXIS2_PLACEMENT_3D('',#137854,#106050,#106051);
#95082=AXIS2_PLACEMENT_3D('',#137856,#106053,#106054);
#95083=AXIS2_PLACEMENT_3D('',#137858,#106056,#106057);
#95084=AXIS2_PLACEMENT_3D('',#137874,#106061,#106062);
#95085=AXIS2_PLACEMENT_3D('',#137889,#106065,#106066);
#95086=AXIS2_PLACEMENT_3D('',#137890,#106067,#106068);
#95087=AXIS2_PLACEMENT_3D('',#137892,#106070,#106071);
#95088=AXIS2_PLACEMENT_3D('',#137908,#106075,#106076);
#95089=AXIS2_PLACEMENT_3D('',#137923,#106079,#106080);
#95090=AXIS2_PLACEMENT_3D('',#137924,#106081,#106082);
#95091=AXIS2_PLACEMENT_3D('',#137926,#106084,#106085);
#95092=AXIS2_PLACEMENT_3D('',#137942,#106089,#106090);
#95093=AXIS2_PLACEMENT_3D('',#137957,#106093,#106094);
#95094=AXIS2_PLACEMENT_3D('',#137958,#106095,#106096);
#95095=AXIS2_PLACEMENT_3D('',#137960,#106098,#106099);
#95096=AXIS2_PLACEMENT_3D('',#137976,#106103,#106104);
#95097=AXIS2_PLACEMENT_3D('',#137991,#106107,#106108);
#95098=AXIS2_PLACEMENT_3D('',#137992,#106109,#106110);
#95099=AXIS2_PLACEMENT_3D('',#137994,#106112,#106113);
#95100=AXIS2_PLACEMENT_3D('',#138010,#106117,#106118);
#95101=AXIS2_PLACEMENT_3D('',#138025,#106121,#106122);
#95102=AXIS2_PLACEMENT_3D('',#138026,#106123,#106124);
#95103=AXIS2_PLACEMENT_3D('',#138028,#106126,#106127);
#95104=AXIS2_PLACEMENT_3D('',#138044,#106131,#106132);
#95105=AXIS2_PLACEMENT_3D('',#138059,#106135,#106136);
#95106=AXIS2_PLACEMENT_3D('',#138060,#106137,#106138);
#95107=AXIS2_PLACEMENT_3D('',#138062,#106140,#106141);
#95108=AXIS2_PLACEMENT_3D('',#138078,#106145,#106146);
#95109=AXIS2_PLACEMENT_3D('',#138093,#106149,#106150);
#95110=AXIS2_PLACEMENT_3D('',#138094,#106151,#106152);
#95111=AXIS2_PLACEMENT_3D('',#138096,#106154,#106155);
#95112=AXIS2_PLACEMENT_3D('',#138112,#106159,#106160);
#95113=AXIS2_PLACEMENT_3D('',#138127,#106163,#106164);
#95114=AXIS2_PLACEMENT_3D('',#138128,#106165,#106166);
#95115=AXIS2_PLACEMENT_3D('',#138130,#106168,#106169);
#95116=AXIS2_PLACEMENT_3D('',#138145,#106172,#106173);
#95117=AXIS2_PLACEMENT_3D('',#138160,#106176,#106177);
#95118=AXIS2_PLACEMENT_3D('',#138161,#106178,#106179);
#95119=AXIS2_PLACEMENT_3D('',#138164,#106180,#106181);
#95120=AXIS2_PLACEMENT_3D('',#138167,#106183,#106184);
#95121=AXIS2_PLACEMENT_3D('',#138168,#106185,#106186);
#95122=AXIS2_PLACEMENT_3D('',#138169,#106187,#106188);
#95123=AXIS2_PLACEMENT_3D('',#138172,#106189,#106190);
#95124=AXIS2_PLACEMENT_3D('',#138174,#106192,#106193);
#95125=AXIS2_PLACEMENT_3D('',#138175,#106194,#106195);
#95126=AXIS2_PLACEMENT_3D('',#138179,#106197,#106198);
#95127=AXIS2_PLACEMENT_3D('',#138180,#106199,#106200);
#95128=AXIS2_PLACEMENT_3D('',#138181,#106201,#106202);
#95129=AXIS2_PLACEMENT_3D('',#138183,#106204,#106205);
#95130=AXIS2_PLACEMENT_3D('',#138186,#106206,#106207);
#95131=AXIS2_PLACEMENT_3D('',#138189,#106209,#106210);
#95132=AXIS2_PLACEMENT_3D('',#138190,#106211,#106212);
#95133=AXIS2_PLACEMENT_3D('',#138191,#106213,#106214);
#95134=AXIS2_PLACEMENT_3D('',#138193,#106216,#106217);
#95135=AXIS2_PLACEMENT_3D('',#138197,#106219,#106220);
#95136=AXIS2_PLACEMENT_3D('',#138198,#106221,#106222);
#95137=AXIS2_PLACEMENT_3D('',#138199,#106223,#106224);
#95138=AXIS2_PLACEMENT_3D('',#138202,#106225,#106226);
#95139=AXIS2_PLACEMENT_3D('',#138205,#106228,#106229);
#95140=AXIS2_PLACEMENT_3D('',#138206,#106230,#106231);
#95141=AXIS2_PLACEMENT_3D('',#138207,#106232,#106233);
#95142=AXIS2_PLACEMENT_3D('',#138209,#106235,#106236);
#95143=AXIS2_PLACEMENT_3D('',#138213,#106238,#106239);
#95144=AXIS2_PLACEMENT_3D('',#138214,#106240,#106241);
#95145=AXIS2_PLACEMENT_3D('',#138215,#106242,#106243);
#95146=AXIS2_PLACEMENT_3D('',#138218,#106244,#106245);
#95147=AXIS2_PLACEMENT_3D('',#138221,#106247,#106248);
#95148=AXIS2_PLACEMENT_3D('',#138222,#106249,#106250);
#95149=AXIS2_PLACEMENT_3D('',#138223,#106251,#106252);
#95150=AXIS2_PLACEMENT_3D('',#138225,#106254,#106255);
#95151=AXIS2_PLACEMENT_3D('',#138229,#106257,#106258);
#95152=AXIS2_PLACEMENT_3D('',#138230,#106259,#106260);
#95153=AXIS2_PLACEMENT_3D('',#138231,#106261,#106262);
#95154=AXIS2_PLACEMENT_3D('',#138234,#106263,#106264);
#95155=AXIS2_PLACEMENT_3D('',#138237,#106266,#106267);
#95156=AXIS2_PLACEMENT_3D('',#138238,#106268,#106269);
#95157=AXIS2_PLACEMENT_3D('',#138239,#106270,#106271);
#95158=AXIS2_PLACEMENT_3D('',#138241,#106273,#106274);
#95159=AXIS2_PLACEMENT_3D('',#138245,#106276,#106277);
#95160=AXIS2_PLACEMENT_3D('',#138246,#106278,#106279);
#95161=AXIS2_PLACEMENT_3D('',#138247,#106280,#106281);
#95162=AXIS2_PLACEMENT_3D('',#138250,#106282,#106283);
#95163=AXIS2_PLACEMENT_3D('',#138253,#106285,#106286);
#95164=AXIS2_PLACEMENT_3D('',#138254,#106287,#106288);
#95165=AXIS2_PLACEMENT_3D('',#138255,#106289,#106290);
#95166=AXIS2_PLACEMENT_3D('',#138257,#106292,#106293);
#95167=AXIS2_PLACEMENT_3D('',#138261,#106295,#106296);
#95168=AXIS2_PLACEMENT_3D('',#138262,#106297,#106298);
#95169=AXIS2_PLACEMENT_3D('',#138263,#106299,#106300);
#95170=AXIS2_PLACEMENT_3D('',#138266,#106301,#106302);
#95171=AXIS2_PLACEMENT_3D('',#138269,#106304,#106305);
#95172=AXIS2_PLACEMENT_3D('',#138270,#106306,#106307);
#95173=AXIS2_PLACEMENT_3D('',#138271,#106308,#106309);
#95174=AXIS2_PLACEMENT_3D('',#138273,#106311,#106312);
#95175=AXIS2_PLACEMENT_3D('',#138277,#106314,#106315);
#95176=AXIS2_PLACEMENT_3D('',#138278,#106316,#106317);
#95177=AXIS2_PLACEMENT_3D('',#138279,#106318,#106319);
#95178=AXIS2_PLACEMENT_3D('',#138282,#106320,#106321);
#95179=AXIS2_PLACEMENT_3D('',#138285,#106323,#106324);
#95180=AXIS2_PLACEMENT_3D('',#138286,#106325,#106326);
#95181=AXIS2_PLACEMENT_3D('',#138287,#106327,#106328);
#95182=AXIS2_PLACEMENT_3D('',#138289,#106330,#106331);
#95183=AXIS2_PLACEMENT_3D('',#138293,#106333,#106334);
#95184=AXIS2_PLACEMENT_3D('',#138294,#106335,#106336);
#95185=AXIS2_PLACEMENT_3D('',#138295,#106337,#106338);
#95186=AXIS2_PLACEMENT_3D('',#138298,#106339,#106340);
#95187=AXIS2_PLACEMENT_3D('',#138301,#106342,#106343);
#95188=AXIS2_PLACEMENT_3D('',#138302,#106344,#106345);
#95189=AXIS2_PLACEMENT_3D('',#138303,#106346,#106347);
#95190=AXIS2_PLACEMENT_3D('',#138305,#106349,#106350);
#95191=AXIS2_PLACEMENT_3D('',#138309,#106352,#106353);
#95192=AXIS2_PLACEMENT_3D('',#138310,#106354,#106355);
#95193=AXIS2_PLACEMENT_3D('',#138311,#106356,#106357);
#95194=AXIS2_PLACEMENT_3D('',#138314,#106358,#106359);
#95195=AXIS2_PLACEMENT_3D('',#138317,#106361,#106362);
#95196=AXIS2_PLACEMENT_3D('',#138318,#106363,#106364);
#95197=AXIS2_PLACEMENT_3D('',#138319,#106365,#106366);
#95198=AXIS2_PLACEMENT_3D('',#138321,#106368,#106369);
#95199=AXIS2_PLACEMENT_3D('',#138325,#106371,#106372);
#95200=AXIS2_PLACEMENT_3D('',#138326,#106373,#106374);
#95201=AXIS2_PLACEMENT_3D('',#138327,#106375,#106376);
#95202=AXIS2_PLACEMENT_3D('',#138330,#106377,#106378);
#95203=AXIS2_PLACEMENT_3D('',#138333,#106380,#106381);
#95204=AXIS2_PLACEMENT_3D('',#138334,#106382,#106383);
#95205=AXIS2_PLACEMENT_3D('',#138335,#106384,#106385);
#95206=AXIS2_PLACEMENT_3D('',#138337,#106387,#106388);
#95207=AXIS2_PLACEMENT_3D('',#138341,#106390,#106391);
#95208=AXIS2_PLACEMENT_3D('',#138342,#106392,#106393);
#95209=AXIS2_PLACEMENT_3D('',#138343,#106394,#106395);
#95210=AXIS2_PLACEMENT_3D('',#138346,#106396,#106397);
#95211=AXIS2_PLACEMENT_3D('',#138349,#106399,#106400);
#95212=AXIS2_PLACEMENT_3D('',#138350,#106401,#106402);
#95213=AXIS2_PLACEMENT_3D('',#138351,#106403,#106404);
#95214=AXIS2_PLACEMENT_3D('',#138353,#106406,#106407);
#95215=AXIS2_PLACEMENT_3D('',#138357,#106409,#106410);
#95216=AXIS2_PLACEMENT_3D('',#138358,#106411,#106412);
#95217=AXIS2_PLACEMENT_3D('',#138359,#106413,#106414);
#95218=AXIS2_PLACEMENT_3D('',#138362,#106415,#106416);
#95219=AXIS2_PLACEMENT_3D('',#138365,#106418,#106419);
#95220=AXIS2_PLACEMENT_3D('',#138366,#106420,#106421);
#95221=AXIS2_PLACEMENT_3D('',#138367,#106422,#106423);
#95222=AXIS2_PLACEMENT_3D('',#138369,#106425,#106426);
#95223=AXIS2_PLACEMENT_3D('',#138373,#106428,#106429);
#95224=AXIS2_PLACEMENT_3D('',#138374,#106430,#106431);
#95225=AXIS2_PLACEMENT_3D('',#138375,#106432,#106433);
#95226=AXIS2_PLACEMENT_3D('',#138378,#106434,#106435);
#95227=AXIS2_PLACEMENT_3D('',#138381,#106437,#106438);
#95228=AXIS2_PLACEMENT_3D('',#138382,#106439,#106440);
#95229=AXIS2_PLACEMENT_3D('',#138383,#106441,#106442);
#95230=AXIS2_PLACEMENT_3D('',#138385,#106444,#106445);
#95231=AXIS2_PLACEMENT_3D('',#138386,#106446,#106447);
#95232=AXIS2_PLACEMENT_3D('',#138390,#106449,#106450);
#95233=AXIS2_PLACEMENT_3D('',#138391,#106451,#106452);
#95234=AXIS2_PLACEMENT_3D('',#138392,#106453,#106454);
#95235=AXIS2_PLACEMENT_3D('',#138395,#106455,#106456);
#95236=AXIS2_PLACEMENT_3D('',#138396,#106457,#106458);
#95237=AXIS2_PLACEMENT_3D('',#138399,#106460,#106461);
#95238=AXIS2_PLACEMENT_3D('',#138400,#106462,#106463);
#95239=AXIS2_PLACEMENT_3D('',#138402,#106465,#106466);
#95240=AXIS2_PLACEMENT_3D('',#138404,#106468,#106469);
#95241=AXIS2_PLACEMENT_3D('',#138406,#106471,#106472);
#95242=AXIS2_PLACEMENT_3D('',#138407,#106473,#106474);
#105579=DIRECTION('axis',(0.,0.,1.));
#105580=DIRECTION('refdir',(1.,0.,0.));
#105581=DIRECTION('center_axis',(4.93038065763132E-32,1.97215226305253E-31,
-1.));
#105582=DIRECTION('ref_axis',(-0.348448562526685,0.937327903816528,1.67675494144795E-31));
#105583=DIRECTION('',(4.93038065763132E-32,1.97215226305253E-31,-1.));
#105584=DIRECTION('center_axis',(4.93038065763132E-32,1.97215226305253E-31,
-1.));
#105585=DIRECTION('ref_axis',(1.,0.,4.93038065763132E-32));
#105586=DIRECTION('center_axis',(4.93038065763132E-32,1.97215226305253E-31,
-1.));
#105587=DIRECTION('ref_axis',(-0.348448562526685,0.937327903816528,1.67675494144795E-31));
#105588=DIRECTION('',(4.93038065763132E-32,1.97215226305253E-31,-1.));
#105589=DIRECTION('center_axis',(4.93038065763132E-32,1.97215226305253E-31,
-1.));
#105590=DIRECTION('ref_axis',(-0.348448562526685,0.937327903816528,1.67675494144795E-31));
#105591=DIRECTION('',(4.93038065763132E-32,1.97215226305253E-31,-1.));
#105592=DIRECTION('center_axis',(4.93038065763132E-32,1.97215226305253E-31,
-1.));
#105593=DIRECTION('ref_axis',(-0.348448562526685,0.937327903816528,1.67675494144795E-31));
#105594=DIRECTION('',(4.93038065763132E-32,1.97215226305253E-31,-1.));
#105595=DIRECTION('center_axis',(4.93038065763132E-32,1.97215226305253E-31,
-1.));
#105596=DIRECTION('ref_axis',(1.,0.,4.93038065763132E-32));
#105597=DIRECTION('center_axis',(4.93038065763132E-32,1.97215226305253E-31,
-1.));
#105598=DIRECTION('ref_axis',(-0.348448196221629,0.937328039989145,1.67675539060342E-31));
#105599=DIRECTION('',(4.93038065763132E-32,1.97215226305253E-31,-1.));
#105600=DIRECTION('center_axis',(4.93038065763132E-32,1.97215226305253E-31,
-1.));
#105601=DIRECTION('ref_axis',(1.,0.,4.93038065763132E-32));
#105602=DIRECTION('center_axis',(4.93038065763132E-32,1.97215226305253E-31,
-1.));
#105603=DIRECTION('ref_axis',(-0.348448196221629,0.937328039989145,1.67675539060342E-31));
#105604=DIRECTION('',(4.93038065763132E-32,1.97215226305253E-31,-1.));
#105605=DIRECTION('center_axis',(4.93038065763132E-32,1.97215226305253E-31,
-1.));
#105606=DIRECTION('ref_axis',(-0.348448196221629,0.937328039989145,1.67675539060342E-31));
#105607=DIRECTION('',(4.93038065763132E-32,1.97215226305253E-31,-1.));
#105608=DIRECTION('center_axis',(4.93038065763132E-32,1.97215226305253E-31,
-1.));
#105609=DIRECTION('ref_axis',(-0.348448196221629,0.937328039989145,1.67675539060342E-31));
#105610=DIRECTION('',(4.93038065763132E-32,1.97215226305253E-31,-1.));
#105611=DIRECTION('center_axis',(4.93038065763132E-32,1.97215226305253E-31,
-1.));
#105612=DIRECTION('ref_axis',(1.,0.,4.93038065763132E-32));
#105613=DIRECTION('center_axis',(4.93038065763132E-32,1.97215226305253E-31,
-1.));
#105614=DIRECTION('ref_axis',(-0.608873383780016,-0.793267421822095,-1.86464189658584E-31));
#105615=DIRECTION('',(4.93038065763132E-32,1.97215226305253E-31,-1.));
#105616=DIRECTION('center_axis',(-4.93038065763132E-32,-1.97215226305253E-31,
1.));
#105617=DIRECTION('ref_axis',(1.,5.75617900000082E-15,4.93038065763144E-32));
#105618=DIRECTION('center_axis',(4.93038065763132E-32,1.97215226305253E-31,
-1.));
#105619=DIRECTION('ref_axis',(-0.608873383780016,-0.793267421822095,-1.86464189658584E-31));
#105620=DIRECTION('',(4.93038065763132E-32,1.97215226305253E-31,-1.));
#105621=DIRECTION('center_axis',(4.93038065763132E-32,1.97215226305253E-31,
-1.));
#105622=DIRECTION('ref_axis',(-0.608873383780016,-0.793267421822095,-1.86464189658584E-31));
#105623=DIRECTION('',(4.93038065763132E-32,1.97215226305253E-31,-1.));
#105624=DIRECTION('center_axis',(4.93038065763132E-32,1.97215226305253E-31,
-1.));
#105625=DIRECTION('ref_axis',(-0.608873383780016,-0.793267421822095,-1.86464189658584E-31));
#105626=DIRECTION('',(4.93038065763132E-32,1.97215226305253E-31,-1.));
#105627=DIRECTION('center_axis',(4.93038065763132E-32,1.97215226305253E-31,
-1.));
#105628=DIRECTION('ref_axis',(1.,5.75617900000082E-15,4.93038065763144E-32));
#105629=DIRECTION('center_axis',(4.93038065763132E-32,1.97215226305253E-31,
-1.));
#105630=DIRECTION('ref_axis',(-0.608873392866957,-0.793267414847402,-1.86464188731089E-31));
#105631=DIRECTION('',(4.93038065763132E-32,1.97215226305253E-31,-1.));
#105632=DIRECTION('center_axis',(-4.93038065763132E-32,-1.97215226305253E-31,
1.));
#105633=DIRECTION('ref_axis',(1.,8.63426850000124E-15,4.93038065763149E-32));
#105634=DIRECTION('center_axis',(4.93038065763132E-32,1.97215226305253E-31,
-1.));
#105635=DIRECTION('ref_axis',(-0.608873392866957,-0.793267414847402,-1.86464188731089E-31));
#105636=DIRECTION('',(4.93038065763132E-32,1.97215226305253E-31,-1.));
#105637=DIRECTION('center_axis',(4.93038065763132E-32,1.97215226305253E-31,
-1.));
#105638=DIRECTION('ref_axis',(-0.608873392866957,-0.793267414847402,-1.86464188731089E-31));
#105639=DIRECTION('',(4.93038065763132E-32,1.97215226305253E-31,-1.));
#105640=DIRECTION('center_axis',(4.93038065763132E-32,1.97215226305253E-31,
-1.));
#105641=DIRECTION('ref_axis',(-0.608873392866957,-0.793267414847402,-1.86464188731089E-31));
#105642=DIRECTION('',(4.93038065763132E-32,1.97215226305253E-31,-1.));
#105643=DIRECTION('center_axis',(4.93038065763132E-32,1.97215226305253E-31,
-1.));
#105644=DIRECTION('ref_axis',(1.,8.63426850000124E-15,4.93038065763149E-32));
#105645=DIRECTION('center_axis',(4.93038065763132E-32,1.97215226305253E-31,
-1.));
#105646=DIRECTION('ref_axis',(-0.608873392866957,-0.793267414847402,-1.86464188731089E-31));
#105647=DIRECTION('center_axis',(4.93038065763132E-32,1.97215226305253E-31,
-1.));
#105648=DIRECTION('ref_axis',(-0.608873383780016,-0.793267421822095,-1.86464189658584E-31));
#105649=DIRECTION('center_axis',(4.93038065763132E-32,1.97215226305253E-31,
-1.));
#105650=DIRECTION('ref_axis',(-0.348448196221629,0.937328039989145,1.67675539060342E-31));
#105651=DIRECTION('center_axis',(4.93038065763132E-32,1.97215226305253E-31,
-1.));
#105652=DIRECTION('ref_axis',(-0.348448562526685,0.937327903816528,1.67675494144795E-31));
#105653=DIRECTION('center_axis',(4.93038065763132E-32,1.97215226305253E-31,
-1.));
#105654=DIRECTION('ref_axis',(-1.,0.,-4.93038065763132E-32));
#105655=DIRECTION('center_axis',(4.93038065763132E-32,1.97215226305253E-31,
-1.));
#105656=DIRECTION('ref_axis',(0.731712168750195,0.681613748469679,1.70500804894814E-31));
#105657=DIRECTION('',(0.909673749800079,-0.415323571356916,-3.70577535073674E-32));
#105658=DIRECTION('center_axis',(-4.93038065763132E-32,-1.97215226305253E-31,
1.));
#105659=DIRECTION('ref_axis',(-0.415323571356918,-0.909673749800078,-1.99878547459536E-31));
#105660=DIRECTION('',(-0.909673749800079,-0.415323571356916,-1.26758510722753E-31));
#105661=DIRECTION('center_axis',(4.93038065763132E-32,1.97215226305253E-31,
-1.));
#105662=DIRECTION('ref_axis',(0.731712168750193,-0.681613748469681,-9.83484144196257E-32));
#105663=DIRECTION('center_axis',(4.93038065763132E-32,1.97215226305253E-31,
-1.));
#105664=DIRECTION('ref_axis',(-1.,0.,-4.93038065763132E-32));
#105665=DIRECTION('center_axis',(4.93038065763132E-32,1.97215226305253E-31,
-1.));
#105666=DIRECTION('ref_axis',(-1.,0.,-4.93038065763132E-32));
#105667=DIRECTION('center_axis',(4.93038065763132E-32,1.97215226305253E-31,
-1.));
#105668=DIRECTION('ref_axis',(-0.731712168808585,-0.681613748406997,-1.70500804885331E-31));
#105669=DIRECTION('',(-0.909673749731055,0.415323571508098,3.70577535405859E-32));
#105670=DIRECTION('center_axis',(-4.93038065763132E-32,-1.97215226305253E-31,
1.));
#105671=DIRECTION('ref_axis',(0.415323571508097,0.909673749731055,1.99878547453377E-31));
#105672=DIRECTION('',(0.909673749731055,0.415323571508098,1.26758510749165E-31));
#105673=DIRECTION('center_axis',(4.93038065763132E-32,1.97215226305253E-31,
-1.));
#105674=DIRECTION('ref_axis',(-0.731712168808585,0.681613748406997,9.83484144043845E-32));
#105675=DIRECTION('center_axis',(4.93038065763132E-32,1.97215226305253E-31,
-1.));
#105676=DIRECTION('ref_axis',(-1.,0.,-4.93038065763132E-32));
#105677=DIRECTION('center_axis',(4.93038065763132E-32,1.97215226305253E-31,
-1.));
#105678=DIRECTION('ref_axis',(-1.,0.,-4.93038065763132E-32));
#105679=DIRECTION('center_axis',(4.93038065763132E-32,1.97215226305253E-31,
-1.));
#105680=DIRECTION('ref_axis',(-1.,0.,-4.93038065763132E-32));
#105681=DIRECTION('center_axis',(-4.93038065763132E-32,-1.97215226305253E-31,
1.));
#105682=DIRECTION('ref_axis',(-1.,0.,-4.93038065763132E-32));
#105683=DIRECTION('',(-0.707106781186547,8.65956056235491E-17,0.707106781186548));
#105684=DIRECTION('center_axis',(4.93038065763132E-32,1.97215226305253E-31,
-1.));
#105685=DIRECTION('ref_axis',(-1.,0.,-4.93038065763132E-32));
#105686=DIRECTION('center_axis',(-4.93038065763132E-32,-1.97215226305253E-31,
1.));
#105687=DIRECTION('ref_axis',(-1.,0.,-4.93038065763132E-32));
#105688=DIRECTION('',(4.93038065763132E-32,1.97215226305253E-31,-1.));
#105689=DIRECTION('center_axis',(4.93038065763132E-32,1.97215226305253E-31,
-1.));
#105690=DIRECTION('ref_axis',(-1.,0.,-4.93038065763132E-32));
#105691=DIRECTION('center_axis',(4.93038065763132E-32,1.97215226305253E-31,
-1.));
#105692=DIRECTION('ref_axis',(-1.,0.,-4.93038065763132E-32));
#105693=DIRECTION('center_axis',(4.93038065763132E-32,1.97215226305253E-31,
-1.));
#105694=DIRECTION('ref_axis',(1.,0.,4.93038065763132E-32));
#105695=DIRECTION('center_axis',(-4.93038065763132E-32,-1.97215226305253E-31,
1.));
#105696=DIRECTION('ref_axis',(1.,0.,4.93038065763132E-32));
#105697=DIRECTION('center_axis',(4.93038065763132E-32,1.97215226305253E-31,
-1.));
#105698=DIRECTION('ref_axis',(1.,0.,4.93038065763132E-32));
#105699=DIRECTION('',(0.707106781186547,8.65956056235494E-17,-0.707106781186548));
#105700=DIRECTION('center_axis',(-4.93038065763132E-32,-1.97215226305253E-31,
1.));
#105701=DIRECTION('ref_axis',(1.,0.,4.93038065763132E-32));
#105702=DIRECTION('center_axis',(4.93038065763132E-32,1.97215226305253E-31,
-1.));
#105703=DIRECTION('ref_axis',(1.,0.,4.93038065763132E-32));
#105704=DIRECTION('center_axis',(4.93038065763132E-32,1.97215226305253E-31,
-1.));
#105705=DIRECTION('ref_axis',(-1.,0.,-4.93038065763132E-32));
#105706=DIRECTION('',(-4.93038065763132E-32,-1.97215226305253E-31,1.));
#105707=DIRECTION('',(4.93038065763132E-32,1.97215226305253E-31,-1.));
#105708=DIRECTION('center_axis',(-4.93038065763132E-32,-1.97215226305253E-31,
1.));
#105709=DIRECTION('ref_axis',(-1.,0.,-4.93038065763132E-32));
#105710=DIRECTION('',(-4.93038065763132E-32,-1.97215226305253E-31,1.));
#105711=DIRECTION('',(4.93038065763132E-32,1.97215226305253E-31,-1.));
#105712=DIRECTION('center_axis',(-4.93038065763132E-32,-1.97215226305253E-31,
1.));
#105713=DIRECTION('ref_axis',(-1.,0.,-4.93038065763132E-32));
#105714=DIRECTION('',(-4.93038065763132E-32,-1.97215226305253E-31,1.));
#105715=DIRECTION('center_axis',(-4.93038065763132E-32,-1.97215226305253E-31,
1.));
#105716=DIRECTION('ref_axis',(1.,0.,4.93038065763132E-32));
#105717=DIRECTION('center_axis',(4.93038065763132E-32,1.97215226305253E-31,
-1.));
#105718=DIRECTION('ref_axis',(1.,0.,4.93038065763132E-32));
#105719=DIRECTION('center_axis',(4.93038065763132E-32,1.97215226305253E-31,
-1.));
#105720=DIRECTION('ref_axis',(1.,0.,4.93038065763132E-32));
#105721=DIRECTION('center_axis',(-4.93038065763132E-32,-1.97215226305253E-31,
1.));
#105722=DIRECTION('ref_axis',(1.,0.,4.93038065763132E-32));
#105723=DIRECTION('',(0.707106781186539,-8.65956056235485E-17,0.707106781186556));
#105724=DIRECTION('center_axis',(4.93038065763132E-32,1.97215226305253E-31,
-1.));
#105725=DIRECTION('ref_axis',(1.,0.,4.93038065763132E-32));
#105726=DIRECTION('center_axis',(-4.93038065763132E-32,-1.97215226305253E-31,
1.));
#105727=DIRECTION('ref_axis',(1.,0.,4.93038065763132E-32));
#105728=DIRECTION('center_axis',(4.93038065763132E-32,1.97215226305253E-31,
-1.));
#105729=DIRECTION('ref_axis',(-1.,0.,-4.93038065763132E-32));
#105730=DIRECTION('center_axis',(4.93038065763132E-32,1.97215226305253E-31,
-1.));
#105731=DIRECTION('ref_axis',(-1.,0.,-4.93038065763132E-32));
#105732=DIRECTION('',(-4.93038065763132E-32,-1.97215226305253E-31,1.));
#105733=DIRECTION('center_axis',(-4.93038065763132E-32,-1.97215226305253E-31,
1.));
#105734=DIRECTION('ref_axis',(1.,0.,4.93038065763132E-32));
#105735=DIRECTION('center_axis',(-4.93038065763132E-32,-1.97215226305253E-31,
1.));
#105736=DIRECTION('ref_axis',(1.,0.,4.93038065763132E-32));
#105737=DIRECTION('center_axis',(4.93038065763132E-32,1.97215226305253E-31,
-1.));
#105738=DIRECTION('ref_axis',(1.,0.,4.93038065763132E-32));
#105739=DIRECTION('center_axis',(-4.93038065763132E-32,-1.97215226305253E-31,
1.));
#105740=DIRECTION('ref_axis',(1.,0.,4.93038065763132E-32));
#105741=DIRECTION('',(-0.707106781186555,8.65956056235504E-17,-0.70710678118654));
#105742=DIRECTION('center_axis',(4.93038065763132E-32,1.97215226305253E-31,
-1.));
#105743=DIRECTION('ref_axis',(1.,0.,4.93038065763132E-32));
#105744=DIRECTION('center_axis',(4.93038065763132E-32,1.97215226305253E-31,
-1.));
#105745=DIRECTION('ref_axis',(-1.,0.,-4.93038065763132E-32));
#105746=DIRECTION('center_axis',(-4.93038065763132E-32,-1.97215226305253E-31,
1.));
#105747=DIRECTION('ref_axis',(-1.,0.,-4.93038065763132E-32));
#105748=DIRECTION('center_axis',(-4.93038065763132E-32,-1.97215226305253E-31,
1.));
#105749=DIRECTION('ref_axis',(1.,0.,4.93038065763132E-32));
#105750=DIRECTION('',(-4.93038065763132E-32,-1.97215226305253E-31,1.));
#105751=DIRECTION('center_axis',(-4.93038065763132E-32,-1.97215226305253E-31,
1.));
#105752=DIRECTION('ref_axis',(1.,0.,4.93038065763132E-32));
#105753=DIRECTION('center_axis',(-4.93038065763132E-32,-1.97215226305253E-31,
1.));
#105754=DIRECTION('ref_axis',(-1.,0.,-4.93038065763132E-32));
#105755=DIRECTION('',(-0.707106781186555,-8.65956056235501E-17,-0.70710678118654));
#105756=DIRECTION('center_axis',(4.93038065763132E-32,1.97215226305253E-31,
-1.));
#105757=DIRECTION('ref_axis',(0.731712168750192,-0.681613748469681,-9.83484144196258E-32));
#105758=DIRECTION('',(-0.293678113693067,0.643236477151022,0.707106781186565));
#105759=DIRECTION('center_axis',(-4.93038065763132E-32,-1.97215226305253E-31,
1.));
#105760=DIRECTION('ref_axis',(0.731712168750192,-0.681613748469682,-9.83484144196259E-32));
#105761=DIRECTION('center_axis',(-0.293678113693089,0.643236477151028,-0.707106781186551));
#105762=DIRECTION('ref_axis',(-0.923516686410398,2.4980018054066E-16,0.383558248407668));
#105763=DIRECTION('',(-0.29367811369309,0.643236477151034,0.707106781186544));
#105764=DIRECTION('',(0.909673749800079,0.415323571356916,1.26758510722753E-31));
#105765=DIRECTION('center_axis',(-4.93038065763132E-32,-1.97215226305253E-31,
1.));
#105766=DIRECTION('ref_axis',(-0.415323571356918,-0.909673749800078,-1.99878547459536E-31));
#105767=DIRECTION('',(-0.29367811369309,-0.643236477151034,0.707106781186544));
#105768=DIRECTION('center_axis',(4.93038065763132E-32,1.97215226305253E-31,
-1.));
#105769=DIRECTION('ref_axis',(-0.415323571356918,-0.909673749800078,-1.99878547459536E-31));
#105770=DIRECTION('center_axis',(-0.293678113693089,-0.643236477151028,
-0.707106781186551));
#105771=DIRECTION('ref_axis',(-0.923516686410398,-2.4980018054066E-16,0.383558248407668));
#105772=DIRECTION('',(-0.293678113693093,-0.643236477151025,0.707106781186552));
#105773=DIRECTION('',(-0.909673749800079,0.415323571356916,3.70577535073674E-32));
#105774=DIRECTION('center_axis',(4.93038065763132E-32,1.97215226305253E-31,
-1.));
#105775=DIRECTION('ref_axis',(0.731712168750195,0.681613748469679,1.70500804894814E-31));
#105776=DIRECTION('center_axis',(-4.93038065763132E-32,-1.97215226305253E-31,
1.));
#105777=DIRECTION('ref_axis',(0.731712168750195,0.681613748469679,1.70500804894814E-31));
#105778=DIRECTION('center_axis',(4.93038065763132E-32,1.97215226305253E-31,
-1.));
#105779=DIRECTION('ref_axis',(-0.731712168808585,0.681613748406997,9.83484144043845E-32));
#105780=DIRECTION('',(0.293678113799996,-0.643236477102231,0.707106781186539));
#105781=DIRECTION('center_axis',(-4.93038065763132E-32,-1.97215226305253E-31,
1.));
#105782=DIRECTION('ref_axis',(-0.731712168808585,0.681613748406997,9.83484144043845E-32));
#105783=DIRECTION('center_axis',(0.293678113799993,-0.643236477102225,-0.707106781186545));
#105784=DIRECTION('ref_axis',(-0.92351668636094,-5.55111512312577E-17,-0.383558248526752));
#105785=DIRECTION('',(0.293678113799987,-0.643236477102215,0.707106781186557));
#105786=DIRECTION('',(-0.909673749731055,-0.415323571508098,-1.26758510749165E-31));
#105787=DIRECTION('center_axis',(-4.93038065763132E-32,-1.97215226305253E-31,
1.));
#105788=DIRECTION('ref_axis',(0.415323571508097,0.909673749731055,1.99878547453377E-31));
#105789=DIRECTION('',(0.293678113799987,0.643236477102215,0.707106781186557));
#105790=DIRECTION('center_axis',(4.93038065763132E-32,1.97215226305253E-31,
-1.));
#105791=DIRECTION('ref_axis',(0.415323571508097,0.909673749731055,1.99878547453377E-31));
#105792=DIRECTION('center_axis',(0.293678113799988,0.643236477102216,-0.707106781186556));
#105793=DIRECTION('ref_axis',(-0.923516686360944,-5.27355936696949E-16,
-0.383558248526742));
#105794=DIRECTION('',(0.293678113799996,0.643236477102231,0.707106781186539));
#105795=DIRECTION('',(0.909673749731055,-0.415323571508098,-3.70577535405859E-32));
#105796=DIRECTION('center_axis',(4.93038065763132E-32,1.97215226305253E-31,
-1.));
#105797=DIRECTION('ref_axis',(-0.731712168808585,-0.681613748406997,-1.70500804885331E-31));
#105798=DIRECTION('center_axis',(-4.93038065763132E-32,-1.97215226305253E-31,
1.));
#105799=DIRECTION('ref_axis',(-0.731712168808585,-0.681613748406997,-1.70500804885331E-31));
#105800=DIRECTION('center_axis',(0.293678113799996,0.643236477102232,0.707106781186538));
#105801=DIRECTION('ref_axis',(0.923516686360937,-4.44089209850063E-16,-0.383558248526758));
#105802=DIRECTION('',(0.293678113799987,0.643236477102215,-0.707106781186557));
#105803=DIRECTION('',(-0.909673749731055,0.415323571508098,3.70577535405859E-32));
#105804=DIRECTION('',(-0.293678113799987,-0.643236477102215,0.707106781186557));
#105805=DIRECTION('',(0.909673749731055,-0.415323571508098,-3.70577535405859E-32));
#105806=DIRECTION('center_axis',(4.93038065763132E-32,1.97215226305253E-31,
-1.));
#105807=DIRECTION('ref_axis',(0.415323571508097,0.909673749731055,1.99878547453377E-31));
#105808=DIRECTION('',(0.29367811380001,-0.643236477102228,-0.707106781186536));
#105809=DIRECTION('center_axis',(-4.93038065763132E-32,-1.97215226305253E-31,
1.));
#105810=DIRECTION('ref_axis',(0.415323571508097,0.909673749731055,1.99878547453377E-31));
#105811=DIRECTION('center_axis',(4.93038065763132E-32,1.97215226305253E-31,
-1.));
#105812=DIRECTION('ref_axis',(0.415323571508097,0.909673749731055,1.99878547453377E-31));
#105813=DIRECTION('center_axis',(0.293678113799988,-0.643236477102216,0.707106781186556));
#105814=DIRECTION('ref_axis',(0.923516686360944,-5.27355936696949E-16,-0.383558248526742));
#105815=DIRECTION('',(0.293678113799996,-0.643236477102231,-0.707106781186539));
#105816=DIRECTION('',(0.909673749731055,0.415323571508098,1.26758510749165E-31));
#105817=DIRECTION('',(-0.909673749731055,-0.415323571508098,-1.26758510749165E-31));
#105818=DIRECTION('center_axis',(-4.93038065763132E-32,-1.97215226305253E-31,
1.));
#105819=DIRECTION('ref_axis',(-0.731712168808585,0.681613748406997,9.83484144043845E-32));
#105820=DIRECTION('',(0.662416044053367,-0.247396411818533,-0.707106781186549));
#105821=DIRECTION('center_axis',(4.93038065763132E-32,1.97215226305253E-31,
-1.));
#105822=DIRECTION('ref_axis',(-0.731712168808585,0.681613748406997,9.83484144043845E-32));
#105823=DIRECTION('center_axis',(-4.93038065763132E-32,-1.97215226305253E-31,
1.));
#105824=DIRECTION('ref_axis',(-0.731712168808585,0.681613748406997,9.83484144043845E-32));
#105825=DIRECTION('center_axis',(4.93038065763132E-32,1.97215226305253E-31,
-1.));
#105826=DIRECTION('ref_axis',(-1.,0.,-4.93038065763132E-32));
#105827=DIRECTION('',(-0.662416044052087,-0.247396411821942,-0.707106781186556));
#105828=DIRECTION('center_axis',(4.93038065763132E-32,1.97215226305253E-31,
-1.));
#105829=DIRECTION('ref_axis',(-1.,0.,-4.93038065763132E-32));
#105830=DIRECTION('center_axis',(-4.93038065763132E-32,-1.97215226305253E-31,
1.));
#105831=DIRECTION('ref_axis',(0.731712168750195,0.681613748469679,1.70500804894814E-31));
#105832=DIRECTION('',(-0.293678113693076,-0.643236477151037,-0.707106781186548));
#105833=DIRECTION('center_axis',(4.93038065763132E-32,1.97215226305253E-31,
-1.));
#105834=DIRECTION('ref_axis',(0.731712168750195,0.681613748469679,1.70500804894814E-31));
#105835=DIRECTION('center_axis',(-4.93038065763132E-32,-1.97215226305253E-31,
1.));
#105836=DIRECTION('ref_axis',(0.731712168750195,0.681613748469679,1.70500804894814E-31));
#105837=DIRECTION('center_axis',(-0.293678113693092,-0.643236477151034,
0.707106781186543));
#105838=DIRECTION('ref_axis',(0.923516686410395,-7.5643526760966E-32,0.383558248407675));
#105839=DIRECTION('',(-0.909673749800079,0.415323571356916,3.70577535073674E-32));
#105840=DIRECTION('',(-0.29367811369309,-0.643236477151034,-0.707106781186544));
#105841=DIRECTION('',(0.909673749800079,-0.415323571356916,-3.70577535073674E-32));
#105842=DIRECTION('center_axis',(4.93038065763132E-32,1.97215226305253E-31,
-1.));
#105843=DIRECTION('ref_axis',(-0.415323571356918,-0.909673749800078,-1.99878547459536E-31));
#105844=DIRECTION('',(-0.29367811369309,0.643236477151034,-0.707106781186544));
#105845=DIRECTION('center_axis',(-4.93038065763132E-32,-1.97215226305253E-31,
1.));
#105846=DIRECTION('ref_axis',(-0.415323571356918,-0.909673749800078,-1.99878547459536E-31));
#105847=DIRECTION('center_axis',(4.93038065763132E-32,1.97215226305253E-31,
-1.));
#105848=DIRECTION('ref_axis',(-0.415323571356918,-0.909673749800078,-1.99878547459536E-31));
#105849=DIRECTION('center_axis',(-0.293678113693089,0.643236477151028,0.707106781186551));
#105850=DIRECTION('ref_axis',(0.923516686410398,-2.4980018054066E-16,0.383558248407668));
#105851=DIRECTION('',(0.909673749800079,0.415323571356916,1.26758510722753E-31));
#105852=DIRECTION('',(-0.29367811369309,0.643236477151034,-0.707106781186544));
#105853=DIRECTION('',(-0.909673749800079,-0.415323571356916,-1.26758510722753E-31));
#105854=DIRECTION('center_axis',(-4.93038065763132E-32,-1.97215226305253E-31,
1.));
#105855=DIRECTION('ref_axis',(0.731712168750192,-0.681613748469681,-9.83484144196258E-32));
#105856=DIRECTION('',(-0.662416044052087,0.247396411821942,-0.707106781186556));
#105857=DIRECTION('center_axis',(4.93038065763132E-32,1.97215226305253E-31,
-1.));
#105858=DIRECTION('ref_axis',(0.731712168750192,-0.681613748469682,-9.83484144196259E-32));
#105859=DIRECTION('center_axis',(-4.93038065763132E-32,-1.97215226305253E-31,
1.));
#105860=DIRECTION('ref_axis',(0.731712168750193,-0.681613748469681,-9.83484144196257E-32));
#105861=DIRECTION('center_axis',(4.93038065763132E-32,1.97215226305253E-31,
-1.));
#105862=DIRECTION('ref_axis',(-1.,0.,-4.93038065763132E-32));
#105863=DIRECTION('',(0.662416044053361,0.247396411818521,-0.707106781186559));
#105864=DIRECTION('center_axis',(4.93038065763132E-32,1.97215226305253E-31,
-1.));
#105865=DIRECTION('ref_axis',(-1.,0.,-4.93038065763132E-32));
#105866=DIRECTION('center_axis',(-4.93038065763132E-32,-1.97215226305253E-31,
1.));
#105867=DIRECTION('ref_axis',(-0.731712168808585,-0.681613748406997,-1.70500804885331E-31));
#105868=DIRECTION('center_axis',(4.93038065763132E-32,1.97215226305253E-31,
-1.));
#105869=DIRECTION('ref_axis',(-0.731712168808585,-0.681613748406997,-1.70500804885331E-31));
#105870=DIRECTION('center_axis',(-4.93038065763132E-32,-1.97215226305253E-31,
1.));
#105871=DIRECTION('ref_axis',(-0.731712168808585,-0.681613748406997,-1.70500804885331E-31));
#105872=DIRECTION('center_axis',(4.93038065763132E-32,1.97215226305253E-31,
-1.));
#105873=DIRECTION('ref_axis',(-0.415323571356918,-0.909673749800078,-1.99878547459536E-31));
#105874=DIRECTION('',(4.93038065763132E-32,1.97215226305253E-31,-1.));
#105875=DIRECTION('',(4.93038065763132E-32,1.97215226305253E-31,-1.));
#105876=DIRECTION('center_axis',(-0.415323571356916,0.909673749800079,1.58924481402006E-31));
#105877=DIRECTION('ref_axis',(0.909673749800079,0.415323571356916,1.26758510722753E-31));
#105878=DIRECTION('',(-4.93038065763132E-32,-1.97215226305253E-31,1.));
#105879=DIRECTION('center_axis',(-4.93038065763132E-32,-1.97215226305253E-31,
1.));
#105880=DIRECTION('ref_axis',(0.731712168750192,-0.681613748469682,-9.83484144196259E-32));
#105881=DIRECTION('center_axis',(4.93038065763132E-32,1.97215226305253E-31,
-1.));
#105882=DIRECTION('ref_axis',(-0.731712168808585,-0.681613748406997,-1.70500804885331E-31));
#105883=DIRECTION('',(4.93038065763132E-32,1.97215226305253E-31,-1.));
#105884=DIRECTION('center_axis',(0.415323571508098,0.909673749731055,1.99878547453377E-31));
#105885=DIRECTION('ref_axis',(0.909673749731055,-0.415323571508098,-3.70577535405859E-32));
#105886=DIRECTION('',(4.93038065763132E-32,1.97215226305253E-31,-1.));
#105887=DIRECTION('center_axis',(4.93038065763132E-32,1.97215226305253E-31,
-1.));
#105888=DIRECTION('ref_axis',(-1.,0.,-4.93038065763132E-32));
#105889=DIRECTION('center_axis',(4.93038065763132E-32,1.97215226305253E-31,
-1.));
#105890=DIRECTION('ref_axis',(0.731712168750195,0.681613748469679,1.70500804894814E-31));
#105891=DIRECTION('',(4.93038065763132E-32,1.97215226305253E-31,-1.));
#105892=DIRECTION('center_axis',(-4.93038065763132E-32,-1.97215226305253E-31,
1.));
#105893=DIRECTION('ref_axis',(-0.731712168808585,0.681613748406997,9.83484144043845E-32));
#105894=DIRECTION('',(-4.93038065763132E-32,-1.97215226305253E-31,1.));
#105895=DIRECTION('center_axis',(0.415323571508098,-0.909673749731055,-1.58924481380939E-31));
#105896=DIRECTION('ref_axis',(-0.909673749731055,-0.415323571508098,-1.26758510749165E-31));
#105897=DIRECTION('',(4.93038065763132E-32,1.97215226305253E-31,-1.));
#105898=DIRECTION('center_axis',(-4.93038065763132E-32,-1.97215226305253E-31,
1.));
#105899=DIRECTION('ref_axis',(1.,0.,4.93038065763132E-32));
#105900=DIRECTION('center_axis',(4.93038065763132E-32,1.97215226305253E-31,
-1.));
#105901=DIRECTION('ref_axis',(1.,0.,4.93038065763132E-32));
#105902=DIRECTION('',(-0.707106781186547,-8.65956056235494E-17,0.707106781186548));
#105903=DIRECTION('center_axis',(-4.93038065763132E-32,-1.97215226305253E-31,
1.));
#105904=DIRECTION('ref_axis',(1.,0.,4.93038065763132E-32));
#105905=DIRECTION('center_axis',(4.93038065763132E-32,1.97215226305253E-31,
-1.));
#105906=DIRECTION('ref_axis',(1.,0.,4.93038065763132E-32));
#105907=DIRECTION('',(4.93038065763132E-32,1.97215226305253E-31,-1.));
#105908=DIRECTION('center_axis',(4.93038065763132E-32,1.97215226305253E-31,
-1.));
#105909=DIRECTION('ref_axis',(1.,0.,4.93038065763132E-32));
#105910=DIRECTION('center_axis',(-4.93038065763132E-32,-1.97215226305253E-31,
1.));
#105911=DIRECTION('ref_axis',(1.,0.,4.93038065763132E-32));
#105912=DIRECTION('center_axis',(-4.93038065763132E-32,-1.97215226305253E-31,
1.));
#105913=DIRECTION('ref_axis',(1.,0.,4.93038065763132E-32));
#105914=DIRECTION('',(0.980976649545336,-0.194125766055945,1.00813261006593E-32));
#105915=DIRECTION('center_axis',(4.93038065763132E-32,1.97215226305253E-31,
-1.));
#105916=DIRECTION('ref_axis',(0.999629431953048,-0.0272212926442944,4.39170827718369E-32));
#105917=DIRECTION('',(-0.980976649545336,-0.194125766055945,-8.66504398694668E-32));
#105918=DIRECTION('center_axis',(-4.93038065763132E-32,-1.97215226305253E-31,
1.));
#105919=DIRECTION('ref_axis',(1.,0.,4.93038065763132E-32));
#105920=DIRECTION('',(0.907731042944837,0.419552563660715,1.27496749553964E-31));
#105921=DIRECTION('center_axis',(4.93038065763132E-32,1.97215226305253E-31,
-1.));
#105922=DIRECTION('ref_axis',(0.824717472892045,0.565544949501416,1.5219578596529E-31));
#105923=DIRECTION('',(-0.67952251818951,-0.733654651231345,-1.78190914873556E-31));
#105924=DIRECTION('center_axis',(-4.93038065763132E-32,-1.97215226305253E-31,
1.));
#105925=DIRECTION('ref_axis',(1.,0.,4.93038065763132E-32));
#105926=DIRECTION('',(0.487763030582801,0.872976074126136,1.96212748132788E-31));
#105927=DIRECTION('center_axis',(4.93038065763132E-32,1.97215226305253E-31,
-1.));
#105928=DIRECTION('ref_axis',(0.334791470302201,0.942292243103428,2.02340871864506E-31));
#105929=DIRECTION('',(-0.11851388100621,-0.992952395640821,-2.01668516882386E-31));
#105930=DIRECTION('center_axis',(-4.93038065763132E-32,-1.97215226305253E-31,
1.));
#105931=DIRECTION('ref_axis',(1.,0.,4.93038065763132E-32));
#105932=DIRECTION('',(-0.118513881006211,0.992952395640821,1.89982145950909E-31));
#105933=DIRECTION('center_axis',(4.93038065763132E-32,1.97215226305253E-31,
-1.));
#105934=DIRECTION('ref_axis',(-0.283013494799533,0.95911592717531,1.75198622024769E-31));
#105935=DIRECTION('',(0.487763030582801,-0.872976074126136,-1.48115599902926E-31));
#105936=DIRECTION('center_axis',(-4.93038065763132E-32,-1.97215226305253E-31,
1.));
#105937=DIRECTION('ref_axis',(1.,0.,4.93038065763132E-32));
#105938=DIRECTION('',(-0.67952251818951,0.733654651231345,1.11184821271426E-31));
#105939=DIRECTION('center_axis',(4.93038065763132E-32,1.97215226305253E-31,
-1.));
#105940=DIRECTION('ref_axis',(-0.792716924162737,0.609589926217592,8.11364533537153E-32));
#105941=DIRECTION('',(0.907731042944837,-0.419552563660715,-3.79875580246296E-32));
#105942=DIRECTION('center_axis',(-4.93038065763132E-32,-1.97215226305253E-31,
1.));
#105943=DIRECTION('ref_axis',(1.,0.,4.93038065763132E-32));
#105944=DIRECTION('',(-0.980976649545336,0.194125766055945,-1.00813261006593E-32));
#105945=DIRECTION('center_axis',(4.93038065763132E-32,1.97215226305253E-31,
-1.));
#105946=DIRECTION('ref_axis',(-0.999629431953048,0.0272212926442945,-4.39170827718369E-32));
#105947=DIRECTION('',(0.980976649545336,0.194125766055945,8.66504398694668E-32));
#105948=DIRECTION('center_axis',(-4.93038065763132E-32,-1.97215226305253E-31,
1.));
#105949=DIRECTION('ref_axis',(1.,0.,4.93038065763132E-32));
#105950=DIRECTION('',(-0.907731042944837,-0.419552563660715,-1.27496749553964E-31));
#105951=DIRECTION('center_axis',(4.93038065763132E-32,1.97215226305253E-31,
-1.));
#105952=DIRECTION('ref_axis',(-0.824717472892045,-0.565544949501416,-1.5219578596529E-31));
#105953=DIRECTION('',(0.67952251818951,0.733654651231345,1.78190914873556E-31));
#105954=DIRECTION('center_axis',(-4.93038065763132E-32,-1.97215226305253E-31,
1.));
#105955=DIRECTION('ref_axis',(1.,0.,4.93038065763132E-32));
#105956=DIRECTION('',(-0.487763030582801,-0.872976074126136,-1.96212748132788E-31));
#105957=DIRECTION('center_axis',(4.93038065763132E-32,1.97215226305253E-31,
-1.));
#105958=DIRECTION('ref_axis',(-0.334791470302201,-0.942292243103428,-2.02340871864506E-31));
#105959=DIRECTION('',(0.11851388100621,0.992952395640821,2.01668516882386E-31));
#105960=DIRECTION('center_axis',(-4.93038065763132E-32,-1.97215226305253E-31,
1.));
#105961=DIRECTION('ref_axis',(1.,0.,4.93038065763132E-32));
#105962=DIRECTION('',(0.118513881006211,-0.992952395640821,-1.89982145950909E-31));
#105963=DIRECTION('center_axis',(4.93038065763132E-32,1.97215226305253E-31,
-1.));
#105964=DIRECTION('ref_axis',(0.283013494799533,-0.95911592717531,-1.75198622024769E-31));
#105965=DIRECTION('',(-0.487763030582801,0.872976074126136,1.48115599902926E-31));
#105966=DIRECTION('center_axis',(-4.93038065763132E-32,-1.97215226305253E-31,
1.));
#105967=DIRECTION('ref_axis',(1.,0.,4.93038065763132E-32));
#105968=DIRECTION('',(0.67952251818951,-0.733654651231345,-1.11184821271426E-31));
#105969=DIRECTION('center_axis',(4.93038065763132E-32,1.97215226305253E-31,
-1.));
#105970=DIRECTION('ref_axis',(0.792716924162737,-0.609589926217592,-8.11364533537153E-32));
#105971=DIRECTION('',(-0.907731042944837,0.419552563660715,3.79875580246296E-32));
#105972=DIRECTION('center_axis',(-4.93038065763132E-32,-1.97215226305253E-31,
1.));
#105973=DIRECTION('ref_axis',(1.,0.,4.93038065763132E-32));
#105974=DIRECTION('center_axis',(-4.93038065763132E-32,-1.97215226305253E-31,
1.));
#105975=DIRECTION('ref_axis',(1.,0.,4.93038065763132E-32));
#105976=DIRECTION('center_axis',(-4.93038065763132E-32,-1.97215226305253E-31,
1.));
#105977=DIRECTION('ref_axis',(1.,0.,4.93038065763132E-32));
#105978=DIRECTION('',(-0.487763030582801,0.872976074126136,1.48115599902926E-31));
#105979=DIRECTION('center_axis',(-4.93038065763132E-32,-1.97215226305253E-31,
1.));
#105980=DIRECTION('ref_axis',(0.283013494799533,-0.95911592717531,-1.75198622024769E-31));
#105981=DIRECTION('',(0.11851388100621,-0.992952395640821,-1.89982145950909E-31));
#105982=DIRECTION('center_axis',(-4.93038065763132E-32,-1.97215226305253E-31,
1.));
#105983=DIRECTION('ref_axis',(1.,0.,4.93038065763132E-32));
#105984=DIRECTION('',(0.11851388100621,0.992952395640821,2.01668516882386E-31));
#105985=DIRECTION('center_axis',(-4.93038065763132E-32,-1.97215226305253E-31,
1.));
#105986=DIRECTION('ref_axis',(-0.334791470302201,-0.942292243103428,-2.02340871864506E-31));
#105987=DIRECTION('',(-0.487763030582801,-0.872976074126136,-1.96212748132788E-31));
#105988=DIRECTION('center_axis',(-4.93038065763132E-32,-1.97215226305253E-31,
1.));
#105989=DIRECTION('ref_axis',(1.,0.,4.93038065763132E-32));
#105990=DIRECTION('',(0.67952251818951,0.733654651231345,1.78190914873556E-31));
#105991=DIRECTION('center_axis',(-4.93038065763132E-32,-1.97215226305253E-31,
1.));
#105992=DIRECTION('ref_axis',(-0.824717472892045,-0.565544949501416,-1.5219578596529E-31));
#105993=DIRECTION('',(-0.907731042944837,-0.419552563660715,-1.27496749553964E-31));
#105994=DIRECTION('center_axis',(-4.93038065763132E-32,-1.97215226305253E-31,
1.));
#105995=DIRECTION('ref_axis',(1.,0.,4.93038065763132E-32));
#105996=DIRECTION('',(0.980976649545336,0.194125766055945,8.66504398694668E-32));
#105997=DIRECTION('center_axis',(-4.93038065763132E-32,-1.97215226305253E-31,
1.));
#105998=DIRECTION('ref_axis',(-0.999629431953048,0.0272212926442946,-4.39170827718369E-32));
#105999=DIRECTION('',(-0.980976649545336,0.194125766055945,-1.00813261006593E-32));
#106000=DIRECTION('center_axis',(-4.93038065763132E-32,-1.97215226305253E-31,
1.));
#106001=DIRECTION('ref_axis',(1.,0.,4.93038065763132E-32));
#106002=DIRECTION('',(0.907731042944837,-0.419552563660715,-3.79875580246296E-32));
#106003=DIRECTION('center_axis',(-4.93038065763132E-32,-1.97215226305253E-31,
1.));
#106004=DIRECTION('ref_axis',(-0.792716924162737,0.609589926217592,8.11364533537153E-32));
#106005=DIRECTION('',(-0.67952251818951,0.733654651231345,1.11184821271426E-31));
#106006=DIRECTION('center_axis',(-4.93038065763132E-32,-1.97215226305253E-31,
1.));
#106007=DIRECTION('ref_axis',(1.,0.,4.93038065763132E-32));
#106008=DIRECTION('',(0.487763030582801,-0.872976074126136,-1.48115599902926E-31));
#106009=DIRECTION('center_axis',(-4.93038065763132E-32,-1.97215226305253E-31,
1.));
#106010=DIRECTION('ref_axis',(-0.283013494799533,0.95911592717531,1.75198622024769E-31));
#106011=DIRECTION('',(-0.118513881006211,0.992952395640821,1.89982145950909E-31));
#106012=DIRECTION('center_axis',(-4.93038065763132E-32,-1.97215226305253E-31,
1.));
#106013=DIRECTION('ref_axis',(1.,0.,4.93038065763132E-32));
#106014=DIRECTION('',(-0.11851388100621,-0.992952395640821,-2.01668516882386E-31));
#106015=DIRECTION('center_axis',(-4.93038065763132E-32,-1.97215226305253E-31,
1.));
#106016=DIRECTION('ref_axis',(0.334791470302201,0.942292243103428,2.02340871864506E-31));
#106017=DIRECTION('',(0.487763030582801,0.872976074126136,1.96212748132788E-31));
#106018=DIRECTION('center_axis',(-4.93038065763132E-32,-1.97215226305253E-31,
1.));
#106019=DIRECTION('ref_axis',(1.,0.,4.93038065763132E-32));
#106020=DIRECTION('',(-0.67952251818951,-0.733654651231345,-1.78190914873556E-31));
#106021=DIRECTION('center_axis',(-4.93038065763132E-32,-1.97215226305253E-31,
1.));
#106022=DIRECTION('ref_axis',(0.824717472892045,0.565544949501416,1.5219578596529E-31));
#106023=DIRECTION('',(0.907731042944837,0.419552563660715,1.27496749553964E-31));
#106024=DIRECTION('center_axis',(-4.93038065763132E-32,-1.97215226305253E-31,
1.));
#106025=DIRECTION('ref_axis',(1.,0.,4.93038065763132E-32));
#106026=DIRECTION('',(-0.980976649545336,-0.194125766055945,-8.66504398694668E-32));
#106027=DIRECTION('center_axis',(-4.93038065763132E-32,-1.97215226305253E-31,
1.));
#106028=DIRECTION('ref_axis',(0.999629431953048,-0.0272212926442945,4.39170827718369E-32));
#106029=DIRECTION('',(0.980976649545336,-0.194125766055945,1.00813261006593E-32));
#106030=DIRECTION('center_axis',(-4.93038065763132E-32,-1.97215226305253E-31,
1.));
#106031=DIRECTION('ref_axis',(1.,0.,4.93038065763132E-32));
#106032=DIRECTION('',(-0.907731042944837,0.419552563660715,3.79875580246296E-32));
#106033=DIRECTION('center_axis',(-4.93038065763132E-32,-1.97215226305253E-31,
1.));
#106034=DIRECTION('ref_axis',(0.792716924162737,-0.609589926217592,-8.11364533537153E-32));
#106035=DIRECTION('',(0.67952251818951,-0.733654651231345,-1.11184821271426E-31));
#106036=DIRECTION('center_axis',(4.93038065763132E-32,1.97215226305253E-31,
-1.));
#106037=DIRECTION('ref_axis',(1.,0.,4.93038065763132E-32));
#106038=DIRECTION('center_axis',(-0.733654651231345,-0.67952251818951,2.41113348070025E-17));
#106039=DIRECTION('ref_axis',(-1.44471196324713E-17,-1.98847542650175E-17,
-1.));
#106040=DIRECTION('',(-4.93038065763132E-32,-1.97215226305253E-31,1.));
#106041=DIRECTION('',(-4.93038065763132E-32,-1.97215226305253E-31,1.));
#106042=DIRECTION('',(-4.33349072293499E-17,-5.96453828357725E-17,-1.));
#106043=DIRECTION('center_axis',(-4.93038065763132E-32,-1.97215226305253E-31,
1.));
#106044=DIRECTION('ref_axis',(0.792716924162737,-0.609589926217592,-8.11364533537153E-32));
#106045=DIRECTION('',(-2.56739074444567E-15,-1.97215226305253E-31,1.));
#106046=DIRECTION('',(-4.93038065763132E-32,-1.97215226305253E-31,1.));
#106047=DIRECTION('center_axis',(0.419552563660715,0.907731042944837,-5.10516967005408E-17));
#106048=DIRECTION('ref_axis',(3.05893462795411E-17,4.21026231781923E-17,
1.));
#106049=DIRECTION('',(4.93038065763132E-32,1.97215226305253E-31,-1.));
#106050=DIRECTION('center_axis',(-4.93038065763132E-32,-1.97215226305253E-31,
1.));
#106051=DIRECTION('ref_axis',(1.,0.,4.93038065763132E-32));
#106052=DIRECTION('',(4.93038065763132E-32,1.97215226305253E-31,-1.));
#106053=DIRECTION('center_axis',(-4.93038065763132E-32,-1.97215226305253E-31,
1.));
#106054=DIRECTION('ref_axis',(1.,0.,4.93038065763132E-32));
#106055=DIRECTION('',(-4.93038065763132E-32,-1.97215226305253E-31,1.));
#106056=DIRECTION('center_axis',(-0.992952395640821,-0.118513881006211,
2.41113348070026E-17));
#106057=DIRECTION('ref_axis',(-2.33759306048745E-17,-7.59530027129711E-18,
-1.));
#106058=DIRECTION('',(-4.93038065763132E-32,-1.97215226305253E-31,1.));
#106059=DIRECTION('',(-4.93038065763132E-32,-1.97215226305253E-31,1.));
#106060=DIRECTION('',(-7.01173527964117E-17,-2.27825089712654E-17,-1.));
#106061=DIRECTION('center_axis',(-4.93038065763132E-32,-1.97215226305253E-31,
1.));
#106062=DIRECTION('ref_axis',(0.283013494799533,-0.95911592717531,-1.75198622024769E-31));
#106063=DIRECTION('',(-4.93038065763132E-32,-1.97215226305253E-31,1.));
#106064=DIRECTION('',(-4.93038065763132E-32,-1.97215226305253E-31,1.));
#106065=DIRECTION('center_axis',(0.872976074126136,0.487763030582801,-5.10516967005409E-17));
#106066=DIRECTION('ref_axis',(4.94946019739376E-17,1.60817710385402E-17,
1.));
#106067=DIRECTION('center_axis',(-4.93038065763132E-32,-1.97215226305253E-31,
1.));
#106068=DIRECTION('ref_axis',(1.,0.,4.93038065763132E-32));
#106069=DIRECTION('',(4.93038065763132E-32,1.97215226305253E-31,-1.));
#106070=DIRECTION('center_axis',(-0.872976074126136,0.487763030582801,2.41113348070028E-17));
#106071=DIRECTION('ref_axis',(-2.33759306048745E-17,7.59530027129753E-18,
-1.));
#106072=DIRECTION('',(-4.93038065763132E-32,-1.97215226305253E-31,1.));
#106073=DIRECTION('',(-4.93038065763132E-32,-1.97215226305253E-31,1.));
#106074=DIRECTION('',(-7.01173527964117E-17,2.27825089712658E-17,-1.));
#106075=DIRECTION('center_axis',(-4.93038065763132E-32,-1.97215226305253E-31,
1.));
#106076=DIRECTION('ref_axis',(-0.334791470302201,-0.942292243103428,-2.02340871864506E-31));
#106077=DIRECTION('',(2.42861286636753E-16,-1.97215226305253E-31,1.));
#106078=DIRECTION('',(-4.93038065763132E-32,-1.97215226305253E-31,1.));
#106079=DIRECTION('center_axis',(0.992952395640821,-0.118513881006211,-5.1051696700541E-17));
#106080=DIRECTION('ref_axis',(4.94946019739376E-17,-1.60817710385406E-17,
1.));
#106081=DIRECTION('center_axis',(-4.93038065763132E-32,-1.97215226305253E-31,
1.));
#106082=DIRECTION('ref_axis',(1.,0.,4.93038065763132E-32));
#106083=DIRECTION('',(4.93038065763132E-32,1.97215226305253E-31,-1.));
#106084=DIRECTION('center_axis',(-0.419552563660715,0.907731042944837,2.41113348070029E-17));
#106085=DIRECTION('ref_axis',(-1.44471196324713E-17,1.98847542650179E-17,
-1.));
#106086=DIRECTION('',(-4.93038065763132E-32,-1.97215226305253E-31,1.));
#106087=DIRECTION('',(-4.93038065763132E-32,-1.97215226305253E-31,1.));
#106088=DIRECTION('',(-4.33349072293499E-17,5.9645382835773E-17,-1.));
#106089=DIRECTION('center_axis',(-4.93038065763132E-32,-1.97215226305253E-31,
1.));
#106090=DIRECTION('ref_axis',(-0.824717472892045,-0.565544949501416,-1.5219578596529E-31));
#106091=DIRECTION('',(-4.93038065763132E-32,-1.97215226305253E-31,1.));
#106092=DIRECTION('',(-4.93038065763132E-32,-1.97215226305253E-31,1.));
#106093=DIRECTION('center_axis',(0.733654651231345,-0.67952251818951,-5.10516967005411E-17));
#106094=DIRECTION('ref_axis',(3.05893462795411E-17,-4.21026231781927E-17,
1.));
#106095=DIRECTION('center_axis',(-4.93038065763132E-32,-1.97215226305253E-31,
1.));
#106096=DIRECTION('ref_axis',(1.,0.,4.93038065763132E-32));
#106097=DIRECTION('',(4.93038065763132E-32,1.97215226305253E-31,-1.));
#106098=DIRECTION('center_axis',(0.194125766055945,0.980976649545336,2.41113348070029E-17));
#106099=DIRECTION('ref_axis',(6.16297582203915E-32,2.45789079874409E-17,
-1.));
#106100=DIRECTION('',(-4.93038065763132E-32,-1.97215226305253E-31,1.));
#106101=DIRECTION('',(-4.93038065763132E-32,-1.97215226305253E-31,1.));
#106102=DIRECTION('',(5.83326066734215E-32,7.37257477290145E-17,-1.));
#106103=DIRECTION('center_axis',(-4.93038065763132E-32,-1.97215226305253E-31,
1.));
#106104=DIRECTION('ref_axis',(-0.999629431953048,0.0272212926442946,-4.39170827718369E-32));
#106105=DIRECTION('',(2.4980018054066E-15,-1.97215226305253E-31,1.));
#106106=DIRECTION('',(-4.93038065763132E-32,-1.97215226305253E-31,1.));
#106107=DIRECTION('center_axis',(0.194125766055945,-0.980976649545336,-5.10516967005412E-17));
#106108=DIRECTION('ref_axis',(-5.8548270309372E-32,-5.20417042793044E-17,
1.));
#106109=DIRECTION('center_axis',(-4.93038065763132E-32,-1.97215226305253E-31,
1.));
#106110=DIRECTION('ref_axis',(1.,0.,4.93038065763132E-32));
#106111=DIRECTION('',(4.93038065763132E-32,1.97215226305253E-31,-1.));
#106112=DIRECTION('center_axis',(0.733654651231345,0.67952251818951,2.41113348070029E-17));
#106113=DIRECTION('ref_axis',(1.44471196324714E-17,1.98847542650179E-17,
-1.));
#106114=DIRECTION('',(-4.93038065763132E-32,-1.97215226305253E-31,1.));
#106115=DIRECTION('',(-4.93038065763132E-32,-1.97215226305253E-31,1.));
#106116=DIRECTION('',(4.33349072293499E-17,5.9645382835773E-17,-1.));
#106117=DIRECTION('center_axis',(-4.93038065763132E-32,-1.97215226305253E-31,
1.));
#106118=DIRECTION('ref_axis',(-0.792716924162737,0.609589926217592,8.11364533537153E-32));
#106119=DIRECTION('',(2.56739074444567E-15,-1.97215226305253E-31,1.));
#106120=DIRECTION('',(-4.93038065763132E-32,-1.97215226305253E-31,1.));
#106121=DIRECTION('center_axis',(-0.419552563660715,-0.907731042944837,
-5.10516967005412E-17));
#106122=DIRECTION('ref_axis',(-3.05893462795412E-17,-4.21026231781927E-17,
1.));
#106123=DIRECTION('center_axis',(-4.93038065763132E-32,-1.97215226305253E-31,
1.));
#106124=DIRECTION('ref_axis',(1.,0.,4.93038065763132E-32));
#106125=DIRECTION('',(4.93038065763132E-32,1.97215226305253E-31,-1.));
#106126=DIRECTION('center_axis',(0.992952395640821,0.118513881006211,2.41113348070028E-17));
#106127=DIRECTION('ref_axis',(2.33759306048746E-17,7.59530027129751E-18,
-1.));
#106128=DIRECTION('',(-4.93038065763132E-32,-1.97215226305253E-31,1.));
#106129=DIRECTION('',(-4.93038065763132E-32,-1.97215226305253E-31,1.));
#106130=DIRECTION('',(7.01173527964118E-17,2.27825089712658E-17,-1.));
#106131=DIRECTION('center_axis',(-4.93038065763132E-32,-1.97215226305253E-31,
1.));
#106132=DIRECTION('ref_axis',(-0.283013494799533,0.95911592717531,1.75198622024769E-31));
#106133=DIRECTION('',(-4.93038065763132E-32,-1.97215226305253E-31,1.));
#106134=DIRECTION('',(-2.4980018054066E-15,-1.97215226305253E-31,1.));
#106135=DIRECTION('center_axis',(-0.872976074126136,-0.487763030582801,
-5.10516967005412E-17));
#106136=DIRECTION('ref_axis',(-4.94946019739377E-17,-1.60817710385406E-17,
1.));
#106137=DIRECTION('center_axis',(-4.93038065763132E-32,-1.97215226305253E-31,
1.));
#106138=DIRECTION('ref_axis',(1.,0.,4.93038065763132E-32));
#106139=DIRECTION('',(4.93038065763132E-32,1.97215226305253E-31,-1.));
#106140=DIRECTION('center_axis',(0.872976074126137,-0.487763030582801,2.41113348070026E-17));
#106141=DIRECTION('ref_axis',(2.33759306048745E-17,-7.59530027129711E-18,
-1.));
#106142=DIRECTION('',(-4.93038065763132E-32,-1.97215226305253E-31,1.));
#106143=DIRECTION('',(-4.93038065763132E-32,2.44249065417534E-14,1.));
#106144=DIRECTION('',(7.01173527964118E-17,-2.27825089712654E-17,-1.));
#106145=DIRECTION('center_axis',(-4.93038065763132E-32,-1.97215226305253E-31,
1.));
#106146=DIRECTION('ref_axis',(0.334791470302201,0.942292243103428,2.02340871864506E-31));
#106147=DIRECTION('',(-4.93038065763132E-32,-1.97215226305253E-31,1.));
#106148=DIRECTION('',(-4.93038065763132E-32,-1.97215226305253E-31,1.));
#106149=DIRECTION('center_axis',(-0.992952395640821,0.118513881006211,-5.1051696700541E-17));
#106150=DIRECTION('ref_axis',(-4.94946019739377E-17,1.60817710385402E-17,
1.));
#106151=DIRECTION('center_axis',(-4.93038065763132E-32,-1.97215226305253E-31,
1.));
#106152=DIRECTION('ref_axis',(1.,0.,4.93038065763132E-32));
#106153=DIRECTION('',(4.93038065763132E-32,1.97215226305253E-31,-1.));
#106154=DIRECTION('center_axis',(0.419552563660715,-0.907731042944837,2.41113348070025E-17));
#106155=DIRECTION('ref_axis',(1.44471196324714E-17,-1.98847542650175E-17,
-1.));
#106156=DIRECTION('',(-4.93038065763132E-32,-1.97215226305253E-31,1.));
#106157=DIRECTION('',(-4.93038065763132E-32,-1.97215226305253E-31,1.));
#106158=DIRECTION('',(4.33349072293499E-17,-5.96453828357726E-17,-1.));
#106159=DIRECTION('center_axis',(-4.93038065763132E-32,-1.97215226305253E-31,
1.));
#106160=DIRECTION('ref_axis',(0.824717472892045,0.565544949501416,1.5219578596529E-31));
#106161=DIRECTION('',(-4.93038065763132E-32,-1.97215226305253E-31,1.));
#106162=DIRECTION('',(-4.93038065763132E-32,-1.97215226305253E-31,1.));
#106163=DIRECTION('center_axis',(-0.733654651231345,0.67952251818951,-5.10516967005409E-17));
#106164=DIRECTION('ref_axis',(-3.05893462795412E-17,4.21026231781923E-17,
1.));
#106165=DIRECTION('center_axis',(-4.93038065763132E-32,-1.97215226305253E-31,
1.));
#106166=DIRECTION('ref_axis',(1.,0.,4.93038065763132E-32));
#106167=DIRECTION('',(4.93038065763132E-32,1.97215226305253E-31,-1.));
#106168=DIRECTION('center_axis',(-0.194125766055945,-0.980976649545336,
2.41113348070025E-17));
#106169=DIRECTION('ref_axis',(4.00593428432545E-32,-2.45789079874405E-17,
-1.));
#106170=DIRECTION('',(-4.93038065763132E-32,-1.97215226305253E-31,1.));
#106171=DIRECTION('',(4.93038065763132E-32,-7.37257477290141E-17,-1.));
#106172=DIRECTION('center_axis',(-4.93038065763132E-32,-1.97215226305253E-31,
1.));
#106173=DIRECTION('ref_axis',(0.999629431953048,-0.0272212926442945,4.39170827718369E-32));
#106174=DIRECTION('',(-2.4980018054066E-15,-1.97215226305253E-31,1.));
#106175=DIRECTION('',(-4.93038065763132E-32,-1.97215226305253E-31,1.));
#106176=DIRECTION('center_axis',(-0.194125766055945,0.980976649545336,-5.10516967005408E-17));
#106177=DIRECTION('ref_axis',(-4.62223186652937E-32,5.2041704279304E-17,
1.));
#106178=DIRECTION('center_axis',(-4.93038065763132E-32,-1.97215226305253E-31,
1.));
#106179=DIRECTION('ref_axis',(-0.464722744083384,0.885456250264015,1.51712854493318E-31));
#106180=DIRECTION('center_axis',(4.93038065763132E-32,1.97215226305253E-31,
-1.));
#106181=DIRECTION('ref_axis',(1.,0.,4.93038065763132E-32));
#106182=DIRECTION('',(-0.415660658584274,0.791976146676961,-0.447213595499958));
#106183=DIRECTION('center_axis',(4.93038065763132E-32,1.97215226305253E-31,
-1.));
#106184=DIRECTION('ref_axis',(1.,7.65671051465626E-16,4.93038065763134E-32));
#106185=DIRECTION('center_axis',(4.93038065763132E-32,1.97215226305253E-31,
-1.));
#106186=DIRECTION('ref_axis',(1.,0.,4.93038065763132E-32));
#106187=DIRECTION('center_axis',(4.93038065763132E-32,1.97215226305253E-31,
-1.));
#106188=DIRECTION('ref_axis',(-0.464722744083384,0.885456250264015,1.51712854493318E-31));
#106189=DIRECTION('center_axis',(-4.93038065763132E-32,-1.97215226305253E-31,
1.));
#106190=DIRECTION('ref_axis',(1.,0.,4.93038065763132E-32));
#106191=DIRECTION('',(-0.415660658584278,0.791976146676969,0.447213595499941));
#106192=DIRECTION('center_axis',(-4.93038065763132E-32,-1.97215226305253E-31,
1.));
#106193=DIRECTION('ref_axis',(1.,0.,4.93038065763132E-32));
#106194=DIRECTION('center_axis',(4.93038065763132E-32,1.97215226305253E-31,
-1.));
#106195=DIRECTION('ref_axis',(1.,0.,4.93038065763132E-32));
#106196=DIRECTION('',(-4.93038065763132E-32,-1.97215226305253E-31,1.));
#106197=DIRECTION('center_axis',(-4.93038065763132E-32,-1.97215226305253E-31,
1.));
#106198=DIRECTION('ref_axis',(1.,0.,4.93038065763132E-32));
#106199=DIRECTION('center_axis',(-4.93038065763132E-32,-1.97215226305253E-31,
1.));
#106200=DIRECTION('ref_axis',(1.,0.,4.93038065763132E-32));
#106201=DIRECTION('center_axis',(4.93038065763132E-32,1.97215226305253E-31,
-1.));
#106202=DIRECTION('ref_axis',(1.,0.,4.93038065763132E-32));
#106203=DIRECTION('',(-4.93038065763132E-32,-1.97215226305253E-31,1.));
#106204=DIRECTION('center_axis',(-4.93038065763132E-32,-1.97215226305253E-31,
1.));
#106205=DIRECTION('ref_axis',(-0.464722744083384,0.885456250264015,1.51712854493318E-31));
#106206=DIRECTION('center_axis',(4.93038065763132E-32,1.97215226305253E-31,
-1.));
#106207=DIRECTION('ref_axis',(1.,0.,4.93038065763132E-32));
#106208=DIRECTION('',(-0.415660658584274,0.791976146676961,-0.447213595499958));
#106209=DIRECTION('center_axis',(4.93038065763132E-32,1.97215226305253E-31,
-1.));
#106210=DIRECTION('ref_axis',(1.,7.65671051465626E-16,4.93038065763134E-32));
#106211=DIRECTION('center_axis',(4.93038065763132E-32,1.97215226305253E-31,
-1.));
#106212=DIRECTION('ref_axis',(1.,0.,4.93038065763132E-32));
#106213=DIRECTION('center_axis',(4.93038065763132E-32,1.97215226305253E-31,
-1.));
#106214=DIRECTION('ref_axis',(-0.464722744083384,0.885456250264015,1.51712854493318E-31));
#106215=DIRECTION('',(-0.415660658584278,0.791976146676969,0.447213595499941));
#106216=DIRECTION('center_axis',(4.93038065763132E-32,1.97215226305253E-31,
-1.));
#106217=DIRECTION('ref_axis',(1.,0.,4.93038065763132E-32));
#106218=DIRECTION('',(-4.93038065763132E-32,-1.97215226305253E-31,1.));
#106219=DIRECTION('center_axis',(-4.93038065763132E-32,-1.97215226305253E-31,
1.));
#106220=DIRECTION('ref_axis',(1.,0.,4.93038065763132E-32));
#106221=DIRECTION('center_axis',(-4.93038065763132E-32,-1.97215226305253E-31,
1.));
#106222=DIRECTION('ref_axis',(1.,0.,4.93038065763132E-32));
#106223=DIRECTION('center_axis',(-4.93038065763132E-32,-1.97215226305253E-31,
1.));
#106224=DIRECTION('ref_axis',(-0.464722744083384,0.885456250264015,1.51712854493318E-31));
#106225=DIRECTION('center_axis',(4.93038065763132E-32,1.97215226305253E-31,
-1.));
#106226=DIRECTION('ref_axis',(1.,0.,4.93038065763132E-32));
#106227=DIRECTION('',(-0.415660658584274,0.791976146676961,-0.447213595499958));
#106228=DIRECTION('center_axis',(4.93038065763132E-32,1.97215226305253E-31,
-1.));
#106229=DIRECTION('ref_axis',(1.,7.65671051465626E-16,4.93038065763134E-32));
#106230=DIRECTION('center_axis',(4.93038065763132E-32,1.97215226305253E-31,
-1.));
#106231=DIRECTION('ref_axis',(1.,0.,4.93038065763132E-32));
#106232=DIRECTION('center_axis',(4.93038065763132E-32,1.97215226305253E-31,
-1.));
#106233=DIRECTION('ref_axis',(-0.464722744083384,0.885456250264015,1.51712854493318E-31));
#106234=DIRECTION('',(-0.415660658584278,0.791976146676969,0.447213595499941));
#106235=DIRECTION('center_axis',(4.93038065763132E-32,1.97215226305253E-31,
-1.));
#106236=DIRECTION('ref_axis',(1.,0.,4.93038065763132E-32));
#106237=DIRECTION('',(-4.93038065763132E-32,-1.97215226305253E-31,1.));
#106238=DIRECTION('center_axis',(-4.93038065763132E-32,-1.97215226305253E-31,
1.));
#106239=DIRECTION('ref_axis',(1.,0.,4.93038065763132E-32));
#106240=DIRECTION('center_axis',(-4.93038065763132E-32,-1.97215226305253E-31,
1.));
#106241=DIRECTION('ref_axis',(1.,0.,4.93038065763132E-32));
#106242=DIRECTION('center_axis',(-4.93038065763132E-32,-1.97215226305253E-31,
1.));
#106243=DIRECTION('ref_axis',(-0.464722744083384,0.885456250264015,1.51712854493318E-31));
#106244=DIRECTION('center_axis',(4.93038065763132E-32,1.97215226305253E-31,
-1.));
#106245=DIRECTION('ref_axis',(1.,0.,4.93038065763132E-32));
#106246=DIRECTION('',(-0.415660658584274,0.791976146676961,-0.447213595499958));
#106247=DIRECTION('center_axis',(4.93038065763132E-32,1.97215226305253E-31,
-1.));
#106248=DIRECTION('ref_axis',(1.,7.65671051465626E-16,4.93038065763134E-32));
#106249=DIRECTION('center_axis',(4.93038065763132E-32,1.97215226305253E-31,
-1.));
#106250=DIRECTION('ref_axis',(1.,0.,4.93038065763132E-32));
#106251=DIRECTION('center_axis',(4.93038065763132E-32,1.97215226305253E-31,
-1.));
#106252=DIRECTION('ref_axis',(-0.464722744083384,0.885456250264015,1.51712854493318E-31));
#106253=DIRECTION('',(-0.415660658584278,0.791976146676969,0.447213595499941));
#106254=DIRECTION('center_axis',(4.93038065763132E-32,1.97215226305253E-31,
-1.));
#106255=DIRECTION('ref_axis',(1.,0.,4.93038065763132E-32));
#106256=DIRECTION('',(-4.93038065763132E-32,-1.97215226305253E-31,1.));
#106257=DIRECTION('center_axis',(-4.93038065763132E-32,-1.97215226305253E-31,
1.));
#106258=DIRECTION('ref_axis',(1.,0.,4.93038065763132E-32));
#106259=DIRECTION('center_axis',(-4.93038065763132E-32,-1.97215226305253E-31,
1.));
#106260=DIRECTION('ref_axis',(1.,0.,4.93038065763132E-32));
#106261=DIRECTION('center_axis',(-4.93038065763132E-32,-1.97215226305253E-31,
1.));
#106262=DIRECTION('ref_axis',(-0.464722744083384,0.885456250264015,1.51712854493318E-31));
#106263=DIRECTION('center_axis',(4.93038065763132E-32,1.97215226305253E-31,
-1.));
#106264=DIRECTION('ref_axis',(1.,0.,4.93038065763132E-32));
#106265=DIRECTION('',(-0.415660658584274,0.791976146676961,-0.447213595499958));
#106266=DIRECTION('center_axis',(4.93038065763132E-32,1.97215226305253E-31,
-1.));
#106267=DIRECTION('ref_axis',(1.,7.65671051465626E-16,4.93038065763134E-32));
#106268=DIRECTION('center_axis',(4.93038065763132E-32,1.97215226305253E-31,
-1.));
#106269=DIRECTION('ref_axis',(1.,0.,4.93038065763132E-32));
#106270=DIRECTION('center_axis',(4.93038065763132E-32,1.97215226305253E-31,
-1.));
#106271=DIRECTION('ref_axis',(-0.464722744083384,0.885456250264015,1.51712854493318E-31));
#106272=DIRECTION('',(-0.415660658584278,0.791976146676969,0.447213595499941));
#106273=DIRECTION('center_axis',(4.93038065763132E-32,1.97215226305253E-31,
-1.));
#106274=DIRECTION('ref_axis',(1.,0.,4.93038065763132E-32));
#106275=DIRECTION('',(-4.93038065763132E-32,-1.97215226305253E-31,1.));
#106276=DIRECTION('center_axis',(-4.93038065763132E-32,-1.97215226305253E-31,
1.));
#106277=DIRECTION('ref_axis',(1.,0.,4.93038065763132E-32));
#106278=DIRECTION('center_axis',(-4.93038065763132E-32,-1.97215226305253E-31,
1.));
#106279=DIRECTION('ref_axis',(1.,0.,4.93038065763132E-32));
#106280=DIRECTION('center_axis',(-4.93038065763132E-32,-1.97215226305253E-31,
1.));
#106281=DIRECTION('ref_axis',(-0.464722744083384,0.885456250264015,1.51712854493318E-31));
#106282=DIRECTION('center_axis',(4.93038065763132E-32,1.97215226305253E-31,
-1.));
#106283=DIRECTION('ref_axis',(1.,0.,4.93038065763132E-32));
#106284=DIRECTION('',(-0.415660658584274,0.791976146676961,-0.447213595499958));
#106285=DIRECTION('center_axis',(4.93038065763132E-32,1.97215226305253E-31,
-1.));
#106286=DIRECTION('ref_axis',(1.,7.65671051465626E-16,4.93038065763134E-32));
#106287=DIRECTION('center_axis',(4.93038065763132E-32,1.97215226305253E-31,
-1.));
#106288=DIRECTION('ref_axis',(1.,0.,4.93038065763132E-32));
#106289=DIRECTION('center_axis',(4.93038065763132E-32,1.97215226305253E-31,
-1.));
#106290=DIRECTION('ref_axis',(-0.464722744083384,0.885456250264015,1.51712854493318E-31));
#106291=DIRECTION('',(-0.415660658584278,0.791976146676969,0.447213595499941));
#106292=DIRECTION('center_axis',(4.93038065763132E-32,1.97215226305253E-31,
-1.));
#106293=DIRECTION('ref_axis',(1.,0.,4.93038065763132E-32));
#106294=DIRECTION('',(-4.93038065763132E-32,-1.97215226305253E-31,1.));
#106295=DIRECTION('center_axis',(-4.93038065763132E-32,-1.97215226305253E-31,
1.));
#106296=DIRECTION('ref_axis',(1.,0.,4.93038065763132E-32));
#106297=DIRECTION('center_axis',(-4.93038065763132E-32,-1.97215226305253E-31,
1.));
#106298=DIRECTION('ref_axis',(1.,0.,4.93038065763132E-32));
#106299=DIRECTION('center_axis',(-4.93038065763132E-32,-1.97215226305253E-31,
1.));
#106300=DIRECTION('ref_axis',(-0.464722744083384,0.885456250264015,1.51712854493318E-31));
#106301=DIRECTION('center_axis',(4.93038065763132E-32,1.97215226305253E-31,
-1.));
#106302=DIRECTION('ref_axis',(1.,0.,4.93038065763132E-32));
#106303=DIRECTION('',(-0.415660658584274,0.791976146676961,-0.447213595499958));
#106304=DIRECTION('center_axis',(4.93038065763132E-32,1.97215226305253E-31,
-1.));
#106305=DIRECTION('ref_axis',(1.,7.65671051465626E-16,4.93038065763134E-32));
#106306=DIRECTION('center_axis',(4.93038065763132E-32,1.97215226305253E-31,
-1.));
#106307=DIRECTION('ref_axis',(1.,0.,4.93038065763132E-32));
#106308=DIRECTION('center_axis',(4.93038065763132E-32,1.97215226305253E-31,
-1.));
#106309=DIRECTION('ref_axis',(-0.464722744083384,0.885456250264015,1.51712854493318E-31));
#106310=DIRECTION('',(-0.415660658584278,0.791976146676969,0.447213595499941));
#106311=DIRECTION('center_axis',(4.93038065763132E-32,1.97215226305253E-31,
-1.));
#106312=DIRECTION('ref_axis',(1.,0.,4.93038065763132E-32));
#106313=DIRECTION('',(-4.93038065763132E-32,-1.97215226305253E-31,1.));
#106314=DIRECTION('center_axis',(-4.93038065763132E-32,-1.97215226305253E-31,
1.));
#106315=DIRECTION('ref_axis',(1.,0.,4.93038065763132E-32));
#106316=DIRECTION('center_axis',(-4.93038065763132E-32,-1.97215226305253E-31,
1.));
#106317=DIRECTION('ref_axis',(1.,0.,4.93038065763132E-32));
#106318=DIRECTION('center_axis',(-4.93038065763132E-32,-1.97215226305253E-31,
1.));
#106319=DIRECTION('ref_axis',(-0.464722744083384,0.885456250264015,1.51712854493318E-31));
#106320=DIRECTION('center_axis',(4.93038065763132E-32,1.97215226305253E-31,
-1.));
#106321=DIRECTION('ref_axis',(1.,0.,4.93038065763132E-32));
#106322=DIRECTION('',(-0.415660658584274,0.791976146676961,-0.447213595499958));
#106323=DIRECTION('center_axis',(4.93038065763132E-32,1.97215226305253E-31,
-1.));
#106324=DIRECTION('ref_axis',(1.,7.65671051465626E-16,4.93038065763134E-32));
#106325=DIRECTION('center_axis',(4.93038065763132E-32,1.97215226305253E-31,
-1.));
#106326=DIRECTION('ref_axis',(1.,0.,4.93038065763132E-32));
#106327=DIRECTION('center_axis',(4.93038065763132E-32,1.97215226305253E-31,
-1.));
#106328=DIRECTION('ref_axis',(-0.464722744083384,0.885456250264015,1.51712854493318E-31));
#106329=DIRECTION('',(-0.415660658584278,0.791976146676969,0.447213595499941));
#106330=DIRECTION('center_axis',(4.93038065763132E-32,1.97215226305253E-31,
-1.));
#106331=DIRECTION('ref_axis',(1.,0.,4.93038065763132E-32));
#106332=DIRECTION('',(-4.93038065763132E-32,-1.97215226305253E-31,1.));
#106333=DIRECTION('center_axis',(-4.93038065763132E-32,-1.97215226305253E-31,
1.));
#106334=DIRECTION('ref_axis',(1.,0.,4.93038065763132E-32));
#106335=DIRECTION('center_axis',(-4.93038065763132E-32,-1.97215226305253E-31,
1.));
#106336=DIRECTION('ref_axis',(1.,0.,4.93038065763132E-32));
#106337=DIRECTION('center_axis',(-4.93038065763132E-32,-1.97215226305253E-31,
1.));
#106338=DIRECTION('ref_axis',(-0.464722744083384,0.885456250264015,1.51712854493318E-31));
#106339=DIRECTION('center_axis',(4.93038065763132E-32,1.97215226305253E-31,
-1.));
#106340=DIRECTION('ref_axis',(1.,0.,4.93038065763132E-32));
#106341=DIRECTION('',(-0.415660658584274,0.791976146676961,-0.447213595499958));
#106342=DIRECTION('center_axis',(4.93038065763132E-32,1.97215226305253E-31,
-1.));
#106343=DIRECTION('ref_axis',(1.,7.65671051465626E-16,4.93038065763134E-32));
#106344=DIRECTION('center_axis',(4.93038065763132E-32,1.97215226305253E-31,
-1.));
#106345=DIRECTION('ref_axis',(1.,0.,4.93038065763132E-32));
#106346=DIRECTION('center_axis',(4.93038065763132E-32,1.97215226305253E-31,
-1.));
#106347=DIRECTION('ref_axis',(-0.464722744083384,0.885456250264015,1.51712854493318E-31));
#106348=DIRECTION('',(-0.415660658584278,0.791976146676969,0.447213595499941));
#106349=DIRECTION('center_axis',(4.93038065763132E-32,1.97215226305253E-31,
-1.));
#106350=DIRECTION('ref_axis',(1.,0.,4.93038065763132E-32));
#106351=DIRECTION('',(-4.93038065763132E-32,-1.97215226305253E-31,1.));
#106352=DIRECTION('center_axis',(-4.93038065763132E-32,-1.97215226305253E-31,
1.));
#106353=DIRECTION('ref_axis',(1.,0.,4.93038065763132E-32));
#106354=DIRECTION('center_axis',(-4.93038065763132E-32,-1.97215226305253E-31,
1.));
#106355=DIRECTION('ref_axis',(1.,0.,4.93038065763132E-32));
#106356=DIRECTION('center_axis',(-4.93038065763132E-32,-1.97215226305253E-31,
1.));
#106357=DIRECTION('ref_axis',(-0.464722744083384,0.885456250264015,1.51712854493318E-31));
#106358=DIRECTION('center_axis',(4.93038065763132E-32,1.97215226305253E-31,
-1.));
#106359=DIRECTION('ref_axis',(1.,0.,4.93038065763132E-32));
#106360=DIRECTION('',(-0.415660658584274,0.791976146676961,-0.447213595499958));
#106361=DIRECTION('center_axis',(4.93038065763132E-32,1.97215226305253E-31,
-1.));
#106362=DIRECTION('ref_axis',(1.,7.65671051465626E-16,4.93038065763134E-32));
#106363=DIRECTION('center_axis',(4.93038065763132E-32,1.97215226305253E-31,
-1.));
#106364=DIRECTION('ref_axis',(1.,0.,4.93038065763132E-32));
#106365=DIRECTION('center_axis',(4.93038065763132E-32,1.97215226305253E-31,
-1.));
#106366=DIRECTION('ref_axis',(-0.464722744083384,0.885456250264015,1.51712854493318E-31));
#106367=DIRECTION('',(-0.415660658584278,0.791976146676969,0.447213595499941));
#106368=DIRECTION('center_axis',(4.93038065763132E-32,1.97215226305253E-31,
-1.));
#106369=DIRECTION('ref_axis',(1.,0.,4.93038065763132E-32));
#106370=DIRECTION('',(-4.93038065763132E-32,-1.97215226305253E-31,1.));
#106371=DIRECTION('center_axis',(-4.93038065763132E-32,-1.97215226305253E-31,
1.));
#106372=DIRECTION('ref_axis',(1.,0.,4.93038065763132E-32));
#106373=DIRECTION('center_axis',(-4.93038065763132E-32,-1.97215226305253E-31,
1.));
#106374=DIRECTION('ref_axis',(1.,0.,4.93038065763132E-32));
#106375=DIRECTION('center_axis',(-4.93038065763132E-32,-1.97215226305253E-31,
1.));
#106376=DIRECTION('ref_axis',(-0.464722744083384,0.885456250264015,1.51712854493318E-31));
#106377=DIRECTION('center_axis',(4.93038065763132E-32,1.97215226305253E-31,
-1.));
#106378=DIRECTION('ref_axis',(1.,0.,4.93038065763132E-32));
#106379=DIRECTION('',(-0.415660658584274,0.791976146676961,-0.447213595499958));
#106380=DIRECTION('center_axis',(4.93038065763132E-32,1.97215226305253E-31,
-1.));
#106381=DIRECTION('ref_axis',(1.,7.65671051465626E-16,4.93038065763134E-32));
#106382=DIRECTION('center_axis',(4.93038065763132E-32,1.97215226305253E-31,
-1.));
#106383=DIRECTION('ref_axis',(1.,0.,4.93038065763132E-32));
#106384=DIRECTION('center_axis',(4.93038065763132E-32,1.97215226305253E-31,
-1.));
#106385=DIRECTION('ref_axis',(-0.464722744083384,0.885456250264015,1.51712854493318E-31));
#106386=DIRECTION('',(-0.415660658584278,0.791976146676969,0.447213595499941));
#106387=DIRECTION('center_axis',(4.93038065763132E-32,1.97215226305253E-31,
-1.));
#106388=DIRECTION('ref_axis',(1.,0.,4.93038065763132E-32));
#106389=DIRECTION('',(-4.93038065763132E-32,-1.97215226305253E-31,1.));
#106390=DIRECTION('center_axis',(-4.93038065763132E-32,-1.97215226305253E-31,
1.));
#106391=DIRECTION('ref_axis',(1.,0.,4.93038065763132E-32));
#106392=DIRECTION('center_axis',(-4.93038065763132E-32,-1.97215226305253E-31,
1.));
#106393=DIRECTION('ref_axis',(1.,0.,4.93038065763132E-32));
#106394=DIRECTION('center_axis',(-4.93038065763132E-32,-1.97215226305253E-31,
1.));
#106395=DIRECTION('ref_axis',(-0.464722744083384,0.885456250264015,1.51712854493318E-31));
#106396=DIRECTION('center_axis',(4.93038065763132E-32,1.97215226305253E-31,
-1.));
#106397=DIRECTION('ref_axis',(1.,0.,4.93038065763132E-32));
#106398=DIRECTION('',(-0.415660658584274,0.791976146676961,-0.447213595499958));
#106399=DIRECTION('center_axis',(4.93038065763132E-32,1.97215226305253E-31,
-1.));
#106400=DIRECTION('ref_axis',(1.,7.65671051465626E-16,4.93038065763134E-32));
#106401=DIRECTION('center_axis',(4.93038065763132E-32,1.97215226305253E-31,
-1.));
#106402=DIRECTION('ref_axis',(1.,0.,4.93038065763132E-32));
#106403=DIRECTION('center_axis',(4.93038065763132E-32,1.97215226305253E-31,
-1.));
#106404=DIRECTION('ref_axis',(-0.464722744083384,0.885456250264015,1.51712854493318E-31));
#106405=DIRECTION('',(-0.415660658584278,0.791976146676969,0.447213595499941));
#106406=DIRECTION('center_axis',(4.93038065763132E-32,1.97215226305253E-31,
-1.));
#106407=DIRECTION('ref_axis',(1.,0.,4.93038065763132E-32));
#106408=DIRECTION('',(-4.93038065763132E-32,-1.97215226305253E-31,1.));
#106409=DIRECTION('center_axis',(-4.93038065763132E-32,-1.97215226305253E-31,
1.));
#106410=DIRECTION('ref_axis',(1.,0.,4.93038065763132E-32));
#106411=DIRECTION('center_axis',(-4.93038065763132E-32,-1.97215226305253E-31,
1.));
#106412=DIRECTION('ref_axis',(1.,0.,4.93038065763132E-32));
#106413=DIRECTION('center_axis',(-4.93038065763132E-32,-1.97215226305253E-31,
1.));
#106414=DIRECTION('ref_axis',(-0.464722744083384,0.885456250264015,1.51712854493318E-31));
#106415=DIRECTION('center_axis',(4.93038065763132E-32,1.97215226305253E-31,
-1.));
#106416=DIRECTION('ref_axis',(1.,0.,4.93038065763132E-32));
#106417=DIRECTION('',(-0.415660658584274,0.791976146676961,-0.447213595499958));
#106418=DIRECTION('center_axis',(4.93038065763132E-32,1.97215226305253E-31,
-1.));
#106419=DIRECTION('ref_axis',(1.,7.65671051465626E-16,4.93038065763134E-32));
#106420=DIRECTION('center_axis',(4.93038065763132E-32,1.97215226305253E-31,
-1.));
#106421=DIRECTION('ref_axis',(1.,0.,4.93038065763132E-32));
#106422=DIRECTION('center_axis',(4.93038065763132E-32,1.97215226305253E-31,
-1.));
#106423=DIRECTION('ref_axis',(-0.464722744083384,0.885456250264015,1.51712854493318E-31));
#106424=DIRECTION('',(-0.415660658584278,0.791976146676969,0.447213595499941));
#106425=DIRECTION('center_axis',(4.93038065763132E-32,1.97215226305253E-31,
-1.));
#106426=DIRECTION('ref_axis',(1.,0.,4.93038065763132E-32));
#106427=DIRECTION('',(-4.93038065763132E-32,-1.97215226305253E-31,1.));
#106428=DIRECTION('center_axis',(-4.93038065763132E-32,-1.97215226305253E-31,
1.));
#106429=DIRECTION('ref_axis',(1.,0.,4.93038065763132E-32));
#106430=DIRECTION('center_axis',(-4.93038065763132E-32,-1.97215226305253E-31,
1.));
#106431=DIRECTION('ref_axis',(1.,0.,4.93038065763132E-32));
#106432=DIRECTION('center_axis',(-4.93038065763132E-32,-1.97215226305253E-31,
1.));
#106433=DIRECTION('ref_axis',(-0.464722744083384,0.885456250264015,1.51712854493318E-31));
#106434=DIRECTION('center_axis',(4.93038065763132E-32,1.97215226305253E-31,
-1.));
#106435=DIRECTION('ref_axis',(1.,0.,4.93038065763132E-32));
#106436=DIRECTION('',(-0.415660658584274,0.791976146676961,-0.447213595499958));
#106437=DIRECTION('center_axis',(4.93038065763132E-32,1.97215226305253E-31,
-1.));
#106438=DIRECTION('ref_axis',(1.,7.65671051465626E-16,4.93038065763134E-32));
#106439=DIRECTION('center_axis',(4.93038065763132E-32,1.97215226305253E-31,
-1.));
#106440=DIRECTION('ref_axis',(1.,0.,4.93038065763132E-32));
#106441=DIRECTION('center_axis',(4.93038065763132E-32,1.97215226305253E-31,
-1.));
#106442=DIRECTION('ref_axis',(-0.464722744083384,0.885456250264015,1.51712854493318E-31));
#106443=DIRECTION('',(-0.415660658584278,0.791976146676969,0.447213595499941));
#106444=DIRECTION('center_axis',(4.93038065763132E-32,1.97215226305253E-31,
-1.));
#106445=DIRECTION('ref_axis',(0.415323571508097,0.909673749731055,1.99878547453377E-31));
#106446=DIRECTION('center_axis',(4.93038065763132E-32,1.97215226305253E-31,
-1.));
#106447=DIRECTION('ref_axis',(1.,0.,4.93038065763132E-32));
#106448=DIRECTION('',(-4.93038065763132E-32,-1.97215226305253E-31,1.));
#106449=DIRECTION('center_axis',(4.93038065763132E-32,1.97215226305253E-31,
-1.));
#106450=DIRECTION('ref_axis',(1.,0.,4.93038065763132E-32));
#106451=DIRECTION('center_axis',(4.93038065763132E-32,1.97215226305253E-31,
-1.));
#106452=DIRECTION('ref_axis',(1.,0.,4.93038065763132E-32));
#106453=DIRECTION('center_axis',(-4.93038065763132E-32,-1.97215226305253E-31,
1.));
#106454=DIRECTION('ref_axis',(-0.464722744083384,0.885456250264015,1.51712854493318E-31));
#106455=DIRECTION('center_axis',(-4.93038065763132E-32,-1.97215226305253E-31,
1.));
#106456=DIRECTION('ref_axis',(1.,0.,4.93038065763132E-32));
#106457=DIRECTION('center_axis',(-4.93038065763132E-32,-1.97215226305253E-31,
1.));
#106458=DIRECTION('ref_axis',(1.,0.,4.93038065763132E-32));
#106459=DIRECTION('',(-0.415660658584274,0.791976146676961,-0.447213595499958));
#106460=DIRECTION('center_axis',(4.93038065763132E-32,1.97215226305253E-31,
-1.));
#106461=DIRECTION('ref_axis',(1.,7.65671051465626E-16,4.93038065763134E-32));
#106462=DIRECTION('center_axis',(4.93038065763132E-32,1.97215226305253E-31,
-1.));
#106463=DIRECTION('ref_axis',(-0.464722744083384,0.885456250264015,1.51712854493318E-31));
#106464=DIRECTION('',(-0.415660658584278,0.791976146676969,0.447213595499941));
#106465=DIRECTION('center_axis',(4.93038065763132E-32,1.97215226305253E-31,
-1.));
#106466=DIRECTION('ref_axis',(1.,0.,4.93038065763132E-32));
#106467=DIRECTION('',(-4.93038065763132E-32,-1.97215226305253E-31,1.));
#106468=DIRECTION('center_axis',(4.93038065763132E-32,1.97215226305253E-31,
-1.));
#106469=DIRECTION('ref_axis',(1.,0.,4.93038065763132E-32));
#106470=DIRECTION('',(-4.93038065763132E-32,-1.97215226305253E-31,1.));
#106471=DIRECTION('center_axis',(-0.415323571356916,-0.909673749800079,
-1.99878547459536E-31));
#106472=DIRECTION('ref_axis',(-0.909673749800079,0.415323571356916,3.70577535073674E-32));
#106473=DIRECTION('center_axis',(4.93038065763132E-32,1.97215226305253E-31,
-1.));
#106474=DIRECTION('ref_axis',(-1.,0.,-4.93038065763132E-32));
#130721=CARTESIAN_POINT('',(0.,0.,0.));
#130722=CARTESIAN_POINT('Origin',(-21.9500000210213,0.999999999999992,-6.00000000000001));
#130723=CARTESIAN_POINT('',(-21.5093868137065,-0.185251134376082,-7.65234634179685));
#130724=CARTESIAN_POINT('',(-21.5094163772775,-0.185130046756847,-7.7903497740652));
#130725=CARTESIAN_POINT('',(-21.5093868137063,-0.185251134376008,-6.00000000000001));
#130726=CARTESIAN_POINT('',(-23.2143447276962,0.9984309442522,-7.94368623524854));
#130727=CARTESIAN_POINT('Ctrl Pts',(-21.5094163780221,-0.185130047031939,
-7.79034977411791));
#130728=CARTESIAN_POINT('Ctrl Pts',(-21.5560227037756,-0.202348715799771,
-7.79364848584603));
#130729=CARTESIAN_POINT('Ctrl Pts',(-21.6036752898958,-0.21684557206526,
-7.79691771167341));
#130730=CARTESIAN_POINT('Ctrl Pts',(-21.6520290024672,-0.228522300280214,
-7.80012768793153));
#130731=CARTESIAN_POINT('Ctrl Pts',(-21.7003642493108,-0.240194569286675,
-7.80333643833655));
#130732=CARTESIAN_POINT('Ctrl Pts',(-21.7494000855687,-0.24904888749276,
-7.80648593753533));
#130733=CARTESIAN_POINT('Ctrl Pts',(-21.7987843632908,-0.255021079848016,
-7.80957109983421));
#130734=CARTESIAN_POINT('Ctrl Pts',(-21.8482059171473,-0.260997780120666,
-7.81265859086867));
#130735=CARTESIAN_POINT('Ctrl Pts',(-21.8979764202531,-0.264087851279457,
-7.81568173932712));
#130736=CARTESIAN_POINT('Ctrl Pts',(-21.9477356337069,-0.264262041475781,
-7.8186598005637));
#130737=CARTESIAN_POINT('Ctrl Pts',(-21.9975111599162,-0.264436288777552,
-7.82163883810962));
#130738=CARTESIAN_POINT('Ctrl Pts',(-22.0472753250638,-0.261692426856607,
-7.82457301529161));
#130739=CARTESIAN_POINT('Ctrl Pts',(-22.0966608194572,-0.256039733590408,
-7.82750339621611));
#130740=CARTESIAN_POINT('Ctrl Pts',(-22.1461396084972,-0.250376361763082,
-7.83043931295342));
#130741=CARTESIAN_POINT('Ctrl Pts',(-22.1952381051126,-0.241792640298569,
-7.83337189951185));
#130742=CARTESIAN_POINT('Ctrl Pts',(-22.2435819516393,-0.230342864021984,
-7.83635887232752));
#130743=CARTESIAN_POINT('Ctrl Pts',(-22.2879715574474,-0.219829611725669,
-7.83910152843317));
#130744=CARTESIAN_POINT('Ctrl Pts',(-22.3317245576032,-0.206900089373834,
-7.84189069189933));
#130745=CARTESIAN_POINT('Ctrl Pts',(-22.3745509540369,-0.191636072322134,
-7.84477645837742));
#130746=CARTESIAN_POINT('Ctrl Pts',(-22.3745684736764,-0.191629828040586,
-7.84477763890141));
#130747=CARTESIAN_POINT('Ctrl Pts',(-22.3745859931617,-0.191623583368604,
-7.84477881944157));
#130748=CARTESIAN_POINT('Ctrl Pts',(-22.3746035124926,-0.191617338306218,
-7.8447799999979));
#130749=CARTESIAN_POINT('Ctrl Pts',(-22.4174213951043,-0.176354178445099,
-7.84766532265466));
#130750=CARTESIAN_POINT('Ctrl Pts',(-22.4594737121133,-0.158695428803833,
-7.85065492207322));
#130751=CARTESIAN_POINT('Ctrl Pts',(-22.5004931234151,-0.1387643463029,
-7.85368972442065));
#130752=CARTESIAN_POINT('Ctrl Pts',(-22.5053443484456,-0.136407165562289,
-7.85404864008139));
#130753=CARTESIAN_POINT('Ctrl Pts',(-22.5101810940409,-0.134018252268478,
-7.85440818799464));
#130754=CARTESIAN_POINT('Ctrl Pts',(-22.5150028933519,-0.131597851584441,
-7.85476827044094));
#130755=CARTESIAN_POINT('Ctrl Pts',(-22.5589591683231,-0.109533101240051,
-7.85805083821301));
#130756=CARTESIAN_POINT('Ctrl Pts',(-22.6016771164603,-0.0848470764096622,
-7.86137728959589));
#130757=CARTESIAN_POINT('Ctrl Pts',(-22.6428506708358,-0.0577313326929714,
-7.86468832169072));
#130758=CARTESIAN_POINT('Ctrl Pts',(-22.6839864864387,-0.0306404426694719,
-7.86799631896649));
#130759=CARTESIAN_POINT('Ctrl Pts',(-22.7235809510388,-0.00112451343309885,
-7.8712886285325));
#130760=CARTESIAN_POINT('Ctrl Pts',(-22.7613552207452,0.0305978737586179,
-7.8745272073172));
#130761=CARTESIAN_POINT('Ctrl Pts',(-22.7991113553565,0.0623050313107944,
-7.87776423128866));
#130762=CARTESIAN_POINT('Ctrl Pts',(-22.8350490983818,0.0962164620954286,
-7.88094747473338));
#130763=CARTESIAN_POINT('Ctrl Pts',(-22.868914357826,0.1320884559541,-7.88406294348325));
#130764=CARTESIAN_POINT('Ctrl Pts',(-22.9027781399198,0.167958884919679,
-7.88717827632276));
#130765=CARTESIAN_POINT('Ctrl Pts',(-22.9345695304503,0.205789724678508,
-7.89022588030349));
#130766=CARTESIAN_POINT('Ctrl Pts',(-22.9640590917588,0.245312165147836,
-7.8932161980417));
#130767=CARTESIAN_POINT('Ctrl Pts',(-22.9935811343522,0.284878137619522,
-7.89620980946617));
#130768=CARTESIAN_POINT('Ctrl Pts',(-23.0207960397528,0.326139522802212,
-7.89914618738315));
#130769=CARTESIAN_POINT('Ctrl Pts',(-23.0455007030266,0.368800646431264,
-7.90205868834638));
#130770=CARTESIAN_POINT('Ctrl Pts',(-23.0702217701547,0.411490096973965,
-7.9049731232053));
#130771=CARTESIAN_POINT('Ctrl Pts',(-23.0924288439946,0.455581259255592,
-7.90786402195172));
#130772=CARTESIAN_POINT('Ctrl Pts',(-23.1119503464419,0.500750344982422,
-7.91078362691741));
#130773=CARTESIAN_POINT('Ctrl Pts',(-23.1302244959823,0.543033290642225,
-7.91351667975933));
#130774=CARTESIAN_POINT('Ctrl Pts',(-23.1461451885907,0.586261260105575,
-7.9162754435804));
#130775=CARTESIAN_POINT('Ctrl Pts',(-23.1596031204119,0.630143818282359,
-7.91911205284188));
#130776=CARTESIAN_POINT('Ctrl Pts',(-23.1605484930719,0.633226414575799,
-7.91931131472539));
#130777=CARTESIAN_POINT('Ctrl Pts',(-23.1614817293283,0.636312254833964,
-7.91951096074278));
#130778=CARTESIAN_POINT('Ctrl Pts',(-23.1624027985064,0.639401244864388,
-7.91971100896574));
#130779=CARTESIAN_POINT('Ctrl Pts',(-23.1660690594275,0.651696785420236,
-7.92050728898423));
#130780=CARTESIAN_POINT('Ctrl Pts',(-23.1695424991904,0.664041822917359,
-7.92130997070593));
#130781=CARTESIAN_POINT('Ctrl Pts',(-23.172821312714,0.676429714133373,
-7.92212022415011));
#130782=CARTESIAN_POINT('Ctrl Pts',(-23.1728251181124,0.676444091548047,
-7.9221211645321));
#130783=CARTESIAN_POINT('Ctrl Pts',(-23.1728289232487,0.676458469020474,
-7.92212210492429));
#130784=CARTESIAN_POINT('Ctrl Pts',(-23.1728327281229,0.676472846550637,
-7.92212304532667));
#130785=CARTESIAN_POINT('Ctrl Pts',(-23.185485780736,0.724285109732905,
-7.92525033950908));
#130786=CARTESIAN_POINT('Ctrl Pts',(-23.1952650209804,0.772848506784041,
-7.92849472874584));
#130787=CARTESIAN_POINT('Ctrl Pts',(-23.2021445513064,0.821870800689957,
-7.93179069122616));
#130788=CARTESIAN_POINT('Ctrl Pts',(-23.2043730055447,0.837750364185012,
-7.93285833701164));
#130789=CARTESIAN_POINT('Ctrl Pts',(-23.2062971123773,0.853677678218472,
-7.93393139425532));
#130790=CARTESIAN_POINT('Ctrl Pts',(-23.207915830539,0.869641649335481,
-7.9350076359548));
#130791=CARTESIAN_POINT('Ctrl Pts',(-23.2122479261328,0.912365238020205,
-7.93788792854347));
#130792=CARTESIAN_POINT('Ctrl Pts',(-23.2143946495102,0.955357932434763,
-7.94079152872966));
#130793=CARTESIAN_POINT('Ctrl Pts',(-23.2143447276962,0.998430944252203,
-7.94368623524854));
#130794=CARTESIAN_POINT('',(-22.9081161737437,1.82521129893649,-8.00000000000001));
#130795=CARTESIAN_POINT('Ctrl Pts',(-23.214499040964,0.998425654430992,
-7.94377502574648));
#130796=CARTESIAN_POINT('Ctrl Pts',(-23.2145652572834,1.05160995694309,
-7.94742259194512));
#130797=CARTESIAN_POINT('Ctrl Pts',(-23.2112760714399,1.10474931579339,
-7.95103824992359));
#130798=CARTESIAN_POINT('Ctrl Pts',(-23.2046495127751,1.15752746694461,
-7.95457642429432));
#130799=CARTESIAN_POINT('Ctrl Pts',(-23.200690529771,1.18905933951439,-7.95669027748839));
#130800=CARTESIAN_POINT('Ctrl Pts',(-23.1955440476404,1.22043256383109,
-7.95877520624573));
#130801=CARTESIAN_POINT('Ctrl Pts',(-23.1892205216726,1.25158060490748,
-7.96082825372533));
#130802=CARTESIAN_POINT('Ctrl Pts',(-23.1830565039967,1.28194294970399,
-7.96282951394283));
#130803=CARTESIAN_POINT('Ctrl Pts',(-23.1757783610785,1.3120702156534,-7.96479911529432));
#130804=CARTESIAN_POINT('Ctrl Pts',(-23.167400318562,1.34190168988727,-7.96673896897314));
#130805=CARTESIAN_POINT('Ctrl Pts',(-23.1581792637964,1.37473485552339,
-7.96887401388065));
#130806=CARTESIAN_POINT('Ctrl Pts',(-23.1476332527721,1.40718326839631,
-7.97097123410555));
#130807=CARTESIAN_POINT('Ctrl Pts',(-23.1357875330326,1.43916765176641,
-7.97303937742848));
#130808=CARTESIAN_POINT('Ctrl Pts',(-23.1223190451642,1.47553363786722,
-7.97539083971763));
#130809=CARTESIAN_POINT('Ctrl Pts',(-23.1071842951135,1.5112621136308,-7.97770216398833));
#130810=CARTESIAN_POINT('Ctrl Pts',(-23.0904306503722,1.54624008424715,
-7.97999558215418));
#130811=CARTESIAN_POINT('Ctrl Pts',(-23.0519689624722,1.62653973306939,
-7.98526062955616));
#130812=CARTESIAN_POINT('Ctrl Pts',(-23.0051370109133,1.70254619131719,
-7.99039898368457));
#130813=CARTESIAN_POINT('Ctrl Pts',(-22.9507170505117,1.77299785050667,
-7.99582789768067));
#130814=CARTESIAN_POINT('Ctrl Pts',(-22.9369822977737,1.79077875500949,
-7.99719807124974));
#130815=CARTESIAN_POINT('Ctrl Pts',(-22.9227769036649,1.80818937719799,
-7.99858622413477));
#130816=CARTESIAN_POINT('Ctrl Pts',(-22.9081161737437,1.82521129893648,
-8.));
#130817=CARTESIAN_POINT('',(-21.0014870926804,1.83623171117239,-8.00000000000001));
#130818=CARTESIAN_POINT('Origin',(-21.9500000210213,0.999999999999992,-8.00000000000001));
#130819=CARTESIAN_POINT('Ctrl Pts',(-21.0014870926799,1.83623171117168,
-8.00000000000009));
#130820=CARTESIAN_POINT('Ctrl Pts',(-21.0556763883481,1.89769702853811,
-7.99452566673546));
#130821=CARTESIAN_POINT('Ctrl Pts',(-21.115703404117,1.95374207720739,-7.98885938194356));
#130822=CARTESIAN_POINT('Ctrl Pts',(-21.213056154207,2.02836378585187,-7.98055621038558));
#130823=CARTESIAN_POINT('Ctrl Pts',(-21.2465536944085,2.05156172433473,
-7.97783121513637));
#130824=CARTESIAN_POINT('Ctrl Pts',(-21.3106622633174,2.09152175596766,
-7.97286867380942));
#130825=CARTESIAN_POINT('Ctrl Pts',(-21.340959808357,2.10871226662972,-7.97061964930845));
#130826=CARTESIAN_POINT('Ctrl Pts',(-21.3973158518954,2.13767970829369,
-7.96660205612705));
#130827=CARTESIAN_POINT('Ctrl Pts',(-21.4231368507775,2.14986534191615,
-7.96482102287359));
#130828=CARTESIAN_POINT('Ctrl Pts',(-21.4861731928968,2.17704416147748,
-7.96060134739312));
#130829=CARTESIAN_POINT('Ctrl Pts',(-21.5237330243955,2.19116126746671,
-7.95819131267466));
#130830=CARTESIAN_POINT('Ctrl Pts',(-21.6583691063655,2.23457891380381,
-7.94982112103086));
#130831=CARTESIAN_POINT('Ctrl Pts',(-21.7582174921326,2.2539741076228,-7.94411972376694));
#130832=CARTESIAN_POINT('Ctrl Pts',(-21.8895157725744,2.26341575427773,
-7.93630584710667));
#130833=CARTESIAN_POINT('Ctrl Pts',(-21.9197934212877,2.264501873635,-7.93447981764929));
#130834=CARTESIAN_POINT('Ctrl Pts',(-21.9669493180662,2.26449895246781,
-7.93155976036272));
#130835=CARTESIAN_POINT('Ctrl Pts',(-21.9838161661189,2.26416032272429,
-7.93049969359661));
#130836=CARTESIAN_POINT('Ctrl Pts',(-22.0226124674591,2.26260437420453,
-7.92801863944682));
#130837=CARTESIAN_POINT('Ctrl Pts',(-22.0445240111228,2.26115322396874,
-7.92658780616593));
#130838=CARTESIAN_POINT('Ctrl Pts',(-22.1632250073712,2.25018136775124,
-7.91871275381176));
#130839=CARTESIAN_POINT('Ctrl Pts',(-22.2587071691502,2.23008884080025,
-7.91195899415794));
#130840=CARTESIAN_POINT('Ctrl Pts',(-22.4009517577418,2.18253252411451,
-7.90184864474664));
#130841=CARTESIAN_POINT('Ctrl Pts',(-22.4498700097206,2.16270019663609,
-7.89835563899462));
#130842=CARTESIAN_POINT('Ctrl Pts',(-22.5239328467189,2.12713217698962,
-7.89305789733272));
#130843=CARTESIAN_POINT('Ctrl Pts',(-22.5500028089861,2.11347326322552,
-7.89119048019733));
#130844=CARTESIAN_POINT('Ctrl Pts',(-22.6022588512574,2.08372574464128,
-7.8874344850262));
#130845=CARTESIAN_POINT('Ctrl Pts',(-22.6283827348897,2.06756742002737,
-7.88554983023936));
#130846=CARTESIAN_POINT('Ctrl Pts',(-22.7335197672645,1.99711787732585,
-7.87790034022239));
#130847=CARTESIAN_POINT('Ctrl Pts',(-22.8068207268085,1.93488341748448,
-7.87243807537444));
#130848=CARTESIAN_POINT('Ctrl Pts',(-22.8989371498963,1.83665093413516,
-7.86464977578417));
#130849=CARTESIAN_POINT('Ctrl Pts',(-22.9241656815761,1.8071353071863,-7.8623919306256));
#130850=CARTESIAN_POINT('Ctrl Pts',(-22.9646626696585,1.75508715350208,
-7.85846180110323));
#130851=CARTESIAN_POINT('Ctrl Pts',(-22.9806344570043,1.73313664296803,
-7.85681841327607));
#130852=CARTESIAN_POINT('Ctrl Pts',(-23.0050187130218,1.69725162314212,
-7.85412509710346));
#130853=CARTESIAN_POINT('Ctrl Pts',(-23.0138897256297,1.68363947155786,
-7.85310140435618));
#130854=CARTESIAN_POINT('Ctrl Pts',(-23.0341402611235,1.6512167808574,-7.85065386673856));
#130855=CARTESIAN_POINT('Ctrl Pts',(-23.0452949934441,1.6322753712771,-7.84921881753903));
#130856=CARTESIAN_POINT('Ctrl Pts',(-23.1028803348784,1.52839144417269,
-7.84135796533044));
#130857=CARTESIAN_POINT('Ctrl Pts',(-23.139933742053,1.43862136049432,-7.83462861707198));
#130858=CARTESIAN_POINT('Ctrl Pts',(-23.1807277311189,1.2950011794314,-7.8245579547231));
#130859=CARTESIAN_POINT('Ctrl Pts',(-23.1919145282173,1.24365110826614,
-7.82107875406906));
#130860=CARTESIAN_POINT('Ctrl Pts',(-23.2043044865844,1.16288957147469,
-7.81580897792239));
#130861=CARTESIAN_POINT('Ctrl Pts',(-23.2077313062482,1.13388404288782,
-7.8139553759453));
#130862=CARTESIAN_POINT('Ctrl Pts',(-23.2126607866774,1.07460118431117,
-7.81023886929075));
#130863=CARTESIAN_POINT('Ctrl Pts',(-23.2140854828188,1.04433639642869,
-7.80837943730091));
#130864=CARTESIAN_POINT('Ctrl Pts',(-23.2150862913203,0.954254188213088,
-7.80293295978635));
#130865=CARTESIAN_POINT('Ctrl Pts',(-23.2115085428974,0.894486043265319,
-7.79943821327412));
#130866=CARTESIAN_POINT('Ctrl Pts',(-23.1955279036933,0.772920406599362,
-7.79234913308464));
#130867=CARTESIAN_POINT('Ctrl Pts',(-23.1827144823299,0.711349155456169,
-7.78876811501925));
#130868=CARTESIAN_POINT('Ctrl Pts',(-23.1556706852961,0.617173452003201,
-7.78301166934413));
#130869=CARTESIAN_POINT('Ctrl Pts',(-23.1445544577311,0.583782274133964,
-7.78091228675576));
#130870=CARTESIAN_POINT('Ctrl Pts',(-23.1259795189943,0.53489166656199,
-7.77769300599477));
#130871=CARTESIAN_POINT('Ctrl Pts',(-23.1195727673118,0.519008204948834,
-7.77662339963613));
#130872=CARTESIAN_POINT('Ctrl Pts',(-23.1051572771907,0.485262213960005,
-7.77429082755341));
#130873=CARTESIAN_POINT('Ctrl Pts',(-23.0970527916685,0.467446608869917,
-7.77302360369203));
#130874=CARTESIAN_POINT('Ctrl Pts',(-23.0561066392935,0.382711771129634,
-7.76684632678012));
#130875=CARTESIAN_POINT('Ctrl Pts',(-23.017805651613,0.318599687827898,
-7.76172380252077));
#130876=CARTESIAN_POINT('Ctrl Pts',(-22.929838491173,0.197151195717176,
-7.75149424034105));
#130877=CARTESIAN_POINT('Ctrl Pts',(-22.880209696823,0.140138106763055,
-7.74641058976998));
#130878=CARTESIAN_POINT('Ctrl Pts',(-22.8037491759279,0.0667229190159224,
-7.7395349037698));
#130879=CARTESIAN_POINT('Ctrl Pts',(-22.7809495947314,0.0463665362775556,
-7.73758457285688));
#130880=CARTESIAN_POINT('Ctrl Pts',(-22.734813362694,0.00808661056340476,
-7.73382093612577));
#130881=CARTESIAN_POINT('Ctrl Pts',(-22.7115447180439,-0.0098881306651899,
-7.73200638408686));
#130882=CARTESIAN_POINT('Ctrl Pts',(-22.6445653140699,-0.0579960945008118,
-7.72699187665342));
#130883=CARTESIAN_POINT('Ctrl Pts',(-22.5995528326252,-0.0862129826772939,
-7.72386041324328));
#130884=CARTESIAN_POINT('Ctrl Pts',(-22.4904547549625,-0.145388578462997,
-7.71663893156329));
#130885=CARTESIAN_POINT('Ctrl Pts',(-22.4252726569225,-0.1739342571129,
-7.71259883893754));
#130886=CARTESIAN_POINT('Ctrl Pts',(-22.3327810959289,-0.205467181841179,
-7.70686664940803));
#130887=CARTESIAN_POINT('Ctrl Pts',(-22.3072562013548,-0.213276696797498,
-7.70528386166558));
#130888=CARTESIAN_POINT('Ctrl Pts',(-22.2608925002553,-0.225872074130784,
-7.70237736538823));
#130889=CARTESIAN_POINT('Ctrl Pts',(-22.2401429436037,-0.230948185930413,
-7.70106544925019));
#130890=CARTESIAN_POINT('Ctrl Pts',(-22.2030075761668,-0.239041835201648,
-7.69868207233511));
#130891=CARTESIAN_POINT('Ctrl Pts',(-22.1866727945651,-0.242265421525683,
-7.69762058317892));
#130892=CARTESIAN_POINT('Ctrl Pts',(-22.1408160050136,-0.250377868835656,
-7.69460880869523));
#130893=CARTESIAN_POINT('Ctrl Pts',(-22.111178368738,-0.254542471526902,
-7.69262714430821));
#130894=CARTESIAN_POINT('Ctrl Pts',(-22.0027027415514,-0.265878073123162,
-7.68530725561696));
#130895=CARTESIAN_POINT('Ctrl Pts',(-21.9233840061674,-0.266695228159861,
-7.6798396469926));
#130896=CARTESIAN_POINT('Ctrl Pts',(-21.789564541093,-0.255492211394217,
-7.67076523367455));
#130897=CARTESIAN_POINT('Ctrl Pts',(-21.734975291159,-0.247303436806563,
-7.6671033899489));
#130898=CARTESIAN_POINT('Ctrl Pts',(-21.6522347269965,-0.229295773689886,
-7.66163623693413));
#130899=CARTESIAN_POINT('Ctrl Pts',(-21.6236073933802,-0.222006688364611,
-7.65975956079658));
#130900=CARTESIAN_POINT('Ctrl Pts',(-21.5663065847785,-0.205259094257848,
-7.65602639139567));
#130901=CARTESIAN_POINT('Ctrl Pts',(-21.5376640869836,-0.195763117627018,
-7.65417242371063));
#130902=CARTESIAN_POINT('Ctrl Pts',(-21.5093868137067,-0.185251134376157,
-7.65234634179685));
#130903=CARTESIAN_POINT('Origin',(-21.9500000210213,0.999999999999992,-6.00000000000001));
#130904=CARTESIAN_POINT('',(-21.5093868140292,-0.185251134496023,-7.15421782883515));
#130905=CARTESIAN_POINT('',(-21.5093591526456,-0.185356720995697,-7.28986799996607));
#130906=CARTESIAN_POINT('',(-21.5093868137063,-0.185251134376008,-6.00000000000001));
#130907=CARTESIAN_POINT('',(-23.2145649522473,1.00099359444644,-7.44330650983136));
#130908=CARTESIAN_POINT('Ctrl Pts',(-21.5093591533682,-0.185356721266173,
-7.28986800001162));
#130909=CARTESIAN_POINT('Ctrl Pts',(-21.5559477712327,-0.202794731700962,
-7.29280447580565));
#130910=CARTESIAN_POINT('Ctrl Pts',(-21.6035192041601,-0.217456141425245,
-7.29574978827595));
#130911=CARTESIAN_POINT('Ctrl Pts',(-21.6517131024261,-0.22921970626668,
-7.2987642189804));
#130912=CARTESIAN_POINT('Ctrl Pts',(-21.682553520669,-0.236747490338739,
-7.3006932246644));
#130913=CARTESIAN_POINT('Ctrl Pts',(-21.7136482905638,-0.24308939355335,
-7.30265082761511));
#130914=CARTESIAN_POINT('Ctrl Pts',(-21.744897502386,-0.248224113096361,
-7.30465399011448));
#130915=CARTESIAN_POINT('Ctrl Pts',(-21.7449142057305,-0.248226857709235,
-7.3046550608459));
#130916=CARTESIAN_POINT('Ctrl Pts',(-21.7449309091192,-0.248229601977445,
-7.30465613159035));
#130917=CARTESIAN_POINT('Ctrl Pts',(-21.7449476125523,-0.248232345901003,
-7.30465720234781));
#130918=CARTESIAN_POINT('Ctrl Pts',(-21.7902341497497,-0.255671702564202,
-7.30756025212355));
#130919=CARTESIAN_POINT('Ctrl Pts',(-21.8360112373321,-0.260597049194722,
-7.31056635456357));
#130920=CARTESIAN_POINT('Ctrl Pts',(-21.8819794934509,-0.262988071267566,
-7.31361640347263));
#130921=CARTESIAN_POINT('Ctrl Pts',(-21.8869280447319,-0.263245468357217,
-7.31394474578339));
#130922=CARTESIAN_POINT('Ctrl Pts',(-21.891878767541,-0.26347351898473,
-7.3142735973829));
#130923=CARTESIAN_POINT('Ctrl Pts',(-21.8968312572195,-0.263672215633016,
-7.31460288453286));
#130924=CARTESIAN_POINT('Ctrl Pts',(-21.9463665079808,-0.265659597523184,
-7.31789644446016));
#130925=CARTESIAN_POINT('Ctrl Pts',(-21.9960839415655,-0.264708253779789,
-7.32123302732497));
#130926=CARTESIAN_POINT('Ctrl Pts',(-22.0456178331554,-0.260838765858485,
-7.32455387831832));
#130927=CARTESIAN_POINT('Ctrl Pts',(-22.095105553473,-0.256972884744047,
-7.32787163389738));
#130928=CARTESIAN_POINT('Ctrl Pts',(-22.1444101675817,-0.250194598032994,
-7.33117339343978));
#130929=CARTESIAN_POINT('Ctrl Pts',(-22.1931768119306,-0.240561133120324,
-7.33442197708555));
#130930=CARTESIAN_POINT('Ctrl Pts',(-22.2419183466623,-0.230932628413967,
-7.33766888805745));
#130931=CARTESIAN_POINT('Ctrl Pts',(-22.2901224986033,-0.2184519603325,
-7.34086258283539));
#130932=CARTESIAN_POINT('Ctrl Pts',(-22.3374437766807,-0.203210226153336,
-7.34399017411066));
#130933=CARTESIAN_POINT('Ctrl Pts',(-22.3872426403831,-0.187170485178113,
-7.34728151572192));
#130934=CARTESIAN_POINT('Ctrl Pts',(-22.4360636024974,-0.168072553915644,
-7.3504994700433));
#130935=CARTESIAN_POINT('Ctrl Pts',(-22.4835147951651,-0.14606334295329,
-7.3536583656872));
#130936=CARTESIAN_POINT('Ctrl Pts',(-22.5286447817275,-0.125130773314123,
-7.35666273522874));
#130937=CARTESIAN_POINT('Ctrl Pts',(-22.5725356502153,-0.101564875153868,
-7.35961410525478));
#130938=CARTESIAN_POINT('Ctrl Pts',(-22.6148612676838,-0.0755294153820678,
-7.36254805775375));
#130939=CARTESIAN_POINT('Ctrl Pts',(-22.6572125276212,-0.0494781823385375,
-7.36548378775273));
#130940=CARTESIAN_POINT('Ctrl Pts',(-22.6979963045529,-0.0209540568645315,
-7.36840249209481));
#130941=CARTESIAN_POINT('Ctrl Pts',(-22.736900303818,0.0098381933498575,
-7.3713578778588));
#130942=CARTESIAN_POINT('Ctrl Pts',(-22.7728194553863,0.0382679569595985,
-7.37408651633313));
#130943=CARTESIAN_POINT('Ctrl Pts',(-22.8071364286681,0.0686316194067912,
-7.37684701091451));
#130944=CARTESIAN_POINT('Ctrl Pts',(-22.8396201836745,0.100731293851856,
-7.3796893756947));
#130945=CARTESIAN_POINT('Ctrl Pts',(-22.8423776955289,0.103456201510709,
-7.37993066105639));
#130946=CARTESIAN_POINT('Ctrl Pts',(-22.8451220276651,0.106193624252658,
-7.3801725363857));
#130947=CARTESIAN_POINT('Ctrl Pts',(-22.8478530557851,0.108943444354392,
-7.38041503227729));
#130948=CARTESIAN_POINT('Ctrl Pts',(-22.8531147285129,0.114241322222942,
-7.38088223142842));
#130949=CARTESIAN_POINT('Ctrl Pts',(-22.8583269358697,0.119585102091055,
-7.38135173993085));
#130950=CARTESIAN_POINT('Ctrl Pts',(-22.863488735766,0.124973820686968,
-7.38182377860623));
#130951=CARTESIAN_POINT('Ctrl Pts',(-22.8635004657162,0.124986066299377,
-7.38182485129217));
#130952=CARTESIAN_POINT('Ctrl Pts',(-22.8635121954061,0.124998312143855,
-7.38182592399117));
#130953=CARTESIAN_POINT('Ctrl Pts',(-22.8635239248358,0.125010558220377,
-7.38182699670324));
#130954=CARTESIAN_POINT('Ctrl Pts',(-22.8949165401771,0.157785925944268,
-7.38469800053578));
#130955=CARTESIAN_POINT('Ctrl Pts',(-22.9245616292306,0.192357156123483,
-7.38767052255618));
#130956=CARTESIAN_POINT('Ctrl Pts',(-22.9522727798873,0.228494562091567,
-7.39068702879009));
#130957=CARTESIAN_POINT('Ctrl Pts',(-22.954373707634,0.231234328470557,
-7.39091572595693));
#130958=CARTESIAN_POINT('Ctrl Pts',(-22.956463517418,0.233983072408943,
-7.3911446759429));
#130959=CARTESIAN_POINT('Ctrl Pts',(-22.9585421274439,0.23674068165377,
-7.39137385367572));
#130960=CARTESIAN_POINT('Ctrl Pts',(-22.9879960567569,0.275816038146746,
-7.39462130493333));
#130961=CARTESIAN_POINT('Ctrl Pts',(-23.0152020207889,0.316676836926239,
-7.39791390493542));
#130962=CARTESIAN_POINT('Ctrl Pts',(-23.0399707714754,0.359018681242872,
-7.40119395866403));
#130963=CARTESIAN_POINT('Ctrl Pts',(-23.0647157848571,0.401319946957919,
-7.40447086893029));
#130964=CARTESIAN_POINT('Ctrl Pts',(-23.0870285259997,0.445099283089772,
-7.40773496054836));
#130965=CARTESIAN_POINT('Ctrl Pts',(-23.1067566936188,0.49003959928208,
-7.4109488033226));
#130966=CARTESIAN_POINT('Ctrl Pts',(-23.1264821046171,0.534973635955073,
-7.41416219702595));
#130967=CARTESIAN_POINT('Ctrl Pts',(-23.1436237351315,0.581068267085949,
-7.4173252525692));
#130968=CARTESIAN_POINT('Ctrl Pts',(-23.1580632312311,0.627994354630757,
-7.42042358804598));
#130969=CARTESIAN_POINT('Ctrl Pts',(-23.1725011666005,0.674915370048347,
-7.42352158863119));
#130970=CARTESIAN_POINT('Ctrl Pts',(-23.1842374649771,0.722667611815115,
-7.42655492468563));
#130971=CARTESIAN_POINT('Ctrl Pts',(-23.1931878410699,0.770910674421012,
-7.42953268626117));
#130972=CARTESIAN_POINT('Ctrl Pts',(-23.2021471186336,0.81920171648744,
-7.43251340932768));
#130973=CARTESIAN_POINT('Ctrl Pts',(-23.208314693299,0.86798449478743,-7.43543862806872));
#130974=CARTESIAN_POINT('Ctrl Pts',(-23.2116425566531,0.916907003400649,
-7.43833933475804));
#130975=CARTESIAN_POINT('Ctrl Pts',(-23.2135475958525,0.944912749646556,
-7.43999984763397));
#130976=CARTESIAN_POINT('Ctrl Pts',(-23.2145227439249,0.972964093664828,
-7.44165272227882));
#130977=CARTESIAN_POINT('Ctrl Pts',(-23.2145649522472,1.00099359438948,
-7.44330650982799));
#130978=CARTESIAN_POINT('Ctrl Pts',(-23.214564952248,1.00099359495523,-7.44330650986139));
#130979=CARTESIAN_POINT('Ctrl Pts',(-23.2146393694028,1.05041219770429,
-7.44622229030034));
#130980=CARTESIAN_POINT('Ctrl Pts',(-23.2118128350904,1.09973542603955,
-7.44913831688056));
#130981=CARTESIAN_POINT('Ctrl Pts',(-23.2061009251658,1.14865878337265,
-7.45211749203754));
#130982=CARTESIAN_POINT('Ctrl Pts',(-23.2040398687697,1.16631203769178,
-7.4531924823811));
#130983=CARTESIAN_POINT('Ctrl Pts',(-23.2016030199901,1.18391370803345,
-7.4542756947842));
#130984=CARTESIAN_POINT('Ctrl Pts',(-23.1987905854071,1.20145107483144,
-7.45537008448875));
#130985=CARTESIAN_POINT('Ctrl Pts',(-23.19572307147,1.22057902802819,-7.45656373204649));
#130986=CARTESIAN_POINT('Ctrl Pts',(-23.1922094223436,1.23962911438569,
-7.45777087145966));
#130987=CARTESIAN_POINT('Ctrl Pts',(-23.1882513857817,1.25858259771115,
-7.45899564334432));
#130988=CARTESIAN_POINT('Ctrl Pts',(-23.1882479227424,1.25859918084688,
-7.45899671494462));
#130989=CARTESIAN_POINT('Ctrl Pts',(-23.1882444593629,1.25861576390876,
-7.45899778655841));
#130990=CARTESIAN_POINT('Ctrl Pts',(-23.1882409956433,1.25863234689677,
-7.45899885818571));
#130991=CARTESIAN_POINT('Ctrl Pts',(-23.178858317585,1.30355308333993,-7.46190172993643));
#130992=CARTESIAN_POINT('Ctrl Pts',(-23.1669541409773,1.34802527177939,
-7.46490770785243));
#130993=CARTESIAN_POINT('Ctrl Pts',(-23.1526174063115,1.3917624131088,-7.46795770494442));
#130994=CARTESIAN_POINT('Ctrl Pts',(-23.1510731139209,1.39647359289396,
-7.46828623772474));
#130995=CARTESIAN_POINT('Ctrl Pts',(-23.1495006350576,1.40117621164047,
-7.46861528124578));
#130996=CARTESIAN_POINT('Ctrl Pts',(-23.1479001088029,1.4058698886138,-7.46894476166106));
#130997=CARTESIAN_POINT('Ctrl Pts',(-23.1318984622988,1.45279605399784,
-7.47223882142405));
#130998=CARTESIAN_POINT('Ctrl Pts',(-23.1130894263544,1.49883274547285,
-7.4755759996429));
#130999=CARTESIAN_POINT('Ctrl Pts',(-23.0916240611239,1.54364618065664,
-7.47889751215052));
#131000=CARTESIAN_POINT('Ctrl Pts',(-23.0701787308529,1.58841778867625,
-7.48221592448409));
#131001=CARTESIAN_POINT('Ctrl Pts',(-23.0460822749542,1.63196861918501,
-7.48551840643433));
#131002=CARTESIAN_POINT('Ctrl Pts',(-23.0195160219019,1.67398824230252,
-7.48876774034043));
#131003=CARTESIAN_POINT('Ctrl Pts',(-22.9929634873123,1.7159861670407,-7.49201539633335));
#131004=CARTESIAN_POINT('Ctrl Pts',(-22.9639437641233,1.75645452377927,
-7.49520986386834));
#131005=CARTESIAN_POINT('Ctrl Pts',(-22.9326663926893,1.79510384012078,
-7.49833821419827));
#131006=CARTESIAN_POINT('Ctrl Pts',(-22.8997571778103,1.83576961854437,
-7.50162978086466));
#131007=CARTESIAN_POINT('Ctrl Pts',(-22.8643482441511,1.8744212906144,-7.5048479713041));
#131008=CARTESIAN_POINT('Ctrl Pts',(-22.8267177637578,1.91074639753886,
-7.50800705489195));
#131009=CARTESIAN_POINT('Ctrl Pts',(-22.7909220328329,1.94530040109382,
-7.51101211102989));
#131010=CARTESIAN_POINT('Ctrl Pts',(-22.7531162199469,1.97774913637893,
-7.51396410504403));
#131011=CARTESIAN_POINT('Ctrl Pts',(-22.7135706565953,2.0078473789134,-7.51689857384268));
#131012=CARTESIAN_POINT('Ctrl Pts',(-22.6740012133173,2.03796379652875,
-7.51983481464538));
#131013=CARTESIAN_POINT('Ctrl Pts',(-22.632689723638,2.06572644802876,-7.52275392175664));
#131014=CARTESIAN_POINT('Ctrl Pts',(-22.589939769477,2.09091779020453,-7.52570956219129));
#131015=CARTESIAN_POINT('Ctrl Pts',(-22.5504634189498,2.11418009009463,
-7.52843887266941));
#131016=CARTESIAN_POINT('Ctrl Pts',(-22.509759964922,2.13524983913903,-7.53119992281915));
#131017=CARTESIAN_POINT('Ctrl Pts',(-22.4680974026757,2.15398274420328,
-7.53404272752769));
#131018=CARTESIAN_POINT('Ctrl Pts',(-22.4645681084673,2.15556963492209,
-7.53428354551037));
#131019=CARTESIAN_POINT('Ctrl Pts',(-22.4610319158699,2.15713978306097,
-7.53452495016558));
#131020=CARTESIAN_POINT('Ctrl Pts',(-22.4574889786075,2.15869311549852,
-7.53476697189692));
#131021=CARTESIAN_POINT('Ctrl Pts',(-22.4506735258064,2.16168121918994,
-7.53523254257023));
#131022=CARTESIAN_POINT('Ctrl Pts',(-22.4438332508344,2.16460706131475,
-7.53570040262063));
#131023=CARTESIAN_POINT('Ctrl Pts',(-22.4369693789612,2.16747011554173,
-7.5361707705175));
#131024=CARTESIAN_POINT('Ctrl Pts',(-22.4369538236924,2.16747660394636,
-7.53617183649006));
#131025=CARTESIAN_POINT('Ctrl Pts',(-22.4369382683024,2.16748309202853,
-7.5361729024755));
#131026=CARTESIAN_POINT('Ctrl Pts',(-22.4369227127913,2.16748957978826,
-7.53617396847382));
#131027=CARTESIAN_POINT('Ctrl Pts',(-22.39454825699,2.18516275586588,-7.53907783310896));
#131028=CARTESIAN_POINT('Ctrl Pts',(-22.3511170053128,2.20050050116548,
-7.54208464648229));
#131029=CARTESIAN_POINT('Ctrl Pts',(-22.3069159212396,2.21341408117809,
-7.5451352773389));
#131030=CARTESIAN_POINT('Ctrl Pts',(-22.3021767343903,2.21479865963033,
-7.54546236229486));
#131031=CARTESIAN_POINT('Ctrl Pts',(-22.2974287453871,2.21615538274289,
-7.5457899509709));
#131032=CARTESIAN_POINT('Ctrl Pts',(-22.2926723419464,2.21748415115904,
-7.54611797048339));
#131033=CARTESIAN_POINT('Ctrl Pts',(-22.2449183024701,2.23082491591788,
-7.54941126907427));
#131034=CARTESIAN_POINT('Ctrl Pts',(-22.1963103279221,2.24134704271031,
-7.55274744660515));
#131035=CARTESIAN_POINT('Ctrl Pts',(-22.1472091448079,2.24898636163867,
-7.55606780468917));
#131036=CARTESIAN_POINT('Ctrl Pts',(-22.0981536426899,2.2566185733717,-7.55938507369762));
#131037=CARTESIAN_POINT('Ctrl Pts',(-22.0486058268957,2.26137365277867,
-7.56268625982269));
#131038=CARTESIAN_POINT('Ctrl Pts',(-21.9989242977315,2.26322557817672,
-7.56593426134831));
#131039=CARTESIAN_POINT('Ctrl Pts',(-21.9492682801424,2.26507655260697,
-7.56918059501796));
#131040=CARTESIAN_POINT('Ctrl Pts',(-21.8994786712579,2.26402743422841,
-7.57237370416246));
#131041=CARTESIAN_POINT('Ctrl Pts',(-21.8499127601215,2.26008731348708,
-7.57550079317662));
#131042=CARTESIAN_POINT('Ctrl Pts',(-21.7977645584286,2.25594191988083,
-7.57879079763499));
#131043=CARTESIAN_POINT('Ctrl Pts',(-21.7458640239365,2.24859598694143,
-7.58200754494334));
#131044=CARTESIAN_POINT('Ctrl Pts',(-21.6946261564365,2.2381021989578,-7.58516546343385));
#131045=CARTESIAN_POINT('Ctrl Pts',(-21.6458826984808,2.22811927932562,
-7.58816964519785));
#131046=CARTESIAN_POINT('Ctrl Pts',(-21.5977390586478,2.2152876048066,-7.5911210087776));
#131047=CARTESIAN_POINT('Ctrl Pts',(-21.550550456418,2.19969145104377,-7.59405522457834));
#131048=CARTESIAN_POINT('Ctrl Pts',(-21.5033332598102,2.18408584664461,
-7.5969912183948));
#131049=CARTESIAN_POINT('Ctrl Pts',(-21.4570725070522,2.16571200475415,
-7.59991045784023));
#131050=CARTESIAN_POINT('Ctrl Pts',(-21.4121194101045,2.1446973198645,-7.60286672036657));
#131051=CARTESIAN_POINT('Ctrl Pts',(-21.3706341752131,2.12530379198745,
-7.60559492495387));
#131052=CARTESIAN_POINT('Ctrl Pts',(-21.3302623001994,2.10366075919581,
-7.60835524906842));
#131053=CARTESIAN_POINT('Ctrl Pts',(-21.2912739573576,2.07990746880294,
-7.61119766217468));
#131054=CARTESIAN_POINT('Ctrl Pts',(-21.2879450475958,2.07787936105329,
-7.61144035360619));
#131055=CARTESIAN_POINT('Ctrl Pts',(-21.2846261925295,2.0758358713926,-7.61168364347605));
#131056=CARTESIAN_POINT('Ctrl Pts',(-21.2813175426721,2.07377708720797,
-7.61192756288755));
#131057=CARTESIAN_POINT('Ctrl Pts',(-21.2750097212594,2.06985208954314,
-7.61239258643285));
#131058=CARTESIAN_POINT('Ctrl Pts',(-21.2687390975643,2.06587159496297,
-7.61285990383907));
#131059=CARTESIAN_POINT('Ctrl Pts',(-21.2625067931607,2.06183631316588,
-7.61332973251004));
#131060=CARTESIAN_POINT('Ctrl Pts',(-21.2624924207027,2.06182700731134,
-7.61333081599256));
#131061=CARTESIAN_POINT('Ctrl Pts',(-21.2624780484484,2.06181770116543,
-7.61333189948843));
#131062=CARTESIAN_POINT('Ctrl Pts',(-21.262463676398,2.06180839472818,-7.61333298299766));
#131063=CARTESIAN_POINT('Ctrl Pts',(-21.2239835549963,2.03689108484768,
-7.61623400026946));
#131064=CARTESIAN_POINT('Ctrl Pts',(-21.1868270745706,2.00978717511707,
-7.6192381826602));
#131065=CARTESIAN_POINT('Ctrl Pts',(-21.1512291127379,1.98068235067877,
-7.62228642094879));
#131066=CARTESIAN_POINT('Ctrl Pts',(-21.1473532623951,1.9775134629681,-7.62261830836052));
#131067=CARTESIAN_POINT('Ctrl Pts',(-21.1434959046142,1.97432090331687,
-7.62295071803349));
#131068=CARTESIAN_POINT('Ctrl Pts',(-21.139657354002,1.97110494676656,-7.62328357367537));
#131069=CARTESIAN_POINT('Ctrl Pts',(-21.1016922462611,1.93929759309203,
-7.62657567571661));
#131070=CARTESIAN_POINT('Ctrl Pts',(-21.0655642803586,1.90519630825761,
-7.62991085463807));
#131071=CARTESIAN_POINT('Ctrl Pts',(-21.0315299705495,1.86906168717004,
-7.63323029595846));
#131072=CARTESIAN_POINT('Ctrl Pts',(-20.9975273948489,1.83296075855307,
-7.63654664218125));
#131073=CARTESIAN_POINT('Ctrl Pts',(-20.9656143026336,1.79483044489107,
-7.63984698647441));
#131074=CARTESIAN_POINT('Ctrl Pts',(-20.9360145328724,1.75495119320424,
-7.6430940527343));
#131075=CARTESIAN_POINT('Ctrl Pts',(-20.9064299391394,1.71509238791451,
-7.64633945419851));
#131076=CARTESIAN_POINT('Ctrl Pts',(-20.8791562220223,1.67348647321077,
-7.64953153657534));
#131077=CARTESIAN_POINT('Ctrl Pts',(-20.8543874954893,1.63043266892735,
-7.65265728570438));
#131078=CARTESIAN_POINT('Ctrl Pts',(-20.8296210733621,1.58738287023691,
-7.65578274402337));
#131079=CARTESIAN_POINT('Ctrl Pts',(-20.807359269724,1.54288543394258,-7.65884193058603));
#131080=CARTESIAN_POINT('Ctrl Pts',(-20.7877665861249,1.49725860380221,
-7.661846368462));
#131081=CARTESIAN_POINT('Ctrl Pts',(-20.7681549102342,1.4515875450057,-7.6648537187088));
#131082=CARTESIAN_POINT('Ctrl Pts',(-20.7512177926814,1.40478485484132,
-7.66780640875322));
#131083=CARTESIAN_POINT('Ctrl Pts',(-20.7370879415237,1.35718935752958,
-7.6707387833695));
#131084=CARTESIAN_POINT('Ctrl Pts',(-20.7229496925521,1.30956557272042,
-7.67367290078801));
#131085=CARTESIAN_POINT('Ctrl Pts',(-20.7116225068754,1.26114801133181,
-7.67658707574696));
#131086=CARTESIAN_POINT('Ctrl Pts',(-20.703201683773,1.21229639639102,-7.67953414160623));
#131087=CARTESIAN_POINT('Ctrl Pts',(-20.6953790276158,1.16691491981061,
-7.6822718648204));
#131088=CARTESIAN_POINT('Ctrl Pts',(-20.6900646801056,1.1211584099592,-7.68503854900198));
#131089=CARTESIAN_POINT('Ctrl Pts',(-20.687299148992,1.0753326793911,-7.68788495294579));
#131090=CARTESIAN_POINT('Ctrl Pts',(-20.6870826550185,1.07174530535956,
-7.68810777788419));
#131091=CARTESIAN_POINT('Ctrl Pts',(-20.6868817645872,1.06815748613482,
-7.68833109136304));
#131092=CARTESIAN_POINT('Ctrl Pts',(-20.6866964891666,1.06456935749218,
-7.68855491773312));
#131093=CARTESIAN_POINT('Ctrl Pts',(-20.6861601106909,1.05418160629602,
-7.6892029024837));
#131094=CARTESIAN_POINT('Ctrl Pts',(-20.6857545740246,1.043791532,-7.68985520057486));
#131095=CARTESIAN_POINT('Ctrl Pts',(-20.6854800248292,1.03340277176877,
-7.69051241219103));
#131096=CARTESIAN_POINT('Ctrl Pts',(-20.6854795792906,1.03338591287967,
-7.69051347871461));
#131097=CARTESIAN_POINT('Ctrl Pts',(-20.6854791340968,1.03336905399399,
-7.69051454525113));
#131098=CARTESIAN_POINT('Ctrl Pts',(-20.685478689248,1.03335219511177,-7.69051561180059));
#131099=CARTESIAN_POINT('Ctrl Pts',(-20.68426768411,0.987457518912684,-7.6934190630238));
#131100=CARTESIAN_POINT('Ctrl Pts',(-20.6856160866493,0.941419909381913,
-7.69642583461519));
#131101=CARTESIAN_POINT('Ctrl Pts',(-20.6895030751693,0.895538674509048,
-7.69947695126876));
#131102=CARTESIAN_POINT('Ctrl Pts',(-20.6899194512904,0.890623854074188,
-7.69980378838462));
#131103=CARTESIAN_POINT('Ctrl Pts',(-20.6903649281569,0.885710867824233,
-7.70013113435119));
#131104=CARTESIAN_POINT('Ctrl Pts',(-20.6908394585241,0.880800111615071,
-7.70045891667684));
#131105=CARTESIAN_POINT('Ctrl Pts',(-20.6956140374226,0.831389589990802,
-7.70375696182499));
#131106=CARTESIAN_POINT('Ctrl Pts',(-20.7033327684018,0.782199754485548,
-7.70709862514005));
#131107=CARTESIAN_POINT('Ctrl Pts',(-20.7139251171565,0.733591049100032,
-7.71042500202741));
#131108=CARTESIAN_POINT('Ctrl Pts',(-20.7245075061223,0.685028049577832,
-7.71374825118433));
#131109=CARTESIAN_POINT('Ctrl Pts',(-20.7379578231943,0.63704495025831,
-7.71705594647716));
#131110=CARTESIAN_POINT('Ctrl Pts',(-20.7541707021653,0.589986349436577,
-7.72031073035324));
#131111=CARTESIAN_POINT('Ctrl Pts',(-20.7703750410767,0.542952536516657,
-7.72356379978687));
#131112=CARTESIAN_POINT('Ctrl Pts',(-20.789338961905,0.496842201669888,
-7.7267639173308));
#131113=CARTESIAN_POINT('Ctrl Pts',(-20.8109248380533,0.451986005087727,
-7.72989801760503));
#131114=CARTESIAN_POINT('Ctrl Pts',(-20.8335840862821,0.404899304229897,
-7.73318796310456));
#131115=CARTESIAN_POINT('Ctrl Pts',(-20.8591329218472,0.359194773336397,
-7.73640499458669));
#131116=CARTESIAN_POINT('Ctrl Pts',(-20.8873736002875,0.315238832915532,
-7.73956310094918));
#131117=CARTESIAN_POINT('Ctrl Pts',(-20.9142987152029,0.273330535650482,
-7.74257409011167));
#131118=CARTESIAN_POINT('Ctrl Pts',(-20.9436706362759,0.233011785794678,
-7.7455319278408));
#131119=CARTESIAN_POINT('Ctrl Pts',(-20.9752824841326,0.194584241866766,
-7.7484719707215));
#131120=CARTESIAN_POINT('Ctrl Pts',(-21.006912832425,0.156134208702855,
-7.75141373422526));
#131121=CARTESIAN_POINT('Ctrl Pts',(-21.0407860208494,0.119577973306089,
-7.75433809542381));
#131122=CARTESIAN_POINT('Ctrl Pts',(-21.0766564070754,0.0851979572082941,
-7.75729853809533));
#131123=CARTESIAN_POINT('Ctrl Pts',(-21.1097881797831,0.0534427686284415,
-7.76003295843553));
#131124=CARTESIAN_POINT('Ctrl Pts',(-21.1446243140553,0.0235440379982971,
-7.76279874938703));
#131125=CARTESIAN_POINT('Ctrl Pts',(-21.1809367785472,-0.00429528527658141,
-7.76564580898741));
#131126=CARTESIAN_POINT('Ctrl Pts',(-21.1840016610854,-0.0066450089038303,
-7.76588610948412));
#131127=CARTESIAN_POINT('Ctrl Pts',(-21.1870770699707,-0.0089800909533138,
-7.76612698892844));
#131128=CARTESIAN_POINT('Ctrl Pts',(-21.1901628736014,-0.0113004255346918,
-7.76636847732289));
#131129=CARTESIAN_POINT('Ctrl Pts',(-21.195838300467,-0.0155679975503176,
-7.76681262409486));
#131130=CARTESIAN_POINT('Ctrl Pts',(-21.201548775814,-0.0197856245643231,
-7.76725883603628));
#131131=CARTESIAN_POINT('Ctrl Pts',(-21.2072933722109,-0.0239526163666588,
-7.76770730157324));
#131132=CARTESIAN_POINT('Ctrl Pts',(-21.2073066081804,-0.0239622174199971,
-7.76770833487058));
#131133=CARTESIAN_POINT('Ctrl Pts',(-21.2073198443311,-0.0239718182045455,
-7.76770936817989));
#131134=CARTESIAN_POINT('Ctrl Pts',(-21.2073330806628,-0.0239814187202979,
-7.76771040150115));
#131135=CARTESIAN_POINT('Ctrl Pts',(-21.2445607881007,-0.0509832495781172,
-7.77061665850255));
#131136=CARTESIAN_POINT('Ctrl Pts',(-21.2833587804813,-0.0759491526982826,
-7.77362476915587));
#131137=CARTESIAN_POINT('Ctrl Pts',(-21.3234665167027,-0.098725861531078,
-7.77667545105122));
#131138=CARTESIAN_POINT('Ctrl Pts',(-21.3265580603532,-0.100481512590064,
-7.77691060060419));
#131139=CARTESIAN_POINT('Ctrl Pts',(-21.3296573601806,-0.102224157158229,
-7.77714600309324));
#131140=CARTESIAN_POINT('Ctrl Pts',(-21.3327642840652,-0.103953725668209,
-7.77738163136852));
#131141=CARTESIAN_POINT('Ctrl Pts',(-21.376109675984,-0.128083323849993,
-7.78066893428247));
#131142=CARTESIAN_POINT('Ctrl Pts',(-21.4209445151194,-0.149668228400233,
-7.7839995919757));
#131143=CARTESIAN_POINT('Ctrl Pts',(-21.4669324790524,-0.168561791557893,
-7.78731487504472));
#131144=CARTESIAN_POINT('Ctrl Pts',(-21.4809893493312,-0.17433687581252,
-7.78832823810872));
#131145=CARTESIAN_POINT('Ctrl Pts',(-21.4951538992482,-0.179860785953845,
-7.78934030157835));
#131146=CARTESIAN_POINT('Ctrl Pts',(-21.5094163772775,-0.18513004675685,
-7.79034977406521));
#131147=CARTESIAN_POINT('Ctrl Pts',(-21.5093868137067,-0.185251134376157,
-7.65234634179685));
#131148=CARTESIAN_POINT('Ctrl Pts',(-21.5093128480698,-0.185223637894142,
-7.65234156526446));
#131149=CARTESIAN_POINT('Ctrl Pts',(-21.509238884932,-0.185196134460566,
-7.65233678892048));
#131150=CARTESIAN_POINT('Ctrl Pts',(-21.4510434928494,-0.163549787454182,
-7.64857870542183));
#131151=CARTESIAN_POINT('Ctrl Pts',(-21.3945883018176,-0.137683887915379,
-7.64495533318918));
#131152=CARTESIAN_POINT('Ctrl Pts',(-21.2863501577122,-0.0781071893864338,
-7.63781023021484));
#131153=CARTESIAN_POINT('Ctrl Pts',(-21.2346855626873,-0.0445433913468252,
-7.63429654681614));
#131154=CARTESIAN_POINT('Ctrl Pts',(-21.1579041077945,0.0137144298681591,
-7.62862794366726));
#131155=CARTESIAN_POINT('Ctrl Pts',(-21.1310219340692,0.0359203108878381,
-7.62654580317381));
#131156=CARTESIAN_POINT('Ctrl Pts',(-21.0923432432901,0.0706567948773928,
-7.62334378722566));
#131157=CARTESIAN_POINT('Ctrl Pts',(-21.0798274758663,0.0823651831614658,
-7.62227282675557));
#131158=CARTESIAN_POINT('Ctrl Pts',(-21.053424423381,0.108091031660806,
-7.61992833542388));
#131159=CARTESIAN_POINT('Ctrl Pts',(-21.0396202195877,0.12218571245985,
-7.61865021649861));
#131160=CARTESIAN_POINT('Ctrl Pts',(-20.9935903068346,0.171438038912264,
-7.61422250868857));
#131161=CARTESIAN_POINT('Ctrl Pts',(-20.9630278008428,0.20809116472436,
-7.61099322679332));
#131162=CARTESIAN_POINT('Ctrl Pts',(-20.8949084606398,0.29987162568279,
-7.60320127747352));
#131163=CARTESIAN_POINT('Ctrl Pts',(-20.8594929686099,0.356421459397041,
-7.59863436844913));
#131164=CARTESIAN_POINT('Ctrl Pts',(-20.8132087185071,0.445213092888341,
-7.59193440148952));
#131165=CARTESIAN_POINT('Ctrl Pts',(-20.7989066664431,0.475531357136871,
-7.58972102651659));
#131166=CARTESIAN_POINT('Ctrl Pts',(-20.7737610005966,0.53483648235841,
-7.58553587033554));
#131167=CARTESIAN_POINT('Ctrl Pts',(-20.7627434091212,0.563723338294082,
-7.5835600388979));
#131168=CARTESIAN_POINT('Ctrl Pts',(-20.7434424683484,0.620495943478359,
-7.57979047079808));
#131169=CARTESIAN_POINT('Ctrl Pts',(-20.7350406710656,0.648320546348082,
-7.57799402259526));
#131170=CARTESIAN_POINT('Ctrl Pts',(-20.71487682135,0.724492028471393,-7.57319542971564));
#131171=CARTESIAN_POINT('Ctrl Pts',(-20.704996179733,0.773284073757678,
-7.57025088306412));
#131172=CARTESIAN_POINT('Ctrl Pts',(-20.6874731010391,0.896906627558796,
-7.56296848958778));
#131173=CARTESIAN_POINT('Ctrl Pts',(-20.683579241259,0.972066347095177,
-7.55870572283618));
#131174=CARTESIAN_POINT('Ctrl Pts',(-20.687799559305,1.08523111887321,-7.55207258970493));
#131175=CARTESIAN_POINT('Ctrl Pts',(-20.6909435456879,1.12325029369719,
-7.54980526507213));
#131176=CARTESIAN_POINT('Ctrl Pts',(-20.6980259515646,1.17840015803419,
-7.54638822984118));
#131177=CARTESIAN_POINT('Ctrl Pts',(-20.7006111008889,1.19568590989837,
-7.54529854448084));
#131178=CARTESIAN_POINT('Ctrl Pts',(-20.70677304212,1.2317596251916,-7.54297547560186));
#131179=CARTESIAN_POINT('Ctrl Pts',(-20.7104193626123,1.25053051708427,
-7.5417393621425));
#131180=CARTESIAN_POINT('Ctrl Pts',(-20.7246473159491,1.31582812592224,
-7.53735964333183));
#131181=CARTESIAN_POINT('Ctrl Pts',(-20.7374346160178,1.36183015848023,
-7.5341327517182));
#131182=CARTESIAN_POINT('Ctrl Pts',(-20.7745565649186,1.47102742105603,
-7.52627390124519));
#131183=CARTESIAN_POINT('Ctrl Pts',(-20.8014278417162,1.53321397034375,
-7.52163491577533));
#131184=CARTESIAN_POINT('Ctrl Pts',(-20.8489477410753,1.62271968376971,
-7.51485171981006));
#131185=CARTESIAN_POINT('Ctrl Pts',(-20.8659348897925,1.65184278272168,
-7.51262475197985));
#131186=CARTESIAN_POINT('Ctrl Pts',(-20.9007519695144,1.70639986519932,
-7.50841839191507));
#131187=CARTESIAN_POINT('Ctrl Pts',(-20.9183947454039,1.73192421582375,
-7.50643478318591));
#131188=CARTESIAN_POINT('Ctrl Pts',(-20.9543374638286,1.78003810793221,
-7.50265830531034));
#131189=CARTESIAN_POINT('Ctrl Pts',(-20.9725123016609,1.80269629318323,
-7.50086245105653));
#131190=CARTESIAN_POINT('Ctrl Pts',(-21.0236277815069,1.86210702135917,
-7.49608800789188));
#131191=CARTESIAN_POINT('Ctrl Pts',(-21.0579659069959,1.89759115647615,
-7.49316564719757));
#131192=CARTESIAN_POINT('Ctrl Pts',(-21.1499307329358,1.9821202753915,-7.48587650808767));
#131193=CARTESIAN_POINT('Ctrl Pts',(-21.2100388991139,2.02816732924938,
-7.48158794822996));
#131194=CARTESIAN_POINT('Ctrl Pts',(-21.296982874725,2.08317828786665,-7.47556149025012));
#131195=CARTESIAN_POINT('Ctrl Pts',(-21.3205352869499,2.09703262517965,
-7.4739438021616));
#131196=CARTESIAN_POINT('Ctrl Pts',(-21.3635559169022,2.12049716782942,
-7.47098307056637));
#131197=CARTESIAN_POINT('Ctrl Pts',(-21.3828580838653,2.13038952792014,
-7.46965260643455));
#131198=CARTESIAN_POINT('Ctrl Pts',(-21.4173154645289,2.14694424479858,
-7.46725760019654));
#131199=CARTESIAN_POINT('Ctrl Pts',(-21.4323641988047,2.15381410324062,
-7.46620405613973));
#131200=CARTESIAN_POINT('Ctrl Pts',(-21.4741114699702,2.1718910349841,-7.46326462807476));
#131201=CARTESIAN_POINT('Ctrl Pts',(-21.5010656623271,2.18247883336374,
-7.46134987780624));
#131202=CARTESIAN_POINT('Ctrl Pts',(-21.6033286098363,2.21864803269781,
-7.45407955987269));
#131203=CARTESIAN_POINT('Ctrl Pts',(-21.6806335164803,2.23803312710359,
-7.44858492562844));
#131204=CARTESIAN_POINT('Ctrl Pts',(-21.798601560024,2.25603485389948,-7.440515329707));
#131205=CARTESIAN_POINT('Ctrl Pts',(-21.8382195982436,2.26017880398547,
-7.43785432010282));
#131206=CARTESIAN_POINT('Ctrl Pts',(-21.9121184193655,2.26439517210371,
-7.43299655949922));
#131207=CARTESIAN_POINT('Ctrl Pts',(-21.946334149411,2.2649573398176,-7.43078902702736));
#131208=CARTESIAN_POINT('Ctrl Pts',(-22.0087315120385,2.2634502239286,-7.42683450174997));
#131209=CARTESIAN_POINT('Ctrl Pts',(-22.0369006154249,2.26182579380693,
-7.42507566455904));
#131210=CARTESIAN_POINT('Ctrl Pts',(-22.1043473439633,2.25566666981565,
-7.42091574432761));
#131211=CARTESIAN_POINT('Ctrl Pts',(-22.1435132377278,2.25022995576206,
-7.41854266342653));
#131212=CARTESIAN_POINT('Ctrl Pts',(-22.2704368832692,2.22650256725899,
-7.41091220876748));
#131213=CARTESIAN_POINT('Ctrl Pts',(-22.3565077899392,2.20072452498635,
-7.40584924890605));
#131214=CARTESIAN_POINT('Ctrl Pts',(-22.465886440877,2.15484340357353,-7.3989214784988));
#131215=CARTESIAN_POINT('Ctrl Pts',(-22.4922466068292,2.14270317193148,
-7.39720917694569));
#131216=CARTESIAN_POINT('Ctrl Pts',(-22.5383232603339,2.11952900541771,
-7.39410139725384));
#131217=CARTESIAN_POINT('Ctrl Pts',(-22.558205766686,2.10885303674972,-7.39272060157604));
#131218=CARTESIAN_POINT('Ctrl Pts',(-22.5920355531881,2.08950443854627,
-7.39028359658388));
#131219=CARTESIAN_POINT('Ctrl Pts',(-22.6061183725347,2.08108193923269,
-7.38924083654891));
#131220=CARTESIAN_POINT('Ctrl Pts',(-22.6431720870343,2.05793060827983,
-7.38642314567974));
#131221=CARTESIAN_POINT('Ctrl Pts',(-22.6658355054383,2.04272911982829,
-7.3846237033285));
#131222=CARTESIAN_POINT('Ctrl Pts',(-22.7572247189644,1.97704583085346,
-7.37709999255782));
#131223=CARTESIAN_POINT('Ctrl Pts',(-22.8212506335037,1.92040917538642,
-7.37119834080684));
#131224=CARTESIAN_POINT('Ctrl Pts',(-22.9052763692649,1.82939589070396,
-7.36283540900043));
#131225=CARTESIAN_POINT('Ctrl Pts',(-22.9301513626988,1.79984635806805,
-7.36026001192446));
#131226=CARTESIAN_POINT('Ctrl Pts',(-22.9740680342113,1.74254496491024,
-7.35552955680058));
#131227=CARTESIAN_POINT('Ctrl Pts',(-22.9934301718599,1.71508193014595,
-7.35336510357126));
#131228=CARTESIAN_POINT('Ctrl Pts',(-23.0270378623879,1.66313602362411,
-7.34944986184622));
#131229=CARTESIAN_POINT('Ctrl Pts',(-23.0415986212628,1.63888385892045,
-7.34768880532691));
#131230=CARTESIAN_POINT('Ctrl Pts',(-23.0750806023269,1.57862486948262,
-7.34345998022255));
#131231=CARTESIAN_POINT('Ctrl Pts',(-23.0931022476479,1.54215386032964,
-7.34102321569987));
#131232=CARTESIAN_POINT('Ctrl Pts',(-23.1443560744998,1.42446052567096,
-7.33345141585946));
#131233=CARTESIAN_POINT('Ctrl Pts',(-23.1709128055311,1.34062394588982,
-7.328492951158));
#131234=CARTESIAN_POINT('Ctrl Pts',(-23.1943824618809,1.22650020510776,
-7.32168560447237));
#131235=CARTESIAN_POINT('Ctrl Pts',(-23.1992187795557,1.19809672397422,
-7.31998496927588));
#131236=CARTESIAN_POINT('Ctrl Pts',(-23.2060921657341,1.14729946626292,
-7.31689526533917));
#131237=CARTESIAN_POINT('Ctrl Pts',(-23.2085098817673,1.12496959265478,
-7.31552061435563));
#131238=CARTESIAN_POINT('Ctrl Pts',(-23.2116640666705,1.08621956374519,
-7.31308895189193));
#131239=CARTESIAN_POINT('Ctrl Pts',(-23.2126772837488,1.06982843393177,
-7.31204509285436));
#131240=CARTESIAN_POINT('Ctrl Pts',(-23.2145314387803,1.02598028471857,
-7.30921417255426));
#131241=CARTESIAN_POINT('Ctrl Pts',(-23.2147973285713,0.998509380542609,
-7.3074021279492));
#131242=CARTESIAN_POINT('Ctrl Pts',(-23.2123334479862,0.890904014894769,
-7.30020459773971));
#131243=CARTESIAN_POINT('Ctrl Pts',(-23.2028802398318,0.811111535271158,
-7.29466403780639));
#131244=CARTESIAN_POINT('Ctrl Pts',(-23.1738147555945,0.676693413761247,
-7.28535531233618));
#131245=CARTESIAN_POINT('Ctrl Pts',(-23.1578923622944,0.621519951837084,
-7.28153872289362));
#131246=CARTESIAN_POINT('Ctrl Pts',(-23.1281229394914,0.539708387752511,
-7.27591270783948));
#131247=CARTESIAN_POINT('Ctrl Pts',(-23.1169889697294,0.512169085648075,
-7.27402397704424));
#131248=CARTESIAN_POINT('Ctrl Pts',(-23.0926636182677,0.457614320444355,
-7.27028577726325));
#131249=CARTESIAN_POINT('Ctrl Pts',(-23.0794582857638,0.430626159808112,
-7.26843821782838));
#131250=CARTESIAN_POINT('Ctrl Pts',(-23.0153806046644,0.310690073313094,
-7.26020026219811));
#131251=CARTESIAN_POINT('Ctrl Pts',(-22.9539151000919,0.223894592919347,
-7.25420360320425));
#131252=CARTESIAN_POINT('Ctrl Pts',(-22.8491318254017,0.10952865726046,
-7.24520234435516));
#131253=CARTESIAN_POINT('Ctrl Pts',(-22.813837741004,0.0752510174626142,
-7.24231659755144));
#131254=CARTESIAN_POINT('Ctrl Pts',(-22.7627146329513,0.0310862001168211,
-7.2381843280834));
#131255=CARTESIAN_POINT('Ctrl Pts',(-22.7485269620261,0.0193606015539327,
-7.23704203663595));
#131256=CARTESIAN_POINT('Ctrl Pts',(-22.7199392281353,-0.00323435670909866,
-7.23473782211452));
#131257=CARTESIAN_POINT('Ctrl Pts',(-22.7055524116394,-0.0141134290087086,
-7.23357685387326));
#131258=CARTESIAN_POINT('Ctrl Pts',(-22.6612846585523,-0.0461231219848734,
-7.23001230202803));
#131259=CARTESIAN_POINT('Ctrl Pts',(-22.630715726351,-0.0662669117592296,
-7.22756153146986));
#131260=CARTESIAN_POINT('Ctrl Pts',(-22.5330388149527,-0.124718759276647,
-7.21985299147399));
#131261=CARTESIAN_POINT('Ctrl Pts',(-22.4632587741855,-0.158228408759995,
-7.21452800356339));
#131262=CARTESIAN_POINT('Ctrl Pts',(-22.3456686073162,-0.201969702661744,
-7.20610337869806));
#131263=CARTESIAN_POINT('Ctrl Pts',(-22.2995520214518,-0.216182172964166,
-7.20292312325515));
#131264=CARTESIAN_POINT('Ctrl Pts',(-22.2246434384929,-0.234653053251299,
-7.19795982609677));
#131265=CARTESIAN_POINT('Ctrl Pts',(-22.1963241977393,-0.240613468952686,
-7.19612777170259));
#131266=CARTESIAN_POINT('Ctrl Pts',(-22.1370813601368,-0.250973542719044,
-7.19237882547494));
#131267=CARTESIAN_POINT('Ctrl Pts',(-22.10614903939,-0.255209925563125,
-7.19046796589624));
#131268=CARTESIAN_POINT('Ctrl Pts',(-21.9765490294657,-0.268093689543489,
-7.18261589499013));
#131269=CARTESIAN_POINT('Ctrl Pts',(-21.8772009745272,-0.266281092757907,
-7.17699752398702));
#131270=CARTESIAN_POINT('Ctrl Pts',(-21.7439922827288,-0.248108567641219,
-7.1692039962486));
#131271=CARTESIAN_POINT('Ctrl Pts',(-21.7091247077903,-0.24185063319301,
-7.16713536098795));
#131272=CARTESIAN_POINT('Ctrl Pts',(-21.6495482977929,-0.228554502269538,
-7.16348626729058));
#131273=CARTESIAN_POINT('Ctrl Pts',(-21.6247062113893,-0.222211580319089,
-7.16192942345191));
#131274=CARTESIAN_POINT('Ctrl Pts',(-21.5843858365215,-0.210600311004532,
-7.15931959009562));
#131275=CARTESIAN_POINT('Ctrl Pts',(-21.5687871891666,-0.205779236362664,
-7.15828840693354));
#131276=CARTESIAN_POINT('Ctrl Pts',(-21.5385579660834,-0.195791061480555,
-7.15624577799516));
#131277=CARTESIAN_POINT('Ctrl Pts',(-21.5239226312969,-0.190654776703856,
-7.15523709376975));
#131278=CARTESIAN_POINT('Ctrl Pts',(-21.509386814352,-0.185251134616039,
-7.15421782883515));
#131279=CARTESIAN_POINT('Origin',(-21.9500000210213,0.999999999999992,-6.00000000000001));
#131280=CARTESIAN_POINT('',(-21.5093868153863,-0.18525113500052,-6.6522544014516));
#131281=CARTESIAN_POINT('',(-21.5094433440835,-0.185020348671028,-6.79053824099259));
#131282=CARTESIAN_POINT('',(-21.5093868137063,-0.185251134376008,-6.00000000000001));
#131283=CARTESIAN_POINT('',(-23.2143063419907,0.999065236394241,-6.94375433137471));
#131284=CARTESIAN_POINT('Ctrl Pts',(-21.5094433447348,-0.185020348911781,
-6.79053824103847));
#131285=CARTESIAN_POINT('Ctrl Pts',(-21.5560295243835,-0.202240840674773,
-6.79382015535907));
#131286=CARTESIAN_POINT('Ctrl Pts',(-21.603654065421,-0.216746349867037,
-6.79706007406326));
#131287=CARTESIAN_POINT('Ctrl Pts',(-21.6519736785055,-0.228436706932433,
-6.80023581525148));
#131288=CARTESIAN_POINT('Ctrl Pts',(-21.7002809854702,-0.240124086678163,
-6.80341074763663));
#131289=CARTESIAN_POINT('Ctrl Pts',(-21.7492830036594,-0.248997715194778,
-6.80652153338587));
#131290=CARTESIAN_POINT('Ctrl Pts',(-21.7986280584045,-0.254991264796082,
-6.80957069021685));
#131291=CARTESIAN_POINT('Ctrl Pts',(-21.8480147108248,-0.260989866934682,
-6.81262241747432));
#131292=CARTESIAN_POINT('Ctrl Pts',(-21.8977449542218,-0.264103330875337,
-6.81561254855112));
#131293=CARTESIAN_POINT('Ctrl Pts',(-21.9474577719668,-0.264300760927358,
-6.81856734041095));
#131294=CARTESIAN_POINT('Ctrl Pts',(-21.9971927366036,-0.264498278933798,
-6.82152344862055));
#131295=CARTESIAN_POINT('Ctrl Pts',(-22.0469101804872,-0.261776790501234,
-6.82444450254065));
#131296=CARTESIAN_POINT('Ctrl Pts',(-22.0962408692552,-0.256145263090496,
-6.82737719120075));
#131297=CARTESIAN_POINT('Ctrl Pts',(-22.1456589885209,-0.250503754727602,
-6.8303150775671));
#131298=CARTESIAN_POINT('Ctrl Pts',(-22.1946887394418,-0.241941306091203,
-6.83326520328801));
#131299=CARTESIAN_POINT('Ctrl Pts',(-22.2429534108828,-0.230514129940558,
-6.83628844575657));
#131300=CARTESIAN_POINT('Ctrl Pts',(-22.2708986835911,-0.223897788333286,
-6.83803890489625));
#131301=CARTESIAN_POINT('Ctrl Pts',(-22.29858737022,-0.216321987947828,
-6.83981410345112));
#131302=CARTESIAN_POINT('Ctrl Pts',(-22.3259462504358,-0.207806132960166,
-6.84162661025685));
#131303=CARTESIAN_POINT('Ctrl Pts',(-22.3259624236005,-0.207801098824114,
-6.84162768171777));
#131304=CARTESIAN_POINT('Ctrl Pts',(-22.3259785966501,-0.207796064359656,
-6.84162875319173));
#131305=CARTESIAN_POINT('Ctrl Pts',(-22.3259947695848,-0.207791029566808,
-6.84162982467873));
#131306=CARTESIAN_POINT('Ctrl Pts',(-22.3698112732581,-0.194150523147158,
-6.84453274953983));
#131307=CARTESIAN_POINT('Ctrl Pts',(-22.4129399665384,-0.178042987725401,
-6.8475387403743));
#131308=CARTESIAN_POINT('Ctrl Pts',(-22.4551041379781,-0.159584384076933,
-6.85058869343851));
#131309=CARTESIAN_POINT('Ctrl Pts',(-22.4596460256163,-0.157596039450061,
-6.85091723171274));
#131310=CARTESIAN_POINT('Ctrl Pts',(-22.4641766927377,-0.155580455081427,
-6.85124628009874));
#131311=CARTESIAN_POINT('Ctrl Pts',(-22.4686957735709,-0.153537805872149,
-6.8515757647222));
#131312=CARTESIAN_POINT('Ctrl Pts',(-22.5138689232656,-0.13311929557977,
-6.85486932347165));
#131313=CARTESIAN_POINT('Ctrl Pts',(-22.5578882557163,-0.10999210798179,
-6.85820592152001));
#131314=CARTESIAN_POINT('Ctrl Pts',(-22.6004360534522,-0.0843385029327583,
-6.86152679697928));
#131315=CARTESIAN_POINT('Ctrl Pts',(-22.6429441827154,-0.0587088154396544,
-6.86484457629575));
#131316=CARTESIAN_POINT('Ctrl Pts',(-22.6839837385748,-0.0305576463727556,
-6.86814636878));
#131317=CARTESIAN_POINT('Ctrl Pts',(-22.7232631349714,-9.51512544804245E-5,
-6.87139498460364));
#131318=CARTESIAN_POINT('Ctrl Pts',(-22.7625223016828,0.0303516550615235,
-6.87464192732429));
#131319=CARTESIAN_POINT('Ctrl Pts',(-22.8000231848581,0.0631073546523845,
-6.87783565303744));
#131320=CARTESIAN_POINT('Ctrl Pts',(-22.835497755303,0.0979357123471776,
-6.88096326252241));
#131321=CARTESIAN_POINT('Ctrl Pts',(-22.8728317763673,0.134589648490881,
-6.88425481015578));
#131322=CARTESIAN_POINT('Ctrl Pts',(-22.9079211560354,0.173539537848562,
-6.88747294771169));
#131323=CARTESIAN_POINT('Ctrl Pts',(-22.9404813706637,0.214478419093898,
-6.89063199209422));
#131324=CARTESIAN_POINT('Ctrl Pts',(-22.9714470610841,0.253412459832623,
-6.89363633317399));
#131325=CARTESIAN_POINT('Ctrl Pts',(-23.0001252022708,0.294145335391891,
-6.89658764971792));
#131326=CARTESIAN_POINT('Ctrl Pts',(-23.0262976368862,0.336384522477805,
-6.89952151269442));
#131327=CARTESIAN_POINT('Ctrl Pts',(-23.0524859312349,0.378649305281093,
-6.90245715350645));
#131328=CARTESIAN_POINT('Ctrl Pts',(-23.0761650308708,0.422422377383413,
-6.90537573239366));
#131329=CARTESIAN_POINT('Ctrl Pts',(-23.0971475208172,0.467380767602949,
-6.90833094800898));
#131330=CARTESIAN_POINT('Ctrl Pts',(-23.1165213823974,0.508892410463372,
-6.91105960120586));
#131331=CARTESIAN_POINT('Ctrl Pts',(-23.1335962467152,0.551415101151114,
-6.91382007620338));
#131332=CARTESIAN_POINT('Ctrl Pts',(-23.1482542287364,0.594668377259283,
-6.91666239450767));
#131333=CARTESIAN_POINT('Ctrl Pts',(-23.1494975356539,0.598337169956046,
-6.9169034832199));
#131334=CARTESIAN_POINT('Ctrl Pts',(-23.1507234790972,0.60201123727547,
-6.91714516076426));
#131335=CARTESIAN_POINT('Ctrl Pts',(-23.1519320008278,0.605690418647588,
-6.9173874576667));
#131336=CARTESIAN_POINT('Ctrl Pts',(-23.1542648310407,0.612792405518175,
-6.9178551675309));
#131337=CARTESIAN_POINT('Ctrl Pts',(-23.1565327240052,0.619913307396138,
-6.9183251911209));
#131338=CARTESIAN_POINT('Ctrl Pts',(-23.1587352677353,0.627051836558025,
-6.91879775004721));
#131339=CARTESIAN_POINT('Ctrl Pts',(-23.1587402617275,0.627068022279061,
-6.91879882151541));
#131340=CARTESIAN_POINT('Ctrl Pts',(-23.1587452553836,0.627084208090731,
-6.91879989299664));
#131341=CARTESIAN_POINT('Ctrl Pts',(-23.1587502487039,0.627100393993012,
-6.9188009644909));
#131342=CARTESIAN_POINT('Ctrl Pts',(-23.1730618829199,0.673491713118847,
-6.92187203408926));
#131343=CARTESIAN_POINT('Ctrl Pts',(-23.1846450412562,0.720746808245064,
-6.92505497657824));
#131344=CARTESIAN_POINT('Ctrl Pts',(-23.1934542128594,0.768570359867943,
-6.92828320901063));
#131345=CARTESIAN_POINT('Ctrl Pts',(-23.1953339441314,0.778775113455718,
-6.92897206032716));
#131346=CARTESIAN_POINT('Ctrl Pts',(-23.1970873498032,0.789005562115176,
-6.92966297380755));
#131347=CARTESIAN_POINT('Ctrl Pts',(-23.198713972783,0.799258529773055,
-6.93035530253995));
#131348=CARTESIAN_POINT('Ctrl Pts',(-23.2067014127284,0.849605146319679,
-6.93375494353926));
#131349=CARTESIAN_POINT('Ctrl Pts',(-23.2116327500809,0.900501157908817,
-6.93718796717115));
#131350=CARTESIAN_POINT('Ctrl Pts',(-23.2134794075178,0.951614527615504,
-6.94059891598172));
#131351=CARTESIAN_POINT('Ctrl Pts',(-23.2137476794667,0.95903998890203,
-6.94109443933478));
#131352=CARTESIAN_POINT('Ctrl Pts',(-23.2139508123716,0.966469956080461,
-6.94158949680679));
#131353=CARTESIAN_POINT('Ctrl Pts',(-23.2140886840524,0.973903326322752,
-6.94208391836729));
#131354=CARTESIAN_POINT('Ctrl Pts',(-23.2142441750389,0.982286643806755,
-6.94264152451061));
#131355=CARTESIAN_POINT('Ctrl Pts',(-23.2143167590587,0.990674437415963,
-6.94319838748987));
#131356=CARTESIAN_POINT('Ctrl Pts',(-23.2143063419907,0.999065236394238,
-6.94375433137472));
#131357=CARTESIAN_POINT('Ctrl Pts',(-23.2143063419899,0.999065237017194,
-6.94375433141597));
#131358=CARTESIAN_POINT('Ctrl Pts',(-23.2142449304963,1.04853129529665,
-6.94703177289403));
#131359=CARTESIAN_POINT('Ctrl Pts',(-23.2112979786896,1.09803111854625,
-6.95027178254654));
#131360=CARTESIAN_POINT('Ctrl Pts',(-23.2054908873639,1.1472102603586,-6.95344951713272));
#131361=CARTESIAN_POINT('Ctrl Pts',(-23.1996856242933,1.19637391902914,
-6.95662625126802));
#131362=CARTESIAN_POINT('Ctrl Pts',(-23.1910220147896,1.24521707334982,
-6.95974073011287));
#131363=CARTESIAN_POINT('Ctrl Pts',(-23.1795602753263,1.29338964514839,
-6.9627924293001));
#131364=CARTESIAN_POINT('Ctrl Pts',(-23.1680890707961,1.34160199769903,
-6.96584664857053));
#131365=CARTESIAN_POINT('Ctrl Pts',(-23.1538149580717,1.38914256170667,
-6.96883810142336));
#131366=CARTESIAN_POINT('Ctrl Pts',(-23.1368344520235,1.4356653418018,-6.97178988093841));
#131367=CARTESIAN_POINT('Ctrl Pts',(-23.119847002301,1.48220714600778,-6.97474286749614));
#131368=CARTESIAN_POINT('Ctrl Pts',(-23.1001506564016,1.52773013236868,
-6.97765643608188));
#131369=CARTESIAN_POINT('Ctrl Pts',(-23.0778815359588,1.57189502631101,
-6.98057434528757));
#131370=CARTESIAN_POINT('Ctrl Pts',(-23.0555709030587,1.61614224920202,
-6.98349769384511));
#131371=CARTESIAN_POINT('Ctrl Pts',(-23.0306774731456,1.65902590948432,
-6.98642591920524));
#131372=CARTESIAN_POINT('Ctrl Pts',(-23.0033831563308,1.70021640929234,
-6.98941774821354));
#131373=CARTESIAN_POINT('Ctrl Pts',(-22.9838335136706,1.72971923794742,
-6.99156065541322));
#131374=CARTESIAN_POINT('Ctrl Pts',(-22.9630530934144,1.75835361120176,
-6.99373656868135));
#131375=CARTESIAN_POINT('Ctrl Pts',(-22.941124785344,1.78600440442,-6.99596889953907));
#131376=CARTESIAN_POINT('Ctrl Pts',(-22.9411142602947,1.7860176761217,-6.99596997100306));
#131377=CARTESIAN_POINT('Ctrl Pts',(-22.9411037349809,1.78603094759722,
-6.99597104248005));
#131378=CARTESIAN_POINT('Ctrl Pts',(-22.9410932094026,1.78604421884654,
-6.99597211397003));
#131379=CARTESIAN_POINT('Ctrl Pts',(-22.912576857981,1.82199926106907,-6.99887504095237));
#131380=CARTESIAN_POINT('Ctrl Pts',(-22.8820072023488,1.85642353740065,
-7.0018810339252));
#131381=CARTESIAN_POINT('Ctrl Pts',(-22.8495921433793,1.88910073118473,
-7.00493098947793));
#131382=CARTESIAN_POINT('Ctrl Pts',(-22.8461004042992,1.89262070733762,
-7.00525952964829));
#131383=CARTESIAN_POINT('Ctrl Pts',(-22.8425873003403,1.89612039899188,
-7.00558857993955));
#131384=CARTESIAN_POINT('Ctrl Pts',(-22.8390531264866,1.89959952799682,
-7.0059180664767));
#131385=CARTESIAN_POINT('Ctrl Pts',(-22.803725316634,1.9343771063016,-7.00921163329467));
#131386=CARTESIAN_POINT('Ctrl Pts',(-22.766286751363,1.9671021311174,-7.01254823995152));
#131387=CARTESIAN_POINT('Ctrl Pts',(-22.7270219553802,1.99754393105081,
-7.01586912436756));
#131388=CARTESIAN_POINT('Ctrl Pts',(-22.6877937667188,2.02795734951106,
-7.01918691265946));
#131389=CARTESIAN_POINT('Ctrl Pts',(-22.646742884109,2.05609208436683,-7.02248871446112));
#131390=CARTESIAN_POINT('Ctrl Pts',(-22.6041704344222,2.08175189380834,
-7.02573733960189));
#131391=CARTESIAN_POINT('Ctrl Pts',(-22.5616199101788,2.10739848806722,
-7.02898429165251));
#131392=CARTESIAN_POINT('Ctrl Pts',(-22.5175494119718,2.1305727835755,-7.03217802669126));
#131393=CARTESIAN_POINT('Ctrl Pts',(-22.4722759027838,2.15110991198693,
-7.03530564507152));
#131394=CARTESIAN_POINT('Ctrl Pts',(-22.4246294094362,2.17272348181581,
-7.03859719571607));
#131395=CARTESIAN_POINT('Ctrl Pts',(-22.3756503149998,2.19141575935739,
-7.04181533609651));
#131396=CARTESIAN_POINT('Ctrl Pts',(-22.3257274976715,2.20703198304337,
-7.04497438246277));
#131397=CARTESIAN_POINT('Ctrl Pts',(-22.2782493866987,2.22188348463761,
-7.04797873121496));
#131398=CARTESIAN_POINT('Ctrl Pts',(-22.229917840384,2.23395283501891,-7.05093005445304));
#131399=CARTESIAN_POINT('Ctrl Pts',(-22.1810843510732,2.24314197341103,
-7.0538639226357));
#131400=CARTESIAN_POINT('Ctrl Pts',(-22.1322212702386,2.25233668012545,
-7.05679956864811));
#131401=CARTESIAN_POINT('Ctrl Pts',(-22.0828556587913,2.25864720832972,
-7.05971815124153));
#131402=CARTESIAN_POINT('Ctrl Pts',(-22.0333563299529,2.26201514749797,
-7.06267336862066));
#131403=CARTESIAN_POINT('Ctrl Pts',(-21.987651789829,2.26512488887148,-7.06540202887625));
#131404=CARTESIAN_POINT('Ctrl Pts',(-21.9418327785334,2.26572573150678,
-7.06816250939777));
#131405=CARTESIAN_POINT('Ctrl Pts',(-21.89620339875,2.26380880003273,-7.07100483175053));
#131406=CARTESIAN_POINT('Ctrl Pts',(-21.8923331613894,2.26364620786417,
-7.07124591462768));
#131407=CARTESIAN_POINT('Ctrl Pts',(-21.8884642621432,2.26346551897568,
-7.07148758629616));
#131408=CARTESIAN_POINT('Ctrl Pts',(-21.8845968717678,2.26326673691656,
-7.07172987727963));
#131409=CARTESIAN_POINT('Ctrl Pts',(-21.8771317025742,2.26288303070643,
-7.07219756815386));
#131410=CARTESIAN_POINT('Ctrl Pts',(-21.8696722944172,2.26243193962731,
-7.07266757251858));
#131411=CARTESIAN_POINT('Ctrl Pts',(-21.8622199967995,2.26191354350392,
-7.07314011195715));
#131412=CARTESIAN_POINT('Ctrl Pts',(-21.8622031005723,2.26191236816994,
-7.07314118332253));
#131413=CARTESIAN_POINT('Ctrl Pts',(-21.8621862043817,2.26191119248999,
-7.07314225470095));
#131414=CARTESIAN_POINT('Ctrl Pts',(-21.8621693082276,2.26191001646409,
-7.07314332609239));
#131415=CARTESIAN_POINT('Ctrl Pts',(-21.8163890542696,2.25872356562301,
-7.07604626911741));
#131416=CARTESIAN_POINT('Ctrl Pts',(-21.7707101713037,2.25297796441622,
-7.07905227638415));
#131417=CARTESIAN_POINT('Ctrl Pts',(-21.7254286398517,2.24472235522329,
-7.08210224404713));
#131418=CARTESIAN_POINT('Ctrl Pts',(-21.7205513644241,2.24383314325175,
-7.08243075617693));
#131419=CARTESIAN_POINT('Ctrl Pts',(-21.7156787362091,2.24291484448638,
-7.08275977831116));
#131420=CARTESIAN_POINT('Ctrl Pts',(-21.7108111513254,2.24196754490119,
-7.08308923659407));
#131421=CARTESIAN_POINT('Ctrl Pts',(-21.6621503478251,2.23249747708056,
-7.08638280109261));
#131422=CARTESIAN_POINT('Ctrl Pts',(-21.6139887726528,2.22012582692901,
-7.08971940313857));
#131423=CARTESIAN_POINT('Ctrl Pts',(-21.5666775724656,2.20495681385013,
-7.0930402816706));
#131424=CARTESIAN_POINT('Ctrl Pts',(-21.5194104800731,2.18980194270201,
-7.09635806417826));
#131425=CARTESIAN_POINT('Ctrl Pts',(-21.4729920172914,2.17185519352251,
-7.09965985893461));
#131426=CARTESIAN_POINT('Ctrl Pts',(-21.4277543235725,2.15125394795828,
-7.1029084772408));
#131427=CARTESIAN_POINT('Ctrl Pts',(-21.3825399271753,2.13066331199429,
-7.10615542251506));
#131428=CARTESIAN_POINT('Ctrl Pts',(-21.338505034419,2.1074209788545,-7.10934915099599));
#131429=CARTESIAN_POINT('Ctrl Pts',(-21.2959648649725,2.08169513258941,
-7.11247676481419));
#131430=CARTESIAN_POINT('Ctrl Pts',(-21.2511953191224,2.05462108777754,
-7.11576828555935));
#131431=CARTESIAN_POINT('Ctrl Pts',(-21.2080815227602,2.02479601831224,
-7.11898639941982));
#131432=CARTESIAN_POINT('Ctrl Pts',(-21.166971020738,1.99245313066713,-7.12214542445695));
#131433=CARTESIAN_POINT('Ctrl Pts',(-21.1278733914934,1.96169383151852,
-7.12514977574436));
#131434=CARTESIAN_POINT('Ctrl Pts',(-21.0905877461024,1.9286573436738,-7.12810110538412));
#131435=CARTESIAN_POINT('Ctrl Pts',(-21.055393731583,1.89357810922764,-7.1310349855263));
#131436=CARTESIAN_POINT('Ctrl Pts',(-21.0201783912629,1.85847761853181,
-7.13397064345211));
#131437=CARTESIAN_POINT('Ctrl Pts',(-20.987057620879,1.82133165357159,-7.13688924355075));
#131438=CARTESIAN_POINT('Ctrl Pts',(-20.9562881608786,1.78241136479329,
-7.13984448534541));
#131439=CARTESIAN_POINT('Ctrl Pts',(-20.9278778618936,1.74647517869324,
-7.14257314236305));
#131440=CARTESIAN_POINT('Ctrl Pts',(-20.9014720289848,1.70902582344569,
-7.14533362496862));
#131441=CARTESIAN_POINT('Ctrl Pts',(-20.8772499490538,1.67030908489392,
-7.14817595367336));
#131442=CARTESIAN_POINT('Ctrl Pts',(-20.8751952104047,1.66702477655643,
-7.14841706602456));
#131443=CARTESIAN_POINT('Ctrl Pts',(-20.8731561573652,1.66373133608191,
-7.14865876733914));
#131444=CARTESIAN_POINT('Ctrl Pts',(-20.8711328836023,1.66042890635819,
-7.14890108815111));
#131445=CARTESIAN_POINT('Ctrl Pts',(-20.8672284359895,1.65405598535886,
-7.14936871093808));
#131446=CARTESIAN_POINT('Ctrl Pts',(-20.863382803979,1.64764972012479,-7.14983864665092));
#131447=CARTESIAN_POINT('Ctrl Pts',(-20.8595966845555,1.64121126826339,
-7.15031111676707));
#131448=CARTESIAN_POINT('Ctrl Pts',(-20.859588097591,1.64119666577696,-7.15031218833499));
#131449=CARTESIAN_POINT('Ctrl Pts',(-20.8595795109326,1.64118206312495,
-7.15031325991594));
#131450=CARTESIAN_POINT('Ctrl Pts',(-20.8595709245804,1.6411674603074,-7.15031433150994));
#131451=CARTESIAN_POINT('Ctrl Pts',(-20.8363107889786,1.60160892540201,
-7.15321724310814));
#131452=CARTESIAN_POINT('Ctrl Pts',(-20.8152185566105,1.5606868361378,-7.15622322004602));
#131453=CARTESIAN_POINT('Ctrl Pts',(-20.7964210724615,1.5186730818474,-7.15927315818181));
#131454=CARTESIAN_POINT('Ctrl Pts',(-20.7943960233729,1.51414694876722,
-7.15960172738783));
#131455=CARTESIAN_POINT('Ctrl Pts',(-20.7923976004164,1.50960819559947,
-7.15993080679469));
#131456=CARTESIAN_POINT('Ctrl Pts',(-20.7904259567716,1.50505719785523,
-7.16026032250563));
#131457=CARTESIAN_POINT('Ctrl Pts',(-20.7707192361575,1.45956964674653,
-7.16355385583285));
#131458=CARTESIAN_POINT('Ctrl Pts',(-20.7536878133768,1.41285302912484,
-7.16689042625828));
#131459=CARTESIAN_POINT('Ctrl Pts',(-20.7394443043776,1.36525587718589,
-7.17021127213291));
#131460=CARTESIAN_POINT('Ctrl Pts',(-20.725214074249,1.31770309889276,-7.17352902206518));
#131461=CARTESIAN_POINT('Ctrl Pts',(-20.713766247517,1.26927144844836,-7.17683078321331));
#131462=CARTESIAN_POINT('Ctrl Pts',(-20.7051753409973,1.22031253559512,
-7.18007936578263));
#131463=CARTESIAN_POINT('Ctrl Pts',(-20.6965888582513,1.1713788334866,-7.18332627553731));
#131464=CARTESIAN_POINT('Ctrl Pts',(-20.690856271928,1.12191840822583,-7.18651996635826));
#131465=CARTESIAN_POINT('Ctrl Pts',(-20.6880171262504,1.07228633367087,
-7.18964753880948));
#131466=CARTESIAN_POINT('Ctrl Pts',(-20.6850290984163,1.02005159932611,
-7.19293911824876));
#131467=CARTESIAN_POINT('Ctrl Pts',(-20.6852463899028,0.967626732948496,
-7.19615728196852));
#131468=CARTESIAN_POINT('Ctrl Pts',(-20.6886731968112,0.915430274980151,
-7.19931634765498));
#131469=CARTESIAN_POINT('Ctrl Pts',(-20.6919321189101,0.865791005856937,
-7.20232064560722));
#131470=CARTESIAN_POINT('Ctrl Pts',(-20.6980937253409,0.816358423504461,
-7.20527191696333));
#131471=CARTESIAN_POINT('Ctrl Pts',(-20.7071227968265,0.767495730525501,
-7.20820573284366));
#131472=CARTESIAN_POINT('Ctrl Pts',(-20.7161573411168,0.718603420329508,
-7.21114132700219));
#131473=CARTESIAN_POINT('Ctrl Pts',(-20.7280632629945,0.670281881205839,
-7.21405985729603));
#131474=CARTESIAN_POINT('Ctrl Pts',(-20.7427621154086,0.622896180656631,
-7.21701502282478));
#131475=CARTESIAN_POINT('Ctrl Pts',(-20.7563341399243,0.579143112632761,
-7.2197436425751));
#131476=CARTESIAN_POINT('Ctrl Pts',(-20.7722876411628,0.536187529397152,
-7.22250408312399));
#131477=CARTESIAN_POINT('Ctrl Pts',(-20.7905212898478,0.494316287094292,
-7.22534636758163));
#131478=CARTESIAN_POINT('Ctrl Pts',(-20.7920678026586,0.490764918208087,
-7.22558743997484));
#131479=CARTESIAN_POINT('Ctrl Pts',(-20.7936307122051,0.487221319441231,
-7.22582910113882));
#131480=CARTESIAN_POINT('Ctrl Pts',(-20.7952099536369,0.483685648775972,
-7.22607138159539));
#131481=CARTESIAN_POINT('Ctrl Pts',(-20.7982598732763,0.476857363256427,
-7.22653928720367));
#131482=CARTESIAN_POINT('Ctrl Pts',(-20.80137062829,0.470058766383288,-7.22700950854635));
#131483=CARTESIAN_POINT('Ctrl Pts',(-20.8045416570145,0.463291089899534,
-7.22748226752908));
#131484=CARTESIAN_POINT('Ctrl Pts',(-20.8045488444521,0.463275750318491,
-7.22748333908219));
#131485=CARTESIAN_POINT('Ctrl Pts',(-20.8045560321993,0.463260410896288,
-7.22748441064832));
#131486=CARTESIAN_POINT('Ctrl Pts',(-20.8045632202561,0.463245071632921,
-7.2274854822275));
#131487=CARTESIAN_POINT('Ctrl Pts',(-20.8240114079387,0.421742774148196,
-7.23038477385445));
#131488=CARTESIAN_POINT('Ctrl Pts',(-20.8458043791237,0.381254595946671,
-7.2333869234291));
#131489=CARTESIAN_POINT('Ctrl Pts',(-20.8697899143661,0.342038658312353,
-7.23643293100584));
#131490=CARTESIAN_POINT('Ctrl Pts',(-20.8717022609837,0.338912004479815,
-7.23667578663644));
#131491=CARTESIAN_POINT('Ctrl Pts',(-20.8736285207544,0.33579345045752,
-7.23691892106093));
#131492=CARTESIAN_POINT('Ctrl Pts',(-20.8755686037111,0.33268313320659,
-7.23716230437709));
#131493=CARTESIAN_POINT('Ctrl Pts',(-20.9018047885627,0.290621602765477,
-7.24045363253935));
#131494=CARTESIAN_POINT('Ctrl Pts',(-20.9305736436336,0.250063409448494,
-7.24378987693124));
#131495=CARTESIAN_POINT('Ctrl Pts',(-20.9616520724195,0.211299434332199,
-7.24711174941872));
#131496=CARTESIAN_POINT('Ctrl Pts',(-20.992699333437,0.172574334623922,
-7.2504302904845));
#131497=CARTESIAN_POINT('Ctrl Pts',(-21.0260513365441,0.13563960361652,
-7.25373418844991));
#131498=CARTESIAN_POINT('Ctrl Pts',(-21.0614608676151,0.100756275337532,
-7.2569856166907));
#131499=CARTESIAN_POINT('Ctrl Pts',(-21.096860231571,0.0658829630853506,
-7.26023611135107));
#131500=CARTESIAN_POINT('Ctrl Pts',(-21.1343158966728,0.0330598020658376,
-7.26343406581022));
#131501=CARTESIAN_POINT('Ctrl Pts',(-21.1735578102251,0.00252106949673933,
-7.26656589599353));
#131502=CARTESIAN_POINT('Ctrl Pts',(-21.2127920393362,-0.0280116829080256,
-7.2696971128947));
#131503=CARTESIAN_POINT('Ctrl Pts',(-21.2538118480952,-0.0562608153356255,
-7.27276227829597));
#131504=CARTESIAN_POINT('Ctrl Pts',(-21.2963243649257,-0.0820188275929159,
-7.27577239800271));
#131505=CARTESIAN_POINT('Ctrl Pts',(-21.3388708395068,-0.107797414594285,
-7.27878492210472));
#131506=CARTESIAN_POINT('Ctrl Pts',(-21.3829124909228,-0.131080651973798,
-7.28174250519655));
#131507=CARTESIAN_POINT('Ctrl Pts',(-21.4281318499633,-0.151689722525295,
-7.28467903974164));
#131508=CARTESIAN_POINT('Ctrl Pts',(-21.4548209426474,-0.163853481715013,
-7.28641222314599));
#131509=CARTESIAN_POINT('Ctrl Pts',(-21.4819198346416,-0.175086248582036,
-7.28813850257311));
#131510=CARTESIAN_POINT('Ctrl Pts',(-21.5093591526456,-0.185356720995693,
-7.28986799996607));
#131511=CARTESIAN_POINT('Ctrl Pts',(-21.509386814352,-0.185251134616039,
-7.15421782883515));
#131512=CARTESIAN_POINT('Ctrl Pts',(-21.5016774549677,-0.182385205649202,
-7.15367724142142));
#131513=CARTESIAN_POINT('Ctrl Pts',(-21.4939960892933,-0.179444071264868,
-7.15313367548889));
#131514=CARTESIAN_POINT('Ctrl Pts',(-21.3984015600881,-0.141768165447487,
-7.14631135305286));
#131515=CARTESIAN_POINT('Ctrl Pts',(-21.3146239355693,-0.0973573701928965,
-7.13974825563708));
#131516=CARTESIAN_POINT('Ctrl Pts',(-21.1935796470064,-0.0146430459551139,
-7.12986617254163));
#131517=CARTESIAN_POINT('Ctrl Pts',(-21.1524347699526,0.0173693226557914,
-7.12641723933394));
#131518=CARTESIAN_POINT('Ctrl Pts',(-21.0914272581765,0.0711997026116773,
-7.12117157061882));
#131519=CARTESIAN_POINT('Ctrl Pts',(-21.0701549147649,0.0913251467019993,
-7.11931373171925));
#131520=CARTESIAN_POINT('Ctrl Pts',(-21.028125205139,0.133950077260687,
-7.11557493377509));
#131521=CARTESIAN_POINT('Ctrl Pts',(-21.0074474826271,0.156500985871011,
-7.11369793648784));
#131522=CARTESIAN_POINT('Ctrl Pts',(-20.9399338930674,0.235717198332699,
-7.10740756164589));
#131523=CARTESIAN_POINT('Ctrl Pts',(-20.8972267836028,0.295704817465734,
-7.10315118273114));
#131524=CARTESIAN_POINT('Ctrl Pts',(-20.8333695615624,0.404306469890634,
-7.09588505622193));
#131525=CARTESIAN_POINT('Ctrl Pts',(-20.8096126817668,0.451155232483091,
-7.09287091813559));
#131526=CARTESIAN_POINT('Ctrl Pts',(-20.7761000912601,0.528880138576766,
-7.08787325911741));
#131527=CARTESIAN_POINT('Ctrl Pts',(-20.7644968367809,0.558891358881146,
-7.08594367180285));
#131528=CARTESIAN_POINT('Ctrl Pts',(-20.7485773888549,0.605249507993371,
-7.0829179856093));
#131529=CARTESIAN_POINT('Ctrl Pts',(-20.7434230764883,0.621296491904699,
-7.08186232598506));
#131530=CARTESIAN_POINT('Ctrl Pts',(-20.732727322013,0.657034019461213,
-7.07948530689958));
#131531=CARTESIAN_POINT('Ctrl Pts',(-20.7273401899309,0.676764309323121,
-7.07815729456183));
#131532=CARTESIAN_POINT('Ctrl Pts',(-20.6985124526237,0.793408050978592,
-7.07024756323032));
#131533=CARTESIAN_POINT('Ctrl Pts',(-20.6861227969027,0.892688016810053,
-7.06331200549673));
#131534=CARTESIAN_POINT('Ctrl Pts',(-20.6852927256059,1.03064934568806,
-7.0540021627203));
#131535=CARTESIAN_POINT('Ctrl Pts',(-20.6867988707224,1.06889974822124,
-7.05145126892799));
#131536=CARTESIAN_POINT('Ctrl Pts',(-20.6928651361649,1.14031504612222,
-7.04675734061466));
#131537=CARTESIAN_POINT('Ctrl Pts',(-20.6970112183015,1.17348144629345,
-7.04460530062357));
#131538=CARTESIAN_POINT('Ctrl Pts',(-20.7070879228682,1.23437365440404,
-7.04070093915766));
#131539=CARTESIAN_POINT('Ctrl Pts',(-20.7126459622716,1.26213854913644,
-7.03893881521513));
#131540=CARTESIAN_POINT('Ctrl Pts',(-20.7285317639935,1.32963475836402,
-7.03468684187248));
#131541=CARTESIAN_POINT('Ctrl Pts',(-20.7398707521148,1.36909537250101,
-7.0322289968299));
#131542=CARTESIAN_POINT('Ctrl Pts',(-20.7812107170666,1.49038695999193,
-7.02467493624276));
#131543=CARTESIAN_POINT('Ctrl Pts',(-20.8177547302236,1.56970867679766,
-7.01974972480851));
#131544=CARTESIAN_POINT('Ctrl Pts',(-20.8827946522328,1.67946388168013,
-7.01229494176093));
#131545=CARTESIAN_POINT('Ctrl Pts',(-20.905086953342,1.71327032962481,-7.00989549970564));
#131546=CARTESIAN_POINT('Ctrl Pts',(-20.9394080518768,1.76024853949107,
-7.00632464563028));
#131547=CARTESIAN_POINT('Ctrl Pts',(-20.9501555968803,1.77432877205982,
-7.00522169222732));
#131548=CARTESIAN_POINT('Ctrl Pts',(-20.9729101552694,1.8028753965415,-7.00290680536955));
#131549=CARTESIAN_POINT('Ctrl Pts',(-20.9849508885042,1.81730874680709,
-7.00169319230561));
#131550=CARTESIAN_POINT('Ctrl Pts',(-21.0350672371991,1.87473185839483,
-6.99670432905464));
#131551=CARTESIAN_POINT('Ctrl Pts',(-21.0757267801254,1.9153704359689,-6.99279993910671));
#131552=CARTESIAN_POINT('Ctrl Pts',(-21.1894280937915,2.01450513059718,
-6.98250186255384));
#131553=CARTESIAN_POINT('Ctrl Pts',(-21.2664535980987,2.06792306168562,
-6.97613524836282));
#131554=CARTESIAN_POINT('Ctrl Pts',(-21.3757443544581,2.12700391817905,
-6.96806792084893));
#131555=CARTESIAN_POINT('Ctrl Pts',(-21.4033444568525,2.14064689971433,
-6.96610134778188));
#131556=CARTESIAN_POINT('Ctrl Pts',(-21.4580076576159,2.16522693070633,
-6.96233527624186));
#131557=CARTESIAN_POINT('Ctrl Pts',(-21.4850054194939,2.1762612427356,-6.9605335530104));
#131558=CARTESIAN_POINT('Ctrl Pts',(-21.5599512854856,2.20390827574016,
-6.95567124426099));
#131559=CARTESIAN_POINT('Ctrl Pts',(-21.6085561264379,2.21858523083194,
-6.952671421686));
#131560=CARTESIAN_POINT('Ctrl Pts',(-21.7434312675698,2.25060575674037,
-6.94459283559037));
#131561=CARTESIAN_POINT('Ctrl Pts',(-21.8308242804758,2.26193527433161,
-6.93963404642151));
#131562=CARTESIAN_POINT('Ctrl Pts',(-21.9472291852791,2.26481942129707,
-6.93271586244532));
#131563=CARTESIAN_POINT('Ctrl Pts',(-21.9757926830589,2.2645593434174,-6.93099183634112));
#131564=CARTESIAN_POINT('Ctrl Pts',(-22.0208120821806,2.26262360784871,
-6.92819989584836));
#131565=CARTESIAN_POINT('Ctrl Pts',(-22.0372856779751,2.26159181437303,
-6.92716190461531));
#131566=CARTESIAN_POINT('Ctrl Pts',(-22.0755281745437,2.2584439024064,-6.92470874863353));
#131567=CARTESIAN_POINT('Ctrl Pts',(-22.0972688222191,2.25608524384247,
-6.92328314082742));
#131568=CARTESIAN_POINT('Ctrl Pts',(-22.1463492637306,2.24946883899091,
-6.92000974581403));
#131569=CARTESIAN_POINT('Ctrl Pts',(-22.173632670081,2.24487496516116,-6.91815116196387));
#131570=CARTESIAN_POINT('Ctrl Pts',(-22.2773521442516,2.2238914110896,-6.91098259487542));
#131571=CARTESIAN_POINT('Ctrl Pts',(-22.3523660892459,2.20132108028442,
-6.90559432166925));
#131572=CARTESIAN_POINT('Ctrl Pts',(-22.4686372203978,2.15421454737421,
-6.89717917424165));
#131573=CARTESIAN_POINT('Ctrl Pts',(-22.5114319616763,2.13401533467892,
-6.8940636963432));
#131574=CARTESIAN_POINT('Ctrl Pts',(-22.5781027331393,2.09784467635113,
-6.88918715892521));
#131575=CARTESIAN_POINT('Ctrl Pts',(-22.6027394544039,2.0833777666151,-6.88737928185582));
#131576=CARTESIAN_POINT('Ctrl Pts',(-22.653299041708,2.05133723980745,-6.88364899261077));
#131577=CARTESIAN_POINT('Ctrl Pts',(-22.6791019356882,2.03361024813863,
-6.88173352477339));
#131578=CARTESIAN_POINT('Ctrl Pts',(-22.731695534707,1.99452700681577,-6.87778420312835));
#131579=CARTESIAN_POINT('Ctrl Pts',(-22.7583297642959,1.97300313689141,
-6.8757578284127));
#131580=CARTESIAN_POINT('Ctrl Pts',(-22.8371991367377,1.90379009647875,
-6.86961604351262));
#131581=CARTESIAN_POINT('Ctrl Pts',(-22.8863334023872,1.8527827984822,-6.86559220198115));
#131582=CARTESIAN_POINT('Ctrl Pts',(-22.958761203722,1.76374337893306,-6.85891593393953));
#131583=CARTESIAN_POINT('Ctrl Pts',(-22.9847661437143,1.7281218705474,-6.85632013207033));
#131584=CARTESIAN_POINT('Ctrl Pts',(-23.0191027862774,1.67552268706351,
-6.85248385660168));
#131585=CARTESIAN_POINT('Ctrl Pts',(-23.0289984739246,1.6596012973375,-6.85132214409339));
#131586=CARTESIAN_POINT('Ctrl Pts',(-23.047568715109,1.62818651079117,-6.84901729150804));
#131587=CARTESIAN_POINT('Ctrl Pts',(-23.0562778972977,1.61271892664599,
-6.84787628508707));
#131588=CARTESIAN_POINT('Ctrl Pts',(-23.0839597678304,1.561040592998,-6.84405602115891));
#131589=CARTESIAN_POINT('Ctrl Pts',(-23.1015013533035,1.52409480796297,
-6.84131278764619));
#131590=CARTESIAN_POINT('Ctrl Pts',(-23.1516090040283,1.40384280193087,
-6.83247424524913));
#131591=CARTESIAN_POINT('Ctrl Pts',(-23.1771511290149,1.31789320089251,
-6.82631061008411));
#131592=CARTESIAN_POINT('Ctrl Pts',(-23.2006185206185,1.19100624080797,
-6.81774663659851));
#131593=CARTESIAN_POINT('Ctrl Pts',(-23.205989483707,1.15172673628016,-6.815162729159));
#131594=CARTESIAN_POINT('Ctrl Pts',(-23.2120118205817,1.08415662469309,
-6.81083069183341));
#131595=CARTESIAN_POINT('Ctrl Pts',(-23.213575354763,1.05597936850348,-6.80905719159886));
#131596=CARTESIAN_POINT('Ctrl Pts',(-23.2149448324097,0.993639117870933,
-6.80519683104589));
#131597=CARTESIAN_POINT('Ctrl Pts',(-23.2143120658532,0.959488398291515,
-6.80312419793399));
#131598=CARTESIAN_POINT('Ctrl Pts',(-23.2099565405224,0.885786321757234,
-6.79871234301716));
#131599=CARTESIAN_POINT('Ctrl Pts',(-23.2057515482306,0.846300300933489,
-6.79638717457841));
#131600=CARTESIAN_POINT('Ctrl Pts',(-23.1875791932575,0.728586207702584,
-6.78947305718707));
#131601=CARTESIAN_POINT('Ctrl Pts',(-23.1680956432057,0.651418263043526,
-6.78497187775141));
#131602=CARTESIAN_POINT('Ctrl Pts',(-23.1317280843806,0.549076780320772,
-6.77852669285569));
#131603=CARTESIAN_POINT('Ctrl Pts',(-23.1210008074229,0.521910198356554,
-6.77676599840483));
#131604=CARTESIAN_POINT('Ctrl Pts',(-23.1027317456309,0.479957607221917,
-6.77393297667239));
#131605=CARTESIAN_POINT('Ctrl Pts',(-23.095823007777,0.46490732177892,-6.77289241106506));
#131606=CARTESIAN_POINT('Ctrl Pts',(-23.0792448076277,0.430587102456728,
-6.77045732701787));
#131607=CARTESIAN_POINT('Ctrl Pts',(-23.0693755259031,0.411422743933523,
-6.76905319870975));
#131608=CARTESIAN_POINT('Ctrl Pts',(-23.0460177062739,0.368780362396985,
-6.76584219280443));
#131609=CARTESIAN_POINT('Ctrl Pts',(-23.0322550202698,0.345464320222795,
-6.76402508239477));
#131610=CARTESIAN_POINT('Ctrl Pts',(-22.9782548353948,0.260345066971941,
-6.75720138707321));
#131611=CARTESIAN_POINT('Ctrl Pts',(-22.933381040543,0.201651760054102,
-6.75211978654992));
#131612=CARTESIAN_POINT('Ctrl Pts',(-22.8493305018051,0.109632506664279,
-6.74372836557732));
#131613=CARTESIAN_POINT('Ctrl Pts',(-22.8127730552537,0.0741634603516683,
-6.74036233026094));
#131614=CARTESIAN_POINT('Ctrl Pts',(-22.752050691716,0.0219786042143744,
-6.73520341851663));
#131615=CARTESIAN_POINT('Ctrl Pts',(-22.7292755071091,0.00373644957244235,
-6.73335327419755));
#131616=CARTESIAN_POINT('Ctrl Pts',(-22.6812361681583,-0.0320850622434765,
-6.72961257636881));
#131617=CARTESIAN_POINT('Ctrl Pts',(-22.6559204924024,-0.0495629563493249,
-6.72772656001868));
#131618=CARTESIAN_POINT('Ctrl Pts',(-22.563394516946,-0.108578753591728,
-6.72109846518524));
#131619=CARTESIAN_POINT('Ctrl Pts',(-22.4929628250474,-0.144723789772137,
-6.71654371157681));
#131620=CARTESIAN_POINT('Ctrl Pts',(-22.3556704954303,-0.199639352037324,
-6.70801727982755));
#131621=CARTESIAN_POINT('Ctrl Pts',(-22.2897513395334,-0.219946807210785,
-6.70405517398232));
#131622=CARTESIAN_POINT('Ctrl Pts',(-22.2029902270708,-0.239094826950152,
-6.69865610670695));
#131623=CARTESIAN_POINT('Ctrl Pts',(-22.1833672854766,-0.242939921594036,
-6.69742282018039));
#131624=CARTESIAN_POINT('Ctrl Pts',(-22.1468711343587,-0.249196646176375,
-6.69509316990416));
#131625=CARTESIAN_POINT('Ctrl Pts',(-22.1300250867619,-0.251735335066461,
-6.69400290215746));
#131626=CARTESIAN_POINT('Ctrl Pts',(-22.0795657633504,-0.258300002317591,
-6.6907008151968));
#131627=CARTESIAN_POINT('Ctrl Pts',(-22.0458378928057,-0.261317130978158,
-6.68844668766188));
#131628=CARTESIAN_POINT('Ctrl Pts',(-21.9541252805914,-0.265821702660416,
-6.68225436445445));
#131629=CARTESIAN_POINT('Ctrl Pts',(-21.8960917603556,-0.264679954291367,
-6.67827112571661));
#131630=CARTESIAN_POINT('Ctrl Pts',(-21.7724231956618,-0.253716939435655,
-6.66982434090838));
#131631=CARTESIAN_POINT('Ctrl Pts',(-21.7070577889929,-0.242707042140617,
-6.66538777908186));
#131632=CARTESIAN_POINT('Ctrl Pts',(-21.6133489506423,-0.219241992523442,
-6.65912460472257));
#131633=CARTESIAN_POINT('Ctrl Pts',(-21.584124641201,-0.210793306324488,
-6.65718428603359));
#131634=CARTESIAN_POINT('Ctrl Pts',(-21.5398478262548,-0.196243134294687,
-6.65425946735996));
#131635=CARTESIAN_POINT('Ctrl Pts',(-21.5245635260665,-0.190893027184671,
-6.65325253478706));
#131636=CARTESIAN_POINT('Ctrl Pts',(-21.5093868170662,-0.185251135625031,
-6.6522544014516));
#131637=CARTESIAN_POINT('Origin',(-21.9500000210213,0.999999999999992,-6.00000000000001));
#131638=CARTESIAN_POINT('',(-21.50938681096,-0.185251133355075,-6.15441066307283));
#131639=CARTESIAN_POINT('',(-21.5093309141335,-0.185465194475762,-6.28967656064001));
#131640=CARTESIAN_POINT('',(-21.5093868137063,-0.185251134376008,-6.00000000000001));
#131641=CARTESIAN_POINT('',(-20.9918838682989,1.82521129893649,-6.00000000000001));
#131642=CARTESIAN_POINT('Ctrl Pts',(-21.5093868082137,-0.185251132334142,
-6.15441066307283));
#131643=CARTESIAN_POINT('Ctrl Pts',(-21.5035873446221,-0.183095200805407,
-6.15401289301834));
#131644=CARTESIAN_POINT('Ctrl Pts',(-21.4978038646796,-0.180896763802468,
-6.15361283867239));
#131645=CARTESIAN_POINT('Ctrl Pts',(-21.4625878473075,-0.167213685525018,
-6.1511571735926));
#131646=CARTESIAN_POINT('Ctrl Pts',(-21.4335804894447,-0.154672656841437,
-6.14905029026393));
#131647=CARTESIAN_POINT('Ctrl Pts',(-21.3135856849169,-0.0973679694903984,
-6.14005981956633));
#131648=CARTESIAN_POINT('Ctrl Pts',(-21.2276787361607,-0.0428303393803642,
-6.13297641724258));
#131649=CARTESIAN_POINT('Ctrl Pts',(-21.1170948879019,0.0476606281421388,
-6.12342269196022));
#131650=CARTESIAN_POINT('Ctrl Pts',(-21.0862990852199,0.0754987566832099,
-6.12069966452596));
#131651=CARTESIAN_POINT('Ctrl Pts',(-21.0375321827043,0.124150089584365,
-6.11627985310815));
#131652=CARTESIAN_POINT('Ctrl Pts',(-21.0187722033716,0.144122929985144,
-6.11454962951449));
#131653=CARTESIAN_POINT('Ctrl Pts',(-20.9803961525467,0.187737147608704,
-6.11093663654197));
#131654=CARTESIAN_POINT('Ctrl Pts',(-20.9609625200354,0.211515593731937,
-6.10906192121341));
#131655=CARTESIAN_POINT('Ctrl Pts',(-20.9218656015674,0.263076472741846,
-6.10517087687439));
#131656=CARTESIAN_POINT('Ctrl Pts',(-20.9024193756609,0.290992460109405,
-6.10316275680569));
#131657=CARTESIAN_POINT('Ctrl Pts',(-20.8449421166225,0.381041246971425,
-6.096924715088));
#131658=CARTESIAN_POINT('Ctrl Pts',(-20.8111395642315,0.445690125375156,
-6.09279366128499));
#131659=CARTESIAN_POINT('Ctrl Pts',(-20.7677397050999,0.54965743979662,
-6.08622680730066));
#131660=CARTESIAN_POINT('Ctrl Pts',(-20.7541383691964,0.587129276127882,
-6.08387207511793));
#131661=CARTESIAN_POINT('Ctrl Pts',(-20.7369502708294,0.642508900598489,
-6.0803260379934));
#131662=CARTESIAN_POINT('Ctrl Pts',(-20.7319450187071,0.659953651000476,
-6.07919968154447));
#131663=CARTESIAN_POINT('Ctrl Pts',(-20.7228072521544,0.694597240670247,
-6.07693335908763));
#131664=CARTESIAN_POINT('Ctrl Pts',(-20.7186567867926,0.711787064855045,
-6.07579489678123));
#131665=CARTESIAN_POINT('Ctrl Pts',(-20.7066535968606,0.766505310633434,
-6.07213793571435));
#131666=CARTESIAN_POINT('Ctrl Pts',(-20.7001468746471,0.804304586881464,
-6.06956333806152));
#131667=CARTESIAN_POINT('Ctrl Pts',(-20.6863695904695,0.913940108943603,
-6.06204794116306));
#131668=CARTESIAN_POINT('Ctrl Pts',(-20.6835176458326,0.986181954357668,
-6.05704484144758));
#131669=CARTESIAN_POINT('Ctrl Pts',(-20.689564655222,1.11725835173862,-6.04811588698487));
#131670=CARTESIAN_POINT('Ctrl Pts',(-20.6964141887923,1.17598545012247,
-6.04416858128833));
#131671=CARTESIAN_POINT('Ctrl Pts',(-20.7133990662909,1.26617387807076,
-6.03820556845549));
#131672=CARTESIAN_POINT('Ctrl Pts',(-20.7206992041205,1.29807757740358,
-6.03611489726459));
#131673=CARTESIAN_POINT('Ctrl Pts',(-20.7379454617443,1.36194169394248,
-6.03195570550728));
#131674=CARTESIAN_POINT('Ctrl Pts',(-20.7479389441103,1.39386226237218,
-6.02989035189926));
#131675=CARTESIAN_POINT('Ctrl Pts',(-20.7827238309017,1.49124604286103,
-6.02359352174865));
#131676=CARTESIAN_POINT('Ctrl Pts',(-20.8116905231942,1.55507554217424,
-6.01947811639436));
#131677=CARTESIAN_POINT('Ctrl Pts',(-20.875497414123,1.66941819395525,-6.01177893977397));
#131678=CARTESIAN_POINT('Ctrl Pts',(-20.9090124892552,1.72043080180369,
-6.00820246191594));
#131679=CARTESIAN_POINT('Ctrl Pts',(-20.9541735789873,1.77940199641434,
-6.00368204388054));
#131680=CARTESIAN_POINT('Ctrl Pts',(-20.9624409819876,1.78985118619023,
-6.00286500844259));
#131681=CARTESIAN_POINT('Ctrl Pts',(-20.977769861111,1.80860843511925,-6.00136535341716));
#131682=CARTESIAN_POINT('Ctrl Pts',(-20.9847702393647,1.81695198063206,
-6.00068598746145));
#131683=CARTESIAN_POINT('Ctrl Pts',(-20.991883868299,1.82521129893659,-6.00000000000002));
#131684=CARTESIAN_POINT('',(-22.9011121207488,1.83390790479519,-6.00000965906464));
#131685=CARTESIAN_POINT('Origin',(-21.9500000210213,0.999999999999992,-6.00000000000001));
#131686=CARTESIAN_POINT('Ctrl Pts',(-22.9011121207488,1.83390790479519,
-6.00000965906464));
#131687=CARTESIAN_POINT('Ctrl Pts',(-22.8713097432318,1.86779472815481,
-6.00298048945063));
#131688=CARTESIAN_POINT('Ctrl Pts',(-22.8396158236806,1.90012348438907,
-6.0060066212151));
#131689=CARTESIAN_POINT('Ctrl Pts',(-22.8062336014144,1.9306940554392,-6.00903832068673));
#131690=CARTESIAN_POINT('Ctrl Pts',(-22.7700412498819,1.96383806979444,
-6.01232522987281));
#131691=CARTESIAN_POINT('Ctrl Pts',(-22.7318639832695,1.99491599973358,
-6.01561829348637));
#131692=CARTESIAN_POINT('Ctrl Pts',(-22.6919801403607,2.02370789545272,
-6.01887250050576));
#131693=CARTESIAN_POINT('Ctrl Pts',(-22.652129889946,2.0524755409614,-6.02212396664258));
#131694=CARTESIAN_POINT('Ctrl Pts',(-22.6105760239588,2.07896112137499,
-6.02533647420468));
#131695=CARTESIAN_POINT('Ctrl Pts',(-22.5676151790485,2.1029762674912,-6.02848756994525));
#131696=CARTESIAN_POINT('Ctrl Pts',(-22.5246715436695,2.12698179346589,
-6.03163740339963));
#131697=CARTESIAN_POINT('Ctrl Pts',(-22.4803220859832,2.14851881515413,
-6.03472586264234));
#131698=CARTESIAN_POINT('Ctrl Pts',(-22.4348812613488,2.1674297043965,-6.03775425916792));
#131699=CARTESIAN_POINT('Ctrl Pts',(-22.3894084180212,2.18635391870427,
-6.04078478957421));
#131700=CARTESIAN_POINT('Ctrl Pts',(-22.3428426744419,2.20264809614928,
-6.04375529690198));
#131701=CARTESIAN_POINT('Ctrl Pts',(-22.295517118546,2.2161867333396,-6.04669004057557));
#131702=CARTESIAN_POINT('Ctrl Pts',(-22.2481745126847,2.2297302480911,-6.04962584154846));
#131703=CARTESIAN_POINT('Ctrl Pts',(-22.2000715613054,2.24051587094073,
-6.05252614961448));
#131704=CARTESIAN_POINT('Ctrl Pts',(-22.1515595825469,2.2484546579708,-6.05543509360173));
#131705=CARTESIAN_POINT('Ctrl Pts',(-22.1029631731448,2.25640726173059,
-6.05834910033883));
#131706=CARTESIAN_POINT('Ctrl Pts',(-22.0539564189202,2.26150252955795,
-6.06127230168759));
#131707=CARTESIAN_POINT('Ctrl Pts',(-22.0049096303005,2.26369496890294,
-6.06426284414001));
#131708=CARTESIAN_POINT('Ctrl Pts',(-21.9743762858115,2.2650598392171,-6.06612456160365));
#131709=CARTESIAN_POINT('Ctrl Pts',(-21.943827780378,2.26530060705494,-6.06801264038704));
#131710=CARTESIAN_POINT('Ctrl Pts',(-21.9133562609771,2.2644166063358,-6.06994211780836));
#131711=CARTESIAN_POINT('Ctrl Pts',(-21.9133398817407,2.26441613116235,
-6.0699431549528));
#131712=CARTESIAN_POINT('Ctrl Pts',(-21.9133235025263,2.26441565566411,
-6.0699441921092));
#131713=CARTESIAN_POINT('Ctrl Pts',(-21.9133071233339,2.26441517984107,
-6.06994522927756));
#131714=CARTESIAN_POINT('Ctrl Pts',(-21.8673192256092,2.26307921034984,
-6.07285728937845));
#131715=CARTESIAN_POINT('Ctrl Pts',(-21.821332023664,2.25917004659305,-6.07587137180823));
#131716=CARTESIAN_POINT('Ctrl Pts',(-21.775644760231,2.25272564667812,-6.07892845683477));
#131717=CARTESIAN_POINT('Ctrl Pts',(-21.7708420212566,2.25204819812217,
-6.07924982389206));
#131718=CARTESIAN_POINT('Ctrl Pts',(-21.7660426336406,2.25134276349747,
-6.07957166615584));
#131719=CARTESIAN_POINT('Ctrl Pts',(-21.7612469702657,2.25060940867523,
-6.07989391506484));
#131720=CARTESIAN_POINT('Ctrl Pts',(-21.7121703029202,2.24310458445299,
-6.08319166581872));
#131721=CARTESIAN_POINT('Ctrl Pts',(-21.6634787674,2.23267271882655,-6.08653145174611));
#131722=CARTESIAN_POINT('Ctrl Pts',(-21.6155281574828,2.21940450502726,
-6.08985485980112));
#131723=CARTESIAN_POINT('Ctrl Pts',(-21.5676209205818,2.20614829279485,
-6.09317526171645));
#131724=CARTESIAN_POINT('Ctrl Pts',(-21.5204531188573,2.19006113845352,
-6.09647902274909));
#131725=CARTESIAN_POINT('Ctrl Pts',(-21.474362858205,2.17126760454069,-6.09972932563849));
#131726=CARTESIAN_POINT('Ctrl Pts',(-21.4282952280532,2.15248329832741,
-6.10297803261629));
#131727=CARTESIAN_POINT('Ctrl Pts',(-21.3833040326441,2.13099533602493,
-6.10617323986711));
#131728=CARTESIAN_POINT('Ctrl Pts',(-21.3397116969543,2.10695972318957,
-6.10930243364974));
#131729=CARTESIAN_POINT('Ctrl Pts',(-21.2939491415504,2.08172751099815,
-6.1125874125705));
#131730=CARTESIAN_POINT('Ctrl Pts',(-21.2497284240167,2.05368728589693,
-6.11579947564642));
#131731=CARTESIAN_POINT('Ctrl Pts',(-21.2074043428962,2.02305714661068,
-6.1189532360732));
#131732=CARTESIAN_POINT('Ctrl Pts',(-21.1670505414467,1.99385290811563,
-6.12196018197049));
#131733=CARTESIAN_POINT('Ctrl Pts',(-21.1284209722979,1.96229436247761,
-6.12491454104969));
#131734=CARTESIAN_POINT('Ctrl Pts',(-21.0918052506033,1.92860514658044,
-6.12785217121838));
#131735=CARTESIAN_POINT('Ctrl Pts',(-21.0551669780058,1.89489518215779,
-6.1307916106157));
#131736=CARTESIAN_POINT('Ctrl Pts',(-21.0205454296841,1.85905165078437,
-6.13371471784211));
#131737=CARTESIAN_POINT('Ctrl Pts',(-20.9882088085043,1.82133591135897,
-6.13667539457963));
#131738=CARTESIAN_POINT('Ctrl Pts',(-20.9584022011698,1.78657104742548,
-6.13940442828013));
#131739=CARTESIAN_POINT('Ctrl Pts',(-20.9305368223933,1.75021498090851,
-6.14216597327682));
#131740=CARTESIAN_POINT('Ctrl Pts',(-20.9048013374323,1.71250560459693,
-6.14500982309761));
#131741=CARTESIAN_POINT('Ctrl Pts',(-20.9025707094642,1.70923713735855,
-6.14525631431225));
#131742=CARTESIAN_POINT('Ctrl Pts',(-20.9003560520861,1.70595849200513,
-6.14550342384911));
#131743=CARTESIAN_POINT('Ctrl Pts',(-20.898157470971,1.70266981655717,-6.14575118413152));
#131744=CARTESIAN_POINT('Ctrl Pts',(-20.8942178967889,1.69677693373415,
-6.1461951386462));
#131745=CARTESIAN_POINT('Ctrl Pts',(-20.8903299935753,1.6908519627177,-6.14664118749188));
#131746=CARTESIAN_POINT('Ctrl Pts',(-20.8864943949038,1.68489586492067,
-6.14708951858961));
#131747=CARTESIAN_POINT('Ctrl Pts',(-20.8864852551754,1.68488167232105,
-6.14709058690379));
#131748=CARTESIAN_POINT('Ctrl Pts',(-20.8864761157439,1.68486747954469,
-6.14709165523094));
#131749=CARTESIAN_POINT('Ctrl Pts',(-20.8864669766095,1.6848532865916,-6.14709272357104));
#131750=CARTESIAN_POINT('Ctrl Pts',(-20.8616393916057,1.64629638052638,
-6.14999500111978));
#131751=CARTESIAN_POINT('Ctrl Pts',(-20.8389189581031,1.60628971347035,
-6.15300031840583));
#131752=CARTESIAN_POINT('Ctrl Pts',(-20.8184436372102,1.56509934702104,
-6.15604948295174));
#131753=CARTESIAN_POINT('Ctrl Pts',(-20.8162248249759,1.5606357447414,-6.1563799062762));
#131754=CARTESIAN_POINT('Ctrl Pts',(-20.8140323731525,1.5561582925127,-6.15671084449976));
#131755=CARTESIAN_POINT('Ctrl Pts',(-20.8118664533325,1.55166736533703,
-6.15704222229796));
#131756=CARTESIAN_POINT('Ctrl Pts',(-20.790352298961,1.50705883475574,-6.16033380910543));
#131757=CARTESIAN_POINT('Ctrl Pts',(-20.7714556833859,1.46111498316825,
-6.16366822070424));
#131758=CARTESIAN_POINT('Ctrl Pts',(-20.7553034137482,1.41417869184914,
-6.16698669931937));
#131759=CARTESIAN_POINT('Ctrl Pts',(-20.7391664062568,1.36728675024439,
-6.17030204233144));
#131760=CARTESIAN_POINT('Ctrl Pts',(-20.7257682505138,1.31940427839298,
-6.17360119049667));
#131761=CARTESIAN_POINT('Ctrl Pts',(-20.715197855059,1.27087886425945,-6.17684696009321));
#131762=CARTESIAN_POINT('Ctrl Pts',(-20.7046330109948,1.2223789348416,-6.18009102506719));
#131763=CARTESIAN_POINT('Ctrl Pts',(-20.6968928772115,1.17323674002102,
-6.1832816730545));
#131764=CARTESIAN_POINT('Ctrl Pts',(-20.6920315695949,1.12380481144512,
-6.18640599515564));
#131765=CARTESIAN_POINT('Ctrl Pts',(-20.6871707749018,1.074378098503,-6.18952998760507));
#131766=CARTESIAN_POINT('Ctrl Pts',(-20.6851882933946,1.02466173578174,
-6.19258771833382));
#131767=CARTESIAN_POINT('Ctrl Pts',(-20.6861034240943,0.975013474372067,
-6.19559081097353));
#131768=CARTESIAN_POINT('Ctrl Pts',(-20.6870194252162,0.925317990247499,
-6.19859675999096));
#131769=CARTESIAN_POINT('Ctrl Pts',(-20.6908388122172,0.875690802066594,
-6.20154816281778));
#131770=CARTESIAN_POINT('Ctrl Pts',(-20.6975434174409,0.826495392766933,
-6.20447944209982));
#131771=CARTESIAN_POINT('Ctrl Pts',(-20.7042519357294,0.77727127114003,
-6.20741243218885));
#131772=CARTESIAN_POINT('Ctrl Pts',(-20.7138494721898,0.728479597982973,
-6.2103256739219));
#131773=CARTESIAN_POINT('Ctrl Pts',(-20.7262751195905,0.680487566651962,
-6.21327203433781));
#131774=CARTESIAN_POINT('Ctrl Pts',(-20.7378129540606,0.63592456759643,
-6.21600787720151));
#131775=CARTESIAN_POINT('Ctrl Pts',(-20.7517895524973,0.592050682334131,
-6.21877285310299));
#131776=CARTESIAN_POINT('Ctrl Pts',(-20.768116273302,0.549161052075565,
-6.22161762458379));
#131777=CARTESIAN_POINT('Ctrl Pts',(-20.7694019968649,0.545783508667803,
-6.22184164934464));
#131778=CARTESIAN_POINT('Ctrl Pts',(-20.7707022884922,0.542412043045365,
-6.22206616895837));
#131779=CARTESIAN_POINT('Ctrl Pts',(-20.7720171020505,0.539046785865255,
-6.22229120816688));
#131780=CARTESIAN_POINT('Ctrl Pts',(-20.7758037854877,0.529354792999785,
-6.22293932457718));
#131781=CARTESIAN_POINT('Ctrl Pts',(-20.7797107818593,0.519714530025211,
-6.22359176515896));
#131782=CARTESIAN_POINT('Ctrl Pts',(-20.7837367273305,0.510129376493374,
-6.22424912979539));
#131783=CARTESIAN_POINT('Ctrl Pts',(-20.7837433509997,0.510113606561484,
-6.22425021132168));
#131784=CARTESIAN_POINT('Ctrl Pts',(-20.7837499749908,0.510097836778732,
-6.2242512928613));
#131785=CARTESIAN_POINT('Ctrl Pts',(-20.7837565993039,0.510082067145121,
-6.22425237441425));
#131786=CARTESIAN_POINT('Ctrl Pts',(-20.801503389991,0.46783460934574,-6.22714989656084));
#131787=CARTESIAN_POINT('Ctrl Pts',(-20.8216332018884,0.426505299554568,
-6.23015053397542));
#131788=CARTESIAN_POINT('Ctrl Pts',(-20.8440044314121,0.38635801429458,
-6.23319531389269));
#131789=CARTESIAN_POINT('Ctrl Pts',(-20.8457968689767,0.383141315715649,
-6.23343926909836));
#131790=CARTESIAN_POINT('Ctrl Pts',(-20.8476036714323,0.379932218863172,
-6.23368350768151));
#131791=CARTESIAN_POINT('Ctrl Pts',(-20.849424753186,0.37673086620638,-6.23392799930922));
#131792=CARTESIAN_POINT('Ctrl Pts',(-20.8739400352976,0.333634468494913,
-6.2372193294295));
#131793=CARTESIAN_POINT('Ctrl Pts',(-20.9010476656863,0.291938329336222,
-6.24055591498521));
#131794=CARTESIAN_POINT('Ctrl Pts',(-20.930536340152,0.251942199479993,
-6.24387839074676));
#131795=CARTESIAN_POINT('Ctrl Pts',(-20.9599958277432,0.211985656415745,
-6.24719757803622));
#131796=CARTESIAN_POINT('Ctrl Pts',(-20.9918314361918,0.173725513541029,
-6.2505023823593));
#131797=CARTESIAN_POINT('Ctrl Pts',(-21.0258065615214,0.137432646464108,
-6.25375489189921));
#131798=CARTESIAN_POINT('Ctrl Pts',(-21.0597753040982,0.101146597563584,
-6.2570067904049));
#131799=CARTESIAN_POINT('Ctrl Pts',(-21.095882711719,0.0668270128838862,
-6.26020631217642));
#131800=CARTESIAN_POINT('Ctrl Pts',(-21.133868217647,0.0347190084594118,
-6.26333979107174));
#131801=CARTESIAN_POINT('Ctrl Pts',(-21.1718464646505,0.00261713978520092,
-6.26647267116797));
#131802=CARTESIAN_POINT('Ctrl Pts',(-21.2117021266801,-0.0272739097097115,
-6.26953958018813));
#131803=CARTESIAN_POINT('Ctrl Pts',(-21.2531507563779,-0.0547348690975048,
-6.2725514642462));
#131804=CARTESIAN_POINT('Ctrl Pts',(-21.2946429409792,-0.0822246849142601,
-6.27556651324171));
#131805=CARTESIAN_POINT('Ctrl Pts',(-21.3377315375078,-0.107279055106542,
-6.27852661330183));
#131806=CARTESIAN_POINT('Ctrl Pts',(-21.3821061237463,-0.129706240497145,
-6.28146565119256));
#131807=CARTESIAN_POINT('Ctrl Pts',(-21.4234870870306,-0.150620430665151,
-6.28420641407863));
#131808=CARTESIAN_POINT('Ctrl Pts',(-21.4659862143645,-0.169249924388195,
-6.2869293430793));
#131809=CARTESIAN_POINT('Ctrl Pts',(-21.5093309141335,-0.185465194475759,
-6.28967656064001));
#131810=CARTESIAN_POINT('Origin',(21.9499999789786,0.999999999999992,-6.00000000000001));
#131811=CARTESIAN_POINT('',(22.3906127228612,-0.185251306655355,-7.65234642888876));
#131812=CARTESIAN_POINT('',(22.3905831448079,-0.185130158742934,-7.79034991681388));
#131813=CARTESIAN_POINT('',(22.3906127231008,-0.185251306566283,-6.00000000000001));
#131814=CARTESIAN_POINT('',(20.6856550625054,0.998431907182509,-7.94368587507956));
#131815=CARTESIAN_POINT('Ctrl Pts',(22.390583144063,-0.185130159018148,
-7.79034991686661));
#131816=CARTESIAN_POINT('Ctrl Pts',(22.3439765723818,-0.202348905991787,
-7.79364863419787));
#131817=CARTESIAN_POINT('Ctrl Pts',(22.2963237313581,-0.216845811350756,
-7.79691786542976));
#131818=CARTESIAN_POINT('Ctrl Pts',(22.2479697582444,-0.228522558252233,
-7.80012784772216));
#131819=CARTESIAN_POINT('Ctrl Pts',(22.1996342522863,-0.240194845617333,
-7.80333660407099));
#131820=CARTESIAN_POINT('Ctrl Pts',(22.1505981513039,-0.249049151948672,
-7.80648610985219));
#131821=CARTESIAN_POINT('Ctrl Pts',(22.1012136067467,-0.255021300792385,
-7.80957128037498));
#131822=CARTESIAN_POINT('Ctrl Pts',(22.0517917907318,-0.260997956930732,
-7.81265877933481));
#131823=CARTESIAN_POINT('Ctrl Pts',(22.0020210234089,-0.264087952829062,
-7.81568193738516));
#131824=CARTESIAN_POINT('Ctrl Pts',(21.9522615474857,-0.264262035242583,
-7.81866001093743));
#131825=CARTESIAN_POINT('Ctrl Pts',(21.9024857611145,-0.264436174717843,
-7.82163906065983));
#131826=CARTESIAN_POINT('Ctrl Pts',(21.852721337544,-0.261692172686859,
-7.82457325276417));
#131827=CARTESIAN_POINT('Ctrl Pts',(21.8033355908035,-0.256039305863788,
-7.82750365227269));
#131828=CARTESIAN_POINT('Ctrl Pts',(21.7538565565994,-0.250375761028484,
-7.83043958717462));
#131829=CARTESIAN_POINT('Ctrl Pts',(21.7047578208058,-0.241791833859899,
-7.83337219559926));
#131830=CARTESIAN_POINT('Ctrl Pts',(21.6564137458961,-0.230341818590182,
-7.83635919443393));
#131831=CARTESIAN_POINT('Ctrl Pts',(21.6120256549547,-0.219828755303278,
-7.83910176787573));
#131832=CARTESIAN_POINT('Ctrl Pts',(21.5682741293063,-0.206899581905377,
-7.84189084857918));
#131833=CARTESIAN_POINT('Ctrl Pts',(21.5254491372987,-0.191636063670674,
-7.84477652606721));
#131834=CARTESIAN_POINT('Ctrl Pts',(21.5254316189557,-0.191629819850547,
-7.84477770650615));
#131835=CARTESIAN_POINT('Ctrl Pts',(21.5254141007671,-0.191623575640044,
-7.84477888696124));
#131836=CARTESIAN_POINT('Ctrl Pts',(21.5253965827328,-0.191617331039193,
-7.84478006743251));
#131837=CARTESIAN_POINT('Ctrl Pts',(21.4825790275111,-0.176354286300112,
-7.84766537366112));
#131838=CARTESIAN_POINT('Ctrl Pts',(21.4405270143201,-0.158695683813985,
-7.85065495522489));
#131839=CARTESIAN_POINT('Ctrl Pts',(21.3995078813328,-0.138764776674,-7.85368973772408));
#131840=CARTESIAN_POINT('Ctrl Pts',(21.3946563001692,-0.136407427636807,
-7.85404867982101));
#131841=CARTESIAN_POINT('Ctrl Pts',(21.3898192004068,-0.134018341350694,
-7.85440825424399));
#131842=CARTESIAN_POINT('Ctrl Pts',(21.3849970490046,-0.131597763031438,
-7.85476836324909));
#131843=CARTESIAN_POINT('Ctrl Pts',(21.3410412664877,-0.109533251718649,
-7.85805089666417));
#131844=CARTESIAN_POINT('Ctrl Pts',(21.298323773979,-0.0848475209218615,
-7.86137731033211));
#131845=CARTESIAN_POINT('Ctrl Pts',(21.2571506329473,-0.0577321201817723,
-7.86468830172209));
#131846=CARTESIAN_POINT('Ctrl Pts',(21.2160152298865,-0.0306415725419846,
-7.86799625836432));
#131847=CARTESIAN_POINT('Ctrl Pts',(21.1764211356863,-0.00112603449223744,
-7.87128852432434));
#131848=CARTESIAN_POINT('Ctrl Pts',(21.1386471893365,0.0305959184157649,
-7.87452705674012));
#131849=CARTESIAN_POINT('Ctrl Pts',(21.1008913766293,0.0623026429823067,
-7.87776403447615));
#131850=CARTESIAN_POINT('Ctrl Pts',(21.0649539086597,0.0962135978617711,
-7.88094722892417));
#131851=CARTESIAN_POINT('Ctrl Pts',(21.0310888726463,0.132085078356058,
-7.88406264585824));
#131852=CARTESIAN_POINT('Ctrl Pts',(20.9972253119952,0.167954996075296,
-7.88717792706622));
#131853=CARTESIAN_POINT('Ctrl Pts',(20.9654340915415,0.205785287335624,
-7.89022547658388));
#131854=CARTESIAN_POINT('Ctrl Pts',(20.9359446440149,0.245307147566483,
-7.89321573672232));
#131855=CARTESIAN_POINT('Ctrl Pts',(20.9064227100348,0.284872546255351,
-7.89620929102037));
#131856=CARTESIAN_POINT('Ctrl Pts',(20.879207857653,0.326133326423576,-7.8991456086336));
#131857=CARTESIAN_POINT('Ctrl Pts',(20.8545031866989,0.36879381969754,-7.9020580457105));
#131858=CARTESIAN_POINT('Ctrl Pts',(20.8297821097013,0.411482643237868,
-7.90497241689815));
#131859=CARTESIAN_POINT('Ctrl Pts',(20.8075749656334,0.455573153364719,
-7.90786324835844));
#131860=CARTESIAN_POINT('Ctrl Pts',(20.7880533274443,0.500741568539848,
-7.91078278219348));
#131861=CARTESIAN_POINT('Ctrl Pts',(20.7697789351712,0.543024154113446,
-7.91351578574777));
#131862=CARTESIAN_POINT('Ctrl Pts',(20.7538579722341,0.586251759290134,
-7.91627449720688));
#131863=CARTESIAN_POINT('Ctrl Pts',(20.740399740493,0.630133950092345,-7.91911105232861));
#131864=CARTESIAN_POINT('Ctrl Pts',(20.739454434309,0.633216235130161,-7.9193102919575));
#131865=CARTESIAN_POINT('Ctrl Pts',(20.7385212621352,0.636301763516945,
-7.91950991564037));
#131866=CARTESIAN_POINT('Ctrl Pts',(20.7376002546373,0.639390441086892,
-7.91970994144433));
#131867=CARTESIAN_POINT('Ctrl Pts',(20.7339326743821,0.651689985765733,
-7.92050647208148));
#131868=CARTESIAN_POINT('Ctrl Pts',(20.7304580418358,0.664039060394589,
-7.92130940854894));
#131869=CARTESIAN_POINT('Ctrl Pts',(20.7271781638064,0.676431015095323,
-7.92211992207834));
#131870=CARTESIAN_POINT('Ctrl Pts',(20.7271743568322,0.676445398511668,
-7.92212086284627));
#131871=CARTESIAN_POINT('Ctrl Pts',(20.7271705501204,0.676459781985813,
-7.92212180362441));
#131872=CARTESIAN_POINT('Ctrl Pts',(20.7271667436709,0.676474165517736,
-7.92212274441275));
#131873=CARTESIAN_POINT('Ctrl Pts',(20.7145136658905,0.724286687274377,
-7.92525003355821));
#131874=CARTESIAN_POINT('Ctrl Pts',(20.7047344388994,0.772850328217294,
-7.92849442468279));
#131875=CARTESIAN_POINT('Ctrl Pts',(20.6978549531996,0.821872855167937,
-7.93179039624007));
#131876=CARTESIAN_POINT('Ctrl Pts',(20.6956260182459,0.837756022690157,
-7.9328582822029));
#131877=CARTESIAN_POINT('Ctrl Pts',(20.6937015692772,0.853686960859425,
-7.93393158278377));
#131878=CARTESIAN_POINT('Ctrl Pts',(20.6920826480587,0.869654568896896,
-7.9350080695044));
#131879=CARTESIAN_POINT('Ctrl Pts',(20.6877513941166,0.912374229662736,
-7.93788809683325));
#131880=CARTESIAN_POINT('Ctrl Pts',(20.6856051097385,0.955362919347453,
-7.94079142940216));
#131881=CARTESIAN_POINT('Ctrl Pts',(20.6856550625054,0.998431907182509,
-7.94368587507956));
#131882=CARTESIAN_POINT('',(20.9918838262563,1.82521129893649,-8.00000000000001));
#131883=CARTESIAN_POINT('Ctrl Pts',(20.6855009578283,0.998426624634692,
-7.943774545494));
#131884=CARTESIAN_POINT('Ctrl Pts',(20.6854347818123,1.05161133140669,-7.94742215375545));
#131885=CARTESIAN_POINT('Ctrl Pts',(20.6887240589389,1.1047510902817,-7.95103786349476));
#131886=CARTESIAN_POINT('Ctrl Pts',(20.6953507587871,1.15752962982536,-7.95457609541917));
#131887=CARTESIAN_POINT('Ctrl Pts',(20.6993094976487,1.18905911815829,-7.95668980760494));
#131888=CARTESIAN_POINT('Ctrl Pts',(20.7044555563998,1.2204299808716,-7.95877460230176));
#131889=CARTESIAN_POINT('Ctrl Pts',(20.7107784821558,1.25157569797626,-7.96082752239111));
#131890=CARTESIAN_POINT('Ctrl Pts',(20.7169430191148,1.28194121729719,-7.96282901699239));
#131891=CARTESIAN_POINT('Ctrl Pts',(20.7242219132126,1.31207161227981,-7.96479884775945));
#131892=CARTESIAN_POINT('Ctrl Pts',(20.7326009343683,1.34190615113201,-7.96673892557842));
#131893=CARTESIAN_POINT('Ctrl Pts',(20.7418217164266,1.3747378835567,-7.9688739046425));
#131894=CARTESIAN_POINT('Ctrl Pts',(20.7523673405614,1.4071848917607,-7.970971063412));
#131895=CARTESIAN_POINT('Ctrl Pts',(20.7642125622979,1.43916790916664,-7.97303914742824));
#131896=CARTESIAN_POINT('Ctrl Pts',(20.777679644269,1.47553007499761,-7.97539039568592));
#131897=CARTESIAN_POINT('Ctrl Pts',(20.7928126393162,1.51125486619278,-7.97770151418053));
#131898=CARTESIAN_POINT('Ctrl Pts',(20.8095641954328,1.54622932327752,-7.97999472541712));
#131899=CARTESIAN_POINT('Ctrl Pts',(20.8480280883029,1.6265355205727,-7.98526025601735));
#131900=CARTESIAN_POINT('Ctrl Pts',(20.8948635669814,1.70254792840251,-7.99039904379838));
#131901=CARTESIAN_POINT('Ctrl Pts',(20.9492881987892,1.77300464616334,-7.99582841388747));
#131902=CARTESIAN_POINT('Ctrl Pts',(20.9630213219082,1.79078319141818,-7.99719842238208));
#131903=CARTESIAN_POINT('Ctrl Pts',(20.977224964316,1.80819154602769,-7.99858640426953));
#131904=CARTESIAN_POINT('Ctrl Pts',(20.9918838262562,1.82521129893648,-8.00000000000004));
#131905=CARTESIAN_POINT('',(22.898512696641,1.83623195013869,-8.00000000000001));
#131906=CARTESIAN_POINT('Origin',(21.9499999789786,0.999999999999992,-8.00000000000001));
#131907=CARTESIAN_POINT('Ctrl Pts',(22.8985126966416,1.83623195013798,-8.00000000000009));
#131908=CARTESIAN_POINT('Ctrl Pts',(22.8436297891941,1.89848397924026,-7.99445558980496));
#131909=CARTESIAN_POINT('Ctrl Pts',(22.7827601951912,1.95517447097983,-7.98871488534317));
#131910=CARTESIAN_POINT('Ctrl Pts',(22.671656060386,2.03989960638361,-7.97926197537341));
#131911=CARTESIAN_POINT('Ctrl Pts',(22.624276631408,2.07122875529249,-7.97548954756314));
#131912=CARTESIAN_POINT('Ctrl Pts',(22.5489424976922,2.11405698150326,-7.96989091770804));
#131913=CARTESIAN_POINT('Ctrl Pts',(22.5224192930673,2.1279146503469,-7.9679887303622));
#131914=CARTESIAN_POINT('Ctrl Pts',(22.4678037755625,2.15402642253875,-7.96420091867253));
#131915=CARTESIAN_POINT('Ctrl Pts',(22.4397078143008,2.16622648734987,-7.96231802136835));
#131916=CARTESIAN_POINT('Ctrl Pts',(22.3483030827951,2.20203042654509,-7.95637196138385));
#131917=CARTESIAN_POINT('Ctrl Pts',(22.2835361641471,2.22158803589501,-7.95243349309627));
#131918=CARTESIAN_POINT('Ctrl Pts',(22.1634086356694,2.24759019110203,-7.94531500915695));
#131919=CARTESIAN_POINT('Ctrl Pts',(22.1085972633573,2.25573521532646,-7.94213191053803));
#131920=CARTESIAN_POINT('Ctrl Pts',(22.0204967723728,2.2629657330336,-7.93690735040823));
#131921=CARTESIAN_POINT('Ctrl Pts',(21.9874714986606,2.26437643676886,-7.93492418251912));
#131922=CARTESIAN_POINT('Ctrl Pts',(21.9372952307496,2.26455229355907,-7.9318250472819));
#131923=CARTESIAN_POINT('Ctrl Pts',(21.9201600093796,2.26426400218925,-7.93075116236837));
#131924=CARTESIAN_POINT('Ctrl Pts',(21.8821002210124,2.26284946843498,-7.92832303891685));
#131925=CARTESIAN_POINT('Ctrl Pts',(21.8611885250819,2.26155125263614,-7.92696163658804));
#131926=CARTESIAN_POINT('Ctrl Pts',(21.7418236175042,2.25115865318114,-7.9190684694165));
#131927=CARTESIAN_POINT('Ctrl Pts',(21.6446749578416,2.23106139711964,-7.9121985977141));
#131928=CARTESIAN_POINT('Ctrl Pts',(21.5004156162989,2.18307241377343,-7.9019463906592));
#131929=CARTESIAN_POINT('Ctrl Pts',(21.451075543509,2.16312595231789,-7.89842329015815));
#131930=CARTESIAN_POINT('Ctrl Pts',(21.3765731557395,2.12739063021314,-7.89309421447382));
#131931=CARTESIAN_POINT('Ctrl Pts',(21.3504652919219,2.11372632868274,-7.89122413009542));
#131932=CARTESIAN_POINT('Ctrl Pts',(21.2982131874887,2.08400818107004,-7.88746856761019));
#131933=CARTESIAN_POINT('Ctrl Pts',(21.2721279179092,2.06789018985442,-7.88558682154398));
#131934=CARTESIAN_POINT('Ctrl Pts',(21.1887889082,2.01210973217063,-7.87952405427109));
#131935=CARTESIAN_POINT('Ctrl Pts',(21.1342206196968,1.9686659641545,-7.87547928913312));
#131936=CARTESIAN_POINT('Ctrl Pts',(21.029555947919,1.87018938372836,-7.86718547274263));
#131937=CARTESIAN_POINT('Ctrl Pts',(20.9801783651624,1.81479496458115,-7.86295438941036));
#131938=CARTESIAN_POINT('Ctrl Pts',(20.9225130888004,1.73738447022363,-7.85713500106844));
#131939=CARTESIAN_POINT('Ctrl Pts',(20.9095730760053,1.71901104711099,-7.85575932754119));
#131940=CARTESIAN_POINT('Ctrl Pts',(20.888053032726,1.68665681085156,-7.85332857558938));
#131941=CARTESIAN_POINT('Ctrl Pts',(20.8792433408731,1.67283654808712,-7.85228673397135));
#131942=CARTESIAN_POINT('Ctrl Pts',(20.8564682921383,1.63552756321596,-7.84946679521615));
#131943=CARTESIAN_POINT('Ctrl Pts',(20.8429923877664,1.61175223623375,-7.84766400755591));
#131944=CARTESIAN_POINT('Ctrl Pts',(20.7887603372009,1.50840344764925,-7.83985828040673));
#131945=CARTESIAN_POINT('Ctrl Pts',(20.7557334390164,1.4250644966225,-7.83366120327489));
#131946=CARTESIAN_POINT('Ctrl Pts',(20.718106760785,1.28982428891886,-7.82420566388658));
#131947=CARTESIAN_POINT('Ctrl Pts',(20.7074237869657,1.23992593849276,-7.82083232495627));
#131948=CARTESIAN_POINT('Ctrl Pts',(20.6954260977827,1.16077739579424,-7.815673277277));
#131949=CARTESIAN_POINT('Ctrl Pts',(20.6920619229972,1.13189790239961,-7.81382948887018));
#131950=CARTESIAN_POINT('Ctrl Pts',(20.6872141936175,1.07253872181825,-7.81011122168199));
#131951=CARTESIAN_POINT('Ctrl Pts',(20.6858322030414,1.04206980797261,-7.80824092476375));
#131952=CARTESIAN_POINT('Ctrl Pts',(20.6848879644734,0.938954808434391,
-7.80201185032114));
#131953=CARTESIAN_POINT('Ctrl Pts',(20.69048063927,0.866406014374577,-7.79780630718665));
#131954=CARTESIAN_POINT('Ctrl Pts',(20.7137856495591,0.724745150124373,
-7.78953253434507));
#131955=CARTESIAN_POINT('Ctrl Pts',(20.7311666888633,0.655856579929814,
-7.785475299777));
#131956=CARTESIAN_POINT('Ctrl Pts',(20.7614715598617,0.567730836360711,
-7.77985854089706));
#131957=CARTESIAN_POINT('Ctrl Pts',(20.7692700943263,0.546862896536249,
-7.77849508982802));
#131958=CARTESIAN_POINT('Ctrl Pts',(20.7837550108444,0.511019980259353,
-7.77607723801927));
#131959=CARTESIAN_POINT('Ctrl Pts',(20.7901887667071,0.495949766780783,
-7.7750356607319));
#131960=CARTESIAN_POINT('Ctrl Pts',(20.8081789253604,0.455979466985741,
-7.77220841384106));
#131961=CARTESIAN_POINT('Ctrl Pts',(20.8202557382879,0.431324891264073,
-7.77039770220559));
#131962=CARTESIAN_POINT('Ctrl Pts',(20.8707345097507,0.336237906654735,
-7.76319912609828));
#131963=CARTESIAN_POINT('Ctrl Pts',(20.9149998996471,0.269131350926939,
-7.75765584879279));
#131964=CARTESIAN_POINT('Ctrl Pts',(20.9908243496453,0.175018505162643,
-7.7494751762915));
#131965=CARTESIAN_POINT('Ctrl Pts',(21.017838006586,0.144613032116268,-7.74675494863844));
#131966=CARTESIAN_POINT('Ctrl Pts',(21.0705061472736,0.0907962843073573,
-7.74180810659167));
#131967=CARTESIAN_POINT('Ctrl Pts',(21.0957500988475,0.067037892260422,
-7.73956977879915));
#131968=CARTESIAN_POINT('Ctrl Pts',(21.1432732656925,0.0258598407101029,
-7.73558275663927));
#131969=CARTESIAN_POINT('Ctrl Pts',(21.1652205008591,0.00809355188603256,
-7.73382123769572));
#131970=CARTESIAN_POINT('Ctrl Pts',(21.2188884667804,-0.0324532458505455,
-7.7296866137588));
#131971=CARTESIAN_POINT('Ctrl Pts',(21.2511059609009,-0.0545289526710269,
-7.72734010877895));
#131972=CARTESIAN_POINT('Ctrl Pts',(21.3609982179887,-0.122575735708734,
-7.71969304827861));
#131973=CARTESIAN_POINT('Ctrl Pts',(21.44256021831,-0.161724533487817,-7.7145931898283));
#131974=CARTESIAN_POINT('Ctrl Pts',(21.5550025599966,-0.201575194328529,
-7.70762359246858));
#131975=CARTESIAN_POINT('Ctrl Pts',(21.5827377485318,-0.2103405208425,-7.70590705870495));
#131976=CARTESIAN_POINT('Ctrl Pts',(21.6325257859147,-0.224206440471404,
-7.70279233426908));
#131977=CARTESIAN_POINT('Ctrl Pts',(21.6544600491531,-0.229685846040324,
-7.70140885883999));
#131978=CARTESIAN_POINT('Ctrl Pts',(21.6925861538772,-0.238131211479962,
-7.69896668246375));
#131979=CARTESIAN_POINT('Ctrl Pts',(21.7087099162753,-0.2413741514721,-7.69792142887289));
#131980=CARTESIAN_POINT('Ctrl Pts',(21.7518898290421,-0.249185878852511,
-7.69509120283369));
#131981=CARTESIAN_POINT('Ctrl Pts',(21.7790375430942,-0.253189772976175,
-7.69328140865882));
#131982=CARTESIAN_POINT('Ctrl Pts',(21.8859837724665,-0.265423285936066,
-7.68608407919356));
#131983=CARTESIAN_POINT('Ctrl Pts',(21.9663611635882,-0.266935892379982,
-7.68054105196579));
#131984=CARTESIAN_POINT('Ctrl Pts',(22.1035214894421,-0.256455405429357,
-7.67123043782603));
#131985=CARTESIAN_POINT('Ctrl Pts',(22.1603447271469,-0.24820091625219,
-7.6674143525328));
#131986=CARTESIAN_POINT('Ctrl Pts',(22.2454479735416,-0.229858796370244,
-7.66178860471871));
#131987=CARTESIAN_POINT('Ctrl Pts',(22.2742508618983,-0.222580782403874,
-7.65989970020417));
#131988=CARTESIAN_POINT('Ctrl Pts',(22.3316239329181,-0.205912954943925,
-7.65616076192792));
#131989=CARTESIAN_POINT('Ctrl Pts',(22.3601688331301,-0.196505172665629,
-7.65431265162712));
#131990=CARTESIAN_POINT('Ctrl Pts',(22.3891067506122,-0.185810329809031,
-7.6524436839551));
#131991=CARTESIAN_POINT('Ctrl Pts',(22.3898598818392,-0.185531172491713,
-7.65239504564353));
#131992=CARTESIAN_POINT('Ctrl Pts',(22.3906127226216,-0.185251306744424,
-7.65234642888876));
#131993=CARTESIAN_POINT('Origin',(21.9499999789786,0.999999999999992,-6.00000000000001));
#131994=CARTESIAN_POINT('',(22.3906127229457,-0.185251306623939,-7.15421791561113));
#131995=CARTESIAN_POINT('',(22.3906403691454,-0.185356836028299,-7.28986813301021));
#131996=CARTESIAN_POINT('',(22.3906127231008,-0.185251306566283,-6.00000000000001));
#131997=CARTESIAN_POINT('',(20.6854351050354,1.00099360643116,-7.4433066090729));
#131998=CARTESIAN_POINT('Ctrl Pts',(22.3906403684231,-0.185356836298634,
-7.28986813305573));
#131999=CARTESIAN_POINT('Ctrl Pts',(22.3440517461525,-0.202794827868046,
-7.29280460895284));
#132000=CARTESIAN_POINT('Ctrl Pts',(22.2964803100234,-0.217456218389545,
-7.2957499216459));
#132001=CARTESIAN_POINT('Ctrl Pts',(22.2482864098299,-0.229219763841232,
-7.29876435271249));
#132002=CARTESIAN_POINT('Ctrl Pts',(22.217446148307,-0.236747496950825,
-7.30069334874856));
#132003=CARTESIAN_POINT('Ctrl Pts',(22.1863515382631,-0.243089361282193,
-7.30265094181487));
#132004=CARTESIAN_POINT('Ctrl Pts',(22.15510248789,-0.248224054371781,-7.30465409393146));
#132005=CARTESIAN_POINT('Ctrl Pts',(22.1550857866994,-0.248226798630788,
-7.30465516452481));
#132006=CARTESIAN_POINT('Ctrl Pts',(22.1550690854644,-0.248229542545221,
-7.30465623513116));
#132007=CARTESIAN_POINT('Ctrl Pts',(22.1550523841852,-0.248232286115091,
-7.30465730575054));
#132008=CARTESIAN_POINT('Ctrl Pts',(22.109765840256,-0.255671644239026,
-7.30756035590221));
#132009=CARTESIAN_POINT('Ctrl Pts',(22.0639887458557,-0.260596991460554,
-7.31056645868888));
#132010=CARTESIAN_POINT('Ctrl Pts',(22.0180204829633,-0.262988013273262,
-7.31361650791182));
#132011=CARTESIAN_POINT('Ctrl Pts',(22.0130719410616,-0.263245409809123,
-7.31394484958566));
#132012=CARTESIAN_POINT('Ctrl Pts',(22.0081212276411,-0.263473459992872,
-7.3142737005458));
#132013=CARTESIAN_POINT('Ctrl Pts',(22.0031687473583,-0.263672156307481,
-7.31460298705436));
#132014=CARTESIAN_POINT('Ctrl Pts',(21.9536334923752,-0.265659538799975,
-7.31789654709556));
#132015=CARTESIAN_POINT('Ctrl Pts',(21.9039160545772,-0.264708195030253,
-7.32123313004558));
#132016=CARTESIAN_POINT('Ctrl Pts',(21.854382158871,-0.260838706472937,
-7.32455398111115));
#132017=CARTESIAN_POINT('Ctrl Pts',(21.8048944344205,-0.256972824721493,
-7.32787173676373));
#132018=CARTESIAN_POINT('Ctrl Pts',(21.7555898162755,-0.250194536762391,
-7.33117349636671));
#132019=CARTESIAN_POINT('Ctrl Pts',(21.7068231680761,-0.240561070008607,
-7.3344220800825));
#132020=CARTESIAN_POINT('Ctrl Pts',(21.6580816294929,-0.230932563461495,
-7.33766899112458));
#132021=CARTESIAN_POINT('Ctrl Pts',(21.6098774738854,-0.218451892946313,
-7.34086268598225));
#132022=CARTESIAN_POINT('Ctrl Pts',(21.5625561924181,-0.203210155758827,
-7.34399027737459));
#132023=CARTESIAN_POINT('Ctrl Pts',(21.512757336974,-0.187170415426774,
-7.34728161832744));
#132024=CARTESIAN_POINT('Ctrl Pts',(21.463936382959,-0.168072485624941,
-7.35049957206803));
#132025=CARTESIAN_POINT('Ctrl Pts',(21.4164851980655,-0.146063276856775,
-7.35365846723112));
#132026=CARTESIAN_POINT('Ctrl Pts',(21.3713552082722,-0.125130704376378,
-7.35666283702268));
#132027=CARTESIAN_POINT('Ctrl Pts',(21.3274643368433,-0.101564802796739,
-7.35961420736341));
#132028=CARTESIAN_POINT('Ctrl Pts',(21.2851387168268,-0.0755293390491522,
-7.36254816026591));
#132029=CARTESIAN_POINT('Ctrl Pts',(21.2427874543799,-0.0494781020520178,
-7.36548389066589));
#132030=CARTESIAN_POINT('Ctrl Pts',(21.2020036753296,-0.0209539720715463,
-7.3684025954985));
#132031=CARTESIAN_POINT('Ctrl Pts',(21.1630996744432,0.00983828316542695,
-7.37135798185939));
#132032=CARTESIAN_POINT('Ctrl Pts',(21.1271805269864,0.0382680469734418,
-7.37408662045877));
#132033=CARTESIAN_POINT('Ctrl Pts',(21.0928635577385,0.0686317094549675,
-7.37684711524653));
#132034=CARTESIAN_POINT('Ctrl Pts',(21.0603798066664,0.100731383818771,
-7.37968948029064));
#132035=CARTESIAN_POINT('Ctrl Pts',(21.057622289732,0.103456296820673,-7.37993076614847));
#132036=CARTESIAN_POINT('Ctrl Pts',(21.0548779525668,0.106193724953976,
-7.38017264197664));
#132037=CARTESIAN_POINT('Ctrl Pts',(21.0521469194695,0.108943550494673,
-7.38041513836999));
#132038=CARTESIAN_POINT('Ctrl Pts',(21.046885270883,0.114241404879535,-7.38088233549279));
#132039=CARTESIAN_POINT('Ctrl Pts',(21.0416730872256,0.119585160851676,
-7.38135184194807));
#132040=CARTESIAN_POINT('Ctrl Pts',(21.0365113105743,0.124973855152702,
-7.38182387855428));
#132041=CARTESIAN_POINT('Ctrl Pts',(21.0364995820756,0.124986099249765,
-7.38182495110761));
#132042=CARTESIAN_POINT('Ctrl Pts',(21.036487853837,0.124998343578842,-7.381826023674));
#132043=CARTESIAN_POINT('Ctrl Pts',(21.0364761258587,0.125010588139904,
-7.38182709625346));
#132044=CARTESIAN_POINT('Ctrl Pts',(21.0050835186137,0.157785946906783,
-7.38469809966508));
#132045=CARTESIAN_POINT('Ctrl Pts',(20.9754384365615,0.192357167576284,
-7.38767062125446));
#132046=CARTESIAN_POINT('Ctrl Pts',(20.9477272918121,0.228494563598768,
-7.39068712703531));
#132047=CARTESIAN_POINT('Ctrl Pts',(20.9456263670576,0.231234325905718,
-7.39091582389083));
#132048=CARTESIAN_POINT('Ctrl Pts',(20.9435365602325,0.233983065747832,
-7.39114477356475));
#132049=CARTESIAN_POINT('Ctrl Pts',(20.9414579531322,0.236740670872581,
-7.39137395098486));
#132050=CARTESIAN_POINT('Ctrl Pts',(20.9120040321276,0.275816012956855,
-7.39462140146588));
#132051=CARTESIAN_POINT('Ctrl Pts',(20.8847980747372,0.316676796555248,
-7.3979140006635));
#132052=CARTESIAN_POINT('Ctrl Pts',(20.8600293289857,0.359018625118562,
-7.40119405356233));
#132053=CARTESIAN_POINT('Ctrl Pts',(20.8352843205297,0.40131987510317,-7.4044709630002));
#132054=CARTESIAN_POINT('Ctrl Pts',(20.812971582611,0.445099194933415,-7.40773505376474));
#132055=CARTESIAN_POINT('Ctrl Pts',(20.7932434164791,0.490039494436445,
-7.41094889565801));
#132056=CARTESIAN_POINT('Ctrl Pts',(20.7735180069206,0.534973514530128,
-7.41416228848821));
#132057=CARTESIAN_POINT('Ctrl Pts',(20.7563763761227,0.581068128698808,
-7.41732534313056));
#132058=CARTESIAN_POINT('Ctrl Pts',(20.7419368779796,0.627994199072142,
-7.42042367767064));
#132059=CARTESIAN_POINT('Ctrl Pts',(20.7274989405527,0.674915197366821,
-7.42352167732232));
#132060=CARTESIAN_POINT('Ctrl Pts',(20.7157626383642,0.72266742180228,-7.42655501240717));
#132061=CARTESIAN_POINT('Ctrl Pts',(20.7068122566636,0.770910467044918,
-7.42953277296501));
#132062=CARTESIAN_POINT('Ctrl Pts',(20.697852973447,0.819201491944744,-7.43251349502601));
#132063=CARTESIAN_POINT('Ctrl Pts',(20.6916853913536,0.867984253049784,
-7.4354387127125));
#132064=CARTESIAN_POINT('Ctrl Pts',(20.6883575187536,0.916906744626067,
-7.43833941828639));
#132065=CARTESIAN_POINT('Ctrl Pts',(20.686452467469,0.944912580975547,-7.43999993644446));
#132066=CARTESIAN_POINT('Ctrl Pts',(20.6854773133495,0.972964015475198,
-7.44165281629599));
#132067=CARTESIAN_POINT('Ctrl Pts',(20.6854351050355,1.00099360637425,-7.44330660906956));
#132068=CARTESIAN_POINT('Ctrl Pts',(20.6854351050347,1.00099360693951,-7.44330660910288));
#132069=CARTESIAN_POINT('Ctrl Pts',(20.6853606881594,1.05041219279047,-7.44622238837541));
#132070=CARTESIAN_POINT('Ctrl Pts',(20.6881872209223,1.09973540379018,-7.44913841382896));
#132071=CARTESIAN_POINT('Ctrl Pts',(20.6938991273629,1.14865874359727,-7.4521175879256));
#132072=CARTESIAN_POINT('Ctrl Pts',(20.6959601823621,1.16631199039665,-7.45319257781373));
#132073=CARTESIAN_POINT('Ctrl Pts',(20.6983970294421,1.18391365320077,-7.45427578976892));
#132074=CARTESIAN_POINT('Ctrl Pts',(20.7012094620179,1.20145101245753,-7.45537017903375));
#132075=CARTESIAN_POINT('Ctrl Pts',(20.7042769785817,1.22057898745944,-7.45656382798587));
#132076=CARTESIAN_POINT('Ctrl Pts',(20.70779063137,1.23962909537417,-7.45777096884554));
#132077=CARTESIAN_POINT('Ctrl Pts',(20.7117486726152,1.25858259994124,-7.45899574224935));
#132078=CARTESIAN_POINT('Ctrl Pts',(20.7117521352302,1.25859918104416,-7.45899681371842));
#132079=CARTESIAN_POINT('Ctrl Pts',(20.7117555981854,1.25861576207324,-7.45899788520098));
#132080=CARTESIAN_POINT('Ctrl Pts',(20.7117590614805,1.25863234302847,-7.45899895669704));
#132081=CARTESIAN_POINT('Ctrl Pts',(20.7211417365784,1.30355306361916,-7.46190182775864));
#132082=CARTESIAN_POINT('Ctrl Pts',(20.7330459087108,1.34802523649897,-7.46490780513171));
#132083=CARTESIAN_POINT('Ctrl Pts',(20.7473826374716,1.3917623628161,-7.4679578018695));
#132084=CARTESIAN_POINT('Ctrl Pts',(20.7489269335377,1.39647355413732,-7.46828633552891));
#132085=CARTESIAN_POINT('Ctrl Pts',(20.7504994162171,1.4011761843785,-7.46861537993406));
#132086=CARTESIAN_POINT('Ctrl Pts',(20.7520999464277,1.40586987280228,-7.46894486123794));
#132087=CARTESIAN_POINT('Ctrl Pts',(20.768101593778,1.45279603916396,-7.47223892191749));
#132088=CARTESIAN_POINT('Ctrl Pts',(20.7869106309768,1.49883273151624,-7.47557610128714));
#132089=CARTESIAN_POINT('Ctrl Pts',(20.8083759978131,1.54364616741722,-7.47889761510544));
#132090=CARTESIAN_POINT('Ctrl Pts',(20.8298213296407,1.58841777605368,-7.48221602874108));
#132091=CARTESIAN_POINT('Ctrl Pts',(20.8539177874338,1.63196860702536,-7.48551851215197));
#132092=CARTESIAN_POINT('Ctrl Pts',(20.8804840426551,1.67398823042049,-7.48876784757917));
#132093=CARTESIAN_POINT('Ctrl Pts',(20.9070365793477,1.71598615533367,-7.49201550508447));
#132094=CARTESIAN_POINT('Ctrl Pts',(20.9360563049012,1.75645451207017,-7.49520997419177));
#132095=CARTESIAN_POINT('Ctrl Pts',(20.9673336789034,1.79510382822157,-7.49833832604472));
#132096=CARTESIAN_POINT('Ctrl Pts',(21.0002428909582,1.83576959961621,-7.50162989376083));
#132097=CARTESIAN_POINT('Ctrl Pts',(21.0356518211773,1.87442126512674,-7.50484808522027));
#132098=CARTESIAN_POINT('Ctrl Pts',(21.0732822976041,1.91074636611629,-7.50800716965886));
#132099=CARTESIAN_POINT('Ctrl Pts',(21.109078030499,1.94530036956959,-7.5110122270882));
#132100=CARTESIAN_POINT('Ctrl Pts',(21.1468838455241,1.97774910464242,-7.51396422222195));
#132101=CARTESIAN_POINT('Ctrl Pts',(21.1864294111691,2.00784734685896,-7.51689869185879));
#132102=CARTESIAN_POINT('Ctrl Pts',(21.2259988566345,2.03796376407449,-7.51983493349222));
#132103=CARTESIAN_POINT('Ctrl Pts',(21.2673103486457,2.0657264150824,-7.52275404115145));
#132104=CARTESIAN_POINT('Ctrl Pts',(21.3100603053001,2.09091775667308,-7.52570968175975));
#132105=CARTESIAN_POINT('Ctrl Pts',(21.3495366765676,2.11418006688782,-7.52843899367297));
#132106=CARTESIAN_POINT('Ctrl Pts',(21.3902401526173,2.13524982412564,-7.53120004496706));
#132107=CARTESIAN_POINT('Ctrl Pts',(21.4319027378402,2.15398273504556,-7.53404285055596));
#132108=CARTESIAN_POINT('Ctrl Pts',(21.4354320126832,2.15556961667789,-7.53428366715902));
#132109=CARTESIAN_POINT('Ctrl Pts',(21.4389681858387,2.15713975591571,-7.53452507042564));
#132110=CARTESIAN_POINT('Ctrl Pts',(21.4425111035855,2.1586930796388,-7.53476709075887));
#132111=CARTESIAN_POINT('Ctrl Pts',(21.4493265365929,2.16168117434781,-7.53523265995508));
#132112=CARTESIAN_POINT('Ctrl Pts',(21.4561667916288,2.1646070078569,-7.53570051850504));
#132113=CARTESIAN_POINT('Ctrl Pts',(21.4630306434348,2.16747005383963,-7.53617088487625));
#132114=CARTESIAN_POINT('Ctrl Pts',(21.4630461964787,2.1674765413165,-7.536171950696));
#132115=CARTESIAN_POINT('Ctrl Pts',(21.4630617496438,2.16748302847101,-7.53617301652863));
#132116=CARTESIAN_POINT('Ctrl Pts',(21.46307730293,2.16748951530316,-7.53617408237413));
#132117=CARTESIAN_POINT('Ctrl Pts',(21.5054518069055,2.18516271254244,-7.53907794937767));
#132118=CARTESIAN_POINT('Ctrl Pts',(21.5488831083792,2.20050047344378,-7.54208476489056));
#132119=CARTESIAN_POINT('Ctrl Pts',(21.5930842430634,2.21341406344646,-7.54513539763158));
#132120=CARTESIAN_POINT('Ctrl Pts',(21.5978233774849,2.2147986260674,-7.54546247879666));
#132121=CARTESIAN_POINT('Ctrl Pts',(21.6025713138547,2.21615533396418,-7.54579006366657));
#132122=CARTESIAN_POINT('Ctrl Pts',(21.6073276644696,2.21748408778358,-7.54611807936035));
#132123=CARTESIAN_POINT('Ctrl Pts',(21.6550817372542,2.23082486346267,-7.54941137848474));
#132124=CARTESIAN_POINT('Ctrl Pts',(21.7036897457322,2.24134699705942,-7.55274755630456));
#132125=CARTESIAN_POINT('Ctrl Pts',(21.7527909628984,2.24898631868653,-7.55606791454492));
#132126=CARTESIAN_POINT('Ctrl Pts',(21.8018464991694,2.25661853313646,-7.55938518371853));
#132127=CARTESIAN_POINT('Ctrl Pts',(21.8513943492424,2.2613736111464,-7.56268636987707));
#132128=CARTESIAN_POINT('Ctrl Pts',(21.9010759123168,2.26322553102128,-7.56593437146185));
#132129=CARTESIAN_POINT('Ctrl Pts',(21.9507319638335,2.2650764999325,-7.56918070519291));
#132130=CARTESIAN_POINT('Ctrl Pts',(22.000521606279,2.26402737190795,-7.57237381442538));
#132131=CARTESIAN_POINT('Ctrl Pts',(22.050087550098,2.26008723736913,-7.57550090374385));
#132132=CARTESIAN_POINT('Ctrl Pts',(22.1022357163895,2.25594183479411,-7.57879090411957));
#132133=CARTESIAN_POINT('Ctrl Pts',(22.1541362151734,2.24859589686446,-7.58200764778882));
#132134=CARTESIAN_POINT('Ctrl Pts',(22.2053740476789,2.23810210760964,-7.58516556324541));
#132135=CARTESIAN_POINT('Ctrl Pts',(22.2541175370563,2.2281191735147,-7.58816974611158));
#132136=CARTESIAN_POINT('Ctrl Pts',(22.3022612073645,2.21528748032301,-7.59112111119599));
#132137=CARTESIAN_POINT('Ctrl Pts',(22.3494498385149,2.19969130365015,-7.59405532906684));
#132138=CARTESIAN_POINT('Ctrl Pts',(22.3966670638231,2.18408567640569,-7.59699132493987));
#132139=CARTESIAN_POINT('Ctrl Pts',(22.4429278437337,2.1657118074518,-7.59991056701147));
#132140=CARTESIAN_POINT('Ctrl Pts',(22.4878809656186,2.14469709134001,-7.6028668328478));
#132141=CARTESIAN_POINT('Ctrl Pts',(22.529366180175,2.12530355491394,-7.60559503763901));
#132142=CARTESIAN_POINT('Ctrl Pts',(22.5697380353023,2.10366051473313,-7.60835536247661));
#132143=CARTESIAN_POINT('Ctrl Pts',(22.6087263589705,2.07990721782239,-7.61119777667448));
#132144=CARTESIAN_POINT('Ctrl Pts',(22.6120553107308,2.07787908293164,-7.61144047138041));
#132145=CARTESIAN_POINT('Ctrl Pts',(22.6153742075372,2.07583556573303,-7.61168376454307));
#132146=CARTESIAN_POINT('Ctrl Pts',(22.6186828988705,2.07377675361698,-7.61192768726687));
#132147=CARTESIAN_POINT('Ctrl Pts',(22.624990550176,2.06985185775231,-7.61239269875699));
#132148=CARTESIAN_POINT('Ctrl Pts',(22.6312610057396,2.06587146792896,-7.61286000399756));
#132149=CARTESIAN_POINT('Ctrl Pts',(22.6374931440773,2.0618362937874,-7.61332982037423));
#132150=CARTESIAN_POINT('Ctrl Pts',(22.6375075149939,2.06182698893121,-7.61333090374106));
#132151=CARTESIAN_POINT('Ctrl Pts',(22.6375218857067,2.06181768378373,-7.61333198712124));
#132152=CARTESIAN_POINT('Ctrl Pts',(22.6375362562159,2.06180837834495,-7.61333307051478));
#132153=CARTESIAN_POINT('Ctrl Pts',(22.6760163315447,2.03689109935326,-7.61623408568443));
#132154=CARTESIAN_POINT('Ctrl Pts',(22.7131727705318,2.00978722455919,-7.61923826595538));
#132155=CARTESIAN_POINT('Ctrl Pts',(22.7487706957536,1.9806824384814,-7.62228650201306));
#132156=CARTESIAN_POINT('Ctrl Pts',(22.7526465906051,1.97751351529805,-7.62261839333449));
#132157=CARTESIAN_POINT('Ctrl Pts',(22.7565039924891,1.97432091962232,-7.62295080692892));
#132158=CARTESIAN_POINT('Ctrl Pts',(22.7603425867873,1.97110492650524,-7.62328366650101));
#132159=CARTESIAN_POINT('Ctrl Pts',(22.7983076326772,1.93929762498099,-7.62657576458379));
#132160=CARTESIAN_POINT('Ctrl Pts',(22.8344355438025,1.90519639880607,-7.62991093927537));
#132161=CARTESIAN_POINT('Ctrl Pts',(22.8684698064752,1.86906184187726,-7.63323037612235));
#132162=CARTESIAN_POINT('Ctrl Pts',(22.9024723351439,1.83296097729504,-7.63654671788179));
#132163=CARTESIAN_POINT('Ctrl Pts',(22.934385387942,1.79483073315077,-7.63984705746996));
#132164=CARTESIAN_POINT('Ctrl Pts',(22.9639851264058,1.75495155551915,-7.64309411880228));
#132165=CARTESIAN_POINT('Ctrl Pts',(22.9935696890332,1.71509282400997,-7.6463395153607));
#132166=CARTESIAN_POINT('Ctrl Pts',(23.0208433831259,1.67348698760192,-7.64953159260903));
#132167=CARTESIAN_POINT('Ctrl Pts',(23.0456120952103,1.63043326522119,-7.65265733638432));
#132168=CARTESIAN_POINT('Ctrl Pts',(23.0703785031404,1.58738354799096,-7.65578278938164));
#132169=CARTESIAN_POINT('Ctrl Pts',(23.0926403011044,1.5428861967377,-7.65884197039542));
#132170=CARTESIAN_POINT('Ctrl Pts',(23.1122329880627,1.49725945430186,-7.66184640247652));
#132171=CARTESIAN_POINT('Ctrl Pts',(23.1318446678839,1.45158848197234,-7.66485374700992));
#132172=CARTESIAN_POINT('Ctrl Pts',(23.1487817982646,1.40478588088184,-7.66780643108939));
#132173=CARTESIAN_POINT('Ctrl Pts',(23.1629116716654,1.35719047428455,-7.6707387994773));
#132174=CARTESIAN_POINT('Ctrl Pts',(23.1770499431126,1.3095667795047,-7.67367291070928));
#132175=CARTESIAN_POINT('Ctrl Pts',(23.1883771606077,1.26114930976549,-7.67658707921416));
#132176=CARTESIAN_POINT('Ctrl Pts',(23.1967980253659,1.21229778702165,-7.67953413838556));
#132177=CARTESIAN_POINT('Ctrl Pts',(23.2046207261191,1.16691636186671,-7.68227185745146));
#132178=CARTESIAN_POINT('Ctrl Pts',(23.2099351229296,1.1211599033523,-7.68503853732298));
#132179=CARTESIAN_POINT('Ctrl Pts',(23.2127007083018,1.07533422374036,-7.68788493701758));
#132180=CARTESIAN_POINT('Ctrl Pts',(23.2129172043911,1.07174688902004,-7.68810775942936));
#132181=CARTESIAN_POINT('Ctrl Pts',(23.2131180972758,1.06815910911293,-7.68833107037233));
#132182=CARTESIAN_POINT('Ctrl Pts',(23.2133033754879,1.06457101979013,-7.68855489419667));
#132183=CARTESIAN_POINT('Ctrl Pts',(23.2138397980788,1.05418268459507,-7.68920291510772));
#132184=CARTESIAN_POINT('Ctrl Pts',(23.2142453641124,1.04379202600083,-7.68985524985652));
#132185=CARTESIAN_POINT('Ctrl Pts',(23.2145199279081,1.03340268179491,-7.69051249873406));
#132186=CARTESIAN_POINT('Ctrl Pts',(23.2145203733976,1.03338582471378,-7.69051356514378));
#132187=CARTESIAN_POINT('Ctrl Pts',(23.2145208185423,1.03336896763607,-7.69051463156644));
#132188=CARTESIAN_POINT('Ctrl Pts',(23.2145212633422,1.03335211056181,-7.69051569800203));
#132189=CARTESIAN_POINT('Ctrl Pts',(23.2157322627867,0.987457518342025,
-7.69341914531073));
#132190=CARTESIAN_POINT('Ctrl Pts',(23.2143838631422,0.941419993553586,
-7.696425913793));
#132191=CARTESIAN_POINT('Ctrl Pts',(23.2104968860145,0.89553884262516,-7.69947702839088));
#132192=CARTESIAN_POINT('Ctrl Pts',(23.2100805041421,0.890623948891015,
-7.69980387075895));
#132193=CARTESIAN_POINT('Ctrl Pts',(23.2096350206477,0.885710889393794,
-7.70013122200685));
#132194=CARTESIAN_POINT('Ctrl Pts',(23.2091604827784,0.880800060007226,
-7.70045900963963));
#132195=CARTESIAN_POINT('Ctrl Pts',(23.2043858980581,0.831389523005676,
-7.70375706006715));
#132196=CARTESIAN_POINT('Ctrl Pts',(23.1966671585257,0.78219967260526,-7.70709872997302));
#132197=CARTESIAN_POINT('Ctrl Pts',(23.1860747987745,0.733590953170563,
-7.7104251143462));
#132198=CARTESIAN_POINT('Ctrl Pts',(23.1754923989363,0.685027940134408,
-7.71374837094617));
#132199=CARTESIAN_POINT('Ctrl Pts',(23.1620420686208,0.637044828130932,
-7.71705607456978));
#132200=CARTESIAN_POINT('Ctrl Pts',(23.1458291743831,0.58998621565744,-7.72031086711321));
#132201=CARTESIAN_POINT('Ctrl Pts',(23.1296248204055,0.542952391650794,
-7.72356394517098));
#132202=CARTESIAN_POINT('Ctrl Pts',(23.1106608825592,0.496842046723612,
-7.72676407167276));
#132203=CARTESIAN_POINT('Ctrl Pts',(23.0890749877739,0.451985841145882,
-7.7298981806231));
#132204=CARTESIAN_POINT('Ctrl Pts',(23.0664157400106,0.4048991724663,-7.73318813232209));
#132205=CARTESIAN_POINT('Ctrl Pts',(23.0408669082453,0.359194672498317,
-7.73640516982291));
#132206=CARTESIAN_POINT('Ctrl Pts',(23.0126262367103,0.315238760789114,
-7.73956328124471));
#132207=CARTESIAN_POINT('Ctrl Pts',(22.9857011055717,0.273330455399889,
-7.74257427778128));
#132208=CARTESIAN_POINT('Ctrl Pts',(22.9563291669508,0.23301169809954,-7.74553212191393));
#132209=CARTESIAN_POINT('Ctrl Pts',(22.9247173003245,0.194584147349198,
-7.74847216961083));
#132210=CARTESIAN_POINT('Ctrl Pts',(22.8930869336765,0.156134107875608,
-7.75141393789406));
#132211=CARTESIAN_POINT('Ctrl Pts',(22.8592137257373,0.119577866736777,
-7.75433830227743));
#132212=CARTESIAN_POINT('Ctrl Pts',(22.823343318757,0.0851978454080979,
-7.75729874603043));
#132213=CARTESIAN_POINT('Ctrl Pts',(22.7902114398814,0.053442568613225,
-7.76003317454963));
#132214=CARTESIAN_POINT('Ctrl Pts',(22.7553751894399,0.0235437599775924,
-7.76279897204339));
#132215=CARTESIAN_POINT('Ctrl Pts',(22.7190626003208,-0.00429562954898666,
-7.76564603671213));
#132216=CARTESIAN_POINT('Ctrl Pts',(22.7159978115506,-0.0066452788154652,
-7.76588632946007));
#132217=CARTESIAN_POINT('Ctrl Pts',(22.7129224970894,-0.00898028741680565,
-7.76612720110572));
#132218=CARTESIAN_POINT('Ctrl Pts',(22.709836788526,-0.0113005494724608,
-7.76636868164864));
#132219=CARTESIAN_POINT('Ctrl Pts',(22.7041614586551,-0.015568046639597,
-7.7668128200727));
#132220=CARTESIAN_POINT('Ctrl Pts',(22.6984510815102,-0.0197856005600674,
-7.76725902354423));
#132221=CARTESIAN_POINT('Ctrl Pts',(22.6927065844721,-0.0239525210596693,
-7.76770748047895));
#132222=CARTESIAN_POINT('Ctrl Pts',(22.6926933515776,-0.0239621198842663,
-7.76770851353428));
#132223=CARTESIAN_POINT('Ctrl Pts',(22.692680118502,-0.0239717184401977,
-7.76770954660158));
#132224=CARTESIAN_POINT('Ctrl Pts',(22.6926668852454,-0.023981316727459,
-7.76771057968083));
#132225=CARTESIAN_POINT('Ctrl Pts',(22.6554388968025,-0.0509833569147772,
-7.77061685314098));
#132226=CARTESIAN_POINT('Ctrl Pts',(22.6166406046479,-0.0759494362312827,
-7.77362497912796));
#132227=CARTESIAN_POINT('Ctrl Pts',(22.5765325545742,-0.0987262866689894,
-7.77667567508239));
#132228=CARTESIAN_POINT('Ctrl Pts',(22.573441076479,-0.100481897676706,
-7.7769108188927));
#132229=CARTESIAN_POINT('Ctrl Pts',(22.5703418425734,-0.102224502742977,
-7.77714621561684));
#132230=CARTESIAN_POINT('Ctrl Pts',(22.567234984968,-0.103954032305686,
-7.77738183810724));
#132231=CARTESIAN_POINT('Ctrl Pts',(22.5238893488562,-0.128083737812819,
-7.78066914896143));
#132232=CARTESIAN_POINT('Ctrl Pts',(22.4790542550743,-0.149668720445147,
-7.7839998130839));
#132233=CARTESIAN_POINT('Ctrl Pts',(22.4330660295219,-0.168562331668783,
-7.78731510173064));
#132234=CARTESIAN_POINT('Ctrl Pts',(22.4190094916684,-0.174337261189623,
-7.78832843677017));
#132235=CARTESIAN_POINT('Ctrl Pts',(22.4048452798424,-0.179861028530698,
-7.78934047221547));
#132236=CARTESIAN_POINT('Ctrl Pts',(22.3905831448079,-0.185130158742937,
-7.79034991681389));
#132237=CARTESIAN_POINT('Ctrl Pts',(22.3906127226216,-0.185251306744425,
-7.65234642888876));
#132238=CARTESIAN_POINT('Ctrl Pts',(22.4940424169462,-0.146801704427007,
-7.64566717319121));
#132239=CARTESIAN_POINT('Ctrl Pts',(22.5919934936769,-0.0949807286400788,
-7.63944789248604));
#132240=CARTESIAN_POINT('Ctrl Pts',(22.7077125771348,-0.0128315743679774,
-7.63118841723727));
#132241=CARTESIAN_POINT('Ctrl Pts',(22.7327516429826,0.0063925361648165,
-7.62933424545274));
#132242=CARTESIAN_POINT('Ctrl Pts',(22.7753917363593,0.0417428777677298,
-7.6260084691289));
#132243=CARTESIAN_POINT('Ctrl Pts',(22.7933044962324,0.0574685179146428,
-7.62455491237901));
#132244=CARTESIAN_POINT('Ctrl Pts',(22.8227144533301,0.0847973108693356,
-7.62205043756754));
#132245=CARTESIAN_POINT('Ctrl Pts',(22.8344499695325,0.0961334981816853,
-7.62101644374416));
#132246=CARTESIAN_POINT('Ctrl Pts',(22.8639477218394,0.12575213502005,-7.6183269698318));
#132247=CARTESIAN_POINT('Ctrl Pts',(22.8813810725006,0.144348860910135,
-7.61665160440707));
#132248=CARTESIAN_POINT('Ctrl Pts',(22.9513597169633,0.223671251125492,
-7.60960261042078));
#132249=CARTESIAN_POINT('Ctrl Pts',(22.9986229118508,0.288805660495983,
-7.60405383489559));
#132250=CARTESIAN_POINT('Ctrl Pts',(23.060750159107,0.394224365295095,-7.59575737106788));
#132251=CARTESIAN_POINT('Ctrl Pts',(23.0802892046431,0.431513556256866,
-7.59293585966622));
#132252=CARTESIAN_POINT('Ctrl Pts',(23.1127497622266,0.501781882236911,
-7.58784193887245));
#132253=CARTESIAN_POINT('Ctrl Pts',(23.1262158014048,0.534462604559476,
-7.58555598900005));
#132254=CARTESIAN_POINT('Ctrl Pts',(23.1479082255124,0.594085705701977,
-7.58152803989586));
#132255=CARTESIAN_POINT('Ctrl Pts',(23.1566368407822,0.620818967804944,
-7.57977133114387));
#132256=CARTESIAN_POINT('Ctrl Pts',(23.1749937836985,0.684122058989001,
-7.57571453740653));
#132257=CARTESIAN_POINT('Ctrl Pts',(23.1838879440589,0.720877145462882,
-7.57343804270218));
#132258=CARTESIAN_POINT('Ctrl Pts',(23.207917352637,0.844103409480788,-7.56599633376565));
#132259=CARTESIAN_POINT('Ctrl Pts',(23.2157015819628,0.931740373279695,
-7.56102594549));
#132260=CARTESIAN_POINT('Ctrl Pts',(23.2138604855805,1.05125058285275,-7.5540717139137));
#132261=CARTESIAN_POINT('Ctrl Pts',(23.212173544829,1.08299198344224,-7.55220547357544));
#132262=CARTESIAN_POINT('Ctrl Pts',(23.2071232470018,1.13847108866683,-7.54886151670606));
#132263=CARTESIAN_POINT('Ctrl Pts',(23.2042771510702,1.1622398388433,-7.54740216036922));
#132264=CARTESIAN_POINT('Ctrl Pts',(23.1983596272575,1.20205116755439,-7.54489190879501));
#132265=CARTESIAN_POINT('Ctrl Pts',(23.1956489309375,1.21814008823688,-7.54385821474024));
#132266=CARTESIAN_POINT('Ctrl Pts',(23.187928302395,1.25910935359935,-7.54117645965506));
#132267=CARTESIAN_POINT('Ctrl Pts',(23.182479673952,1.28389751965807,-7.53950880388485));
#132268=CARTESIAN_POINT('Ctrl Pts',(23.1567165702479,1.38630501446538,-7.53247368416446));
#132269=CARTESIAN_POINT('Ctrl Pts',(23.1297844725607,1.46206581161866,-7.52693026664844));
#132270=CARTESIAN_POINT('Ctrl Pts',(23.0780072942364,1.57301065407658,-7.51862840776639));
#132271=CARTESIAN_POINT('Ctrl Pts',(23.0582527008603,1.61034261579051,-7.51579724109893));
#132272=CARTESIAN_POINT('Ctrl Pts',(23.0185615338199,1.67704503166432,-7.51068859432403));
#132273=CARTESIAN_POINT('Ctrl Pts',(22.999185591811,1.70669915764103,-7.50839743056693));
#132274=CARTESIAN_POINT('Ctrl Pts',(22.9622239499138,1.75838939182723,-7.50436283716511));
#132275=CARTESIAN_POINT('Ctrl Pts',(22.945098841732,1.78072420267642,-7.50260457167021));
#132276=CARTESIAN_POINT('Ctrl Pts',(22.9032619088592,1.83167286462451,-7.49854654235209));
#132277=CARTESIAN_POINT('Ctrl Pts',(22.8779838591178,1.8597873932142,-7.49627028810481));
#132278=CARTESIAN_POINT('Ctrl Pts',(22.7865360348136,1.9527566981103,-7.48853950837726));
#132279=CARTESIAN_POINT('Ctrl Pts',(22.71453501403,2.01144637887395,-7.48330926971999));
#132280=CARTESIAN_POINT('Ctrl Pts',(22.6019953159732,2.08424059208809,-7.47548431391633));
#132281=CARTESIAN_POINT('Ctrl Pts',(22.5661384742771,2.10501055167859,-7.47303182357788));
#132282=CARTESIAN_POINT('Ctrl Pts',(22.5135061497038,2.13213868372751,-7.46939923328097));
#132283=CARTESIAN_POINT('Ctrl Pts',(22.4975115635861,2.13995974178171,-7.46829110514068));
#132284=CARTESIAN_POINT('Ctrl Pts',(22.4643986880383,2.15529369003329,-7.46597801943084));
#132285=CARTESIAN_POINT('Ctrl Pts',(22.4472685292147,2.16276972783158,-7.46477174353053));
#132286=CARTESIAN_POINT('Ctrl Pts',(22.3907808842619,2.18594590488653,-7.46077687256424));
#132287=CARTESIAN_POINT('Ctrl Pts',(22.350801022297,2.20004726641911,-7.45792353638843));
#132288=CARTESIAN_POINT('Ctrl Pts',(22.2412256319327,2.23260874400658,-7.45015260210442));
#132289=CARTESIAN_POINT('Ctrl Pts',(22.1706305908785,2.24718078234766,-7.44520570761822));
#132290=CARTESIAN_POINT('Ctrl Pts',(22.064982496159,2.25973215937322,-7.4380732599374));
#132291=CARTESIAN_POINT('Ctrl Pts',(22.0306332055258,2.26239640582401,-7.43579387888845));
#132292=CARTESIAN_POINT('Ctrl Pts',(21.964834184023,2.26480287394941,-7.43150841673015));
#132293=CARTESIAN_POINT('Ctrl Pts',(21.9334189453514,2.26478128611373,-7.4294973769525));
#132294=CARTESIAN_POINT('Ctrl Pts',(21.8735417530957,2.26250838197262,-7.42572513855168));
#132295=CARTESIAN_POINT('Ctrl Pts',(21.8450919047288,2.26046331327807,-7.42395903110725));
#132296=CARTESIAN_POINT('Ctrl Pts',(21.7702245754135,2.25252882291126,-7.41936508256022));
#132297=CARTESIAN_POINT('Ctrl Pts',(21.7240220470378,2.24502299084699,-7.41658606110863));
#132298=CARTESIAN_POINT('Ctrl Pts',(21.6013294761016,2.21803382440755,-7.40923607717549));
#132299=CARTESIAN_POINT('Ctrl Pts',(21.5260772287764,2.19392900240862,-7.40476688660263));
#132300=CARTESIAN_POINT('Ctrl Pts',(21.4280404131668,2.15208006521468,-7.39852815817694));
#132301=CARTESIAN_POINT('Ctrl Pts',(21.4028861130073,2.14034929418271,-7.39688652492375));
#132302=CARTESIAN_POINT('Ctrl Pts',(21.3585966046755,2.1178919537636,-7.39388849054287));
#132303=CARTESIAN_POINT('Ctrl Pts',(21.3393158888165,2.10747694400457,-7.39254519573733));
#132304=CARTESIAN_POINT('Ctrl Pts',(21.3060099155187,2.08835161129564,-7.39014025546559));
#132305=CARTESIAN_POINT('Ctrl Pts',(21.2918672857805,2.07985817811305,-7.38909025232836));
#132306=CARTESIAN_POINT('Ctrl Pts',(21.2537909873064,2.05596547979712,-7.38618732685736));
#132307=CARTESIAN_POINT('Ctrl Pts',(21.2302057659276,2.04003177582916,-7.38430683217135));
#132308=CARTESIAN_POINT('Ctrl Pts',(21.1426578145012,1.97648124603869,-7.37706120409505));
#132309=CARTESIAN_POINT('Ctrl Pts',(21.082710517875,1.92364829631565,-7.37155182614802));
#132310=CARTESIAN_POINT('Ctrl Pts',(20.9894976562408,1.82436776290702,-7.36233988963408));
#132311=CARTESIAN_POINT('Ctrl Pts',(20.9536540357179,1.78066832010741,-7.35858625454727));
#132312=CARTESIAN_POINT('Ctrl Pts',(20.9036342900622,1.71060309154341,-7.35302492959291));
#132313=CARTESIAN_POINT('Ctrl Pts',(20.8872727047603,1.68589275824092,-7.35114118363483));
#132314=CARTESIAN_POINT('Ctrl Pts',(20.856064081108,1.63495741887035,-7.34740385023755));
#132315=CARTESIAN_POINT('Ctrl Pts',(20.8412559616005,1.60873113725932,-7.34555246927876));
#132316=CARTESIAN_POINT('Ctrl Pts',(20.8016048229586,1.53224915517022,-7.34033520065384));
#132317=CARTESIAN_POINT('Ctrl Pts',(20.779146682433,1.48083680418887,-7.33704665955409));
#132318=CARTESIAN_POINT('Ctrl Pts',(20.7377482843471,1.36577726456233,-7.32995734862329));
#132319=CARTESIAN_POINT('Ctrl Pts',(20.7202567895926,1.30179175836331,-7.32618408331455));
#132320=CARTESIAN_POINT('Ctrl Pts',(20.7011034060175,1.20129378299635,-7.32017645307106));
#132321=CARTESIAN_POINT('Ctrl Pts',(20.6958695030891,1.165584249061,-7.31802512267355));
#132322=CARTESIAN_POINT('Ctrl Pts',(20.6903982972497,1.11252578400097,-7.31474267246062));
#132323=CARTESIAN_POINT('Ctrl Pts',(20.6889791408844,1.09531455843413,-7.31366449049371));
#132324=CARTESIAN_POINT('Ctrl Pts',(20.6867094072561,1.05862649599552,-7.31132845500143));
#132325=CARTESIAN_POINT('Ctrl Pts',(20.6859559202214,1.03914909123811,-7.31006674594604));
#132326=CARTESIAN_POINT('Ctrl Pts',(20.6841833830569,0.925175835434842,
-7.30258656709236));
#132327=CARTESIAN_POINT('Ctrl Pts',(20.6933100903781,0.830825266112662,
-7.29602917988473));
#132328=CARTESIAN_POINT('Ctrl Pts',(20.7214330497066,0.697841071848591,
-7.28681993620161));
#132329=CARTESIAN_POINT('Ctrl Pts',(20.7319924008396,0.657750486805098,
-7.28404389664926));
#132330=CARTESIAN_POINT('Ctrl Pts',(20.7550740262191,0.584863246294596,
-7.2790162876575));
#132331=CARTESIAN_POINT('Ctrl Pts',(20.767029088062,0.55192992193275,-7.27675199282445));
#132332=CARTESIAN_POINT('Ctrl Pts',(20.7910315881237,0.493497554231235,
-7.27274381050841));
#132333=CARTESIAN_POINT('Ctrl Pts',(20.8025930471859,0.467825233822383,
-7.2709860327521));
#132334=CARTESIAN_POINT('Ctrl Pts',(20.831874929885,0.408204866226418,-7.26690003541734));
#132335=CARTESIAN_POINT('Ctrl Pts',(20.8502993136262,0.374632950242004,
-7.26459659104704));
#132336=CARTESIAN_POINT('Ctrl Pts',(20.9158058648428,0.267145273476332,
-7.25714151648513));
#132337=CARTESIAN_POINT('Ctrl Pts',(20.9690395420465,0.197285777983223,
-7.25218070410798));
#132338=CARTESIAN_POINT('Ctrl Pts',(21.0505237594515,0.110683815647943,
-7.24525768449972));
#132339=CARTESIAN_POINT('Ctrl Pts',(21.072819747555,0.0886848127540274,
-7.24341714949713));
#132340=CARTESIAN_POINT('Ctrl Pts',(21.1133937292975,0.0515209482369094,
-7.24011225500614));
#132341=CARTESIAN_POINT('Ctrl Pts',(21.1313254804036,0.0360008121798749,
-7.23866560485725));
#132342=CARTESIAN_POINT('Ctrl Pts',(21.1623242857697,0.0106598629329513,
-7.23616735567625));
#132343=CARTESIAN_POINT('Ctrl Pts',(21.1751639987662,0.000572149131192745,
-7.23513233418825));
#132344=CARTESIAN_POINT('Ctrl Pts',(21.2086825114943,-0.0247280162274421,
-7.23242982649631));
#132345=CARTESIAN_POINT('Ctrl Pts',(21.2296341052558,-0.0395633249824545,
-7.23074200674234));
#132346=CARTESIAN_POINT('Ctrl Pts',(21.3180287714083,-0.0981977629417452,
-7.22367123082529));
#132347=CARTESIAN_POINT('Ctrl Pts',(21.3891218927,-0.136152072304188,-7.21811451497419));
#132348=CARTESIAN_POINT('Ctrl Pts',(21.5183012720179,-0.190018021893765,
-7.20862726820053));
#132349=CARTESIAN_POINT('Ctrl Pts',(21.5748216979094,-0.2090283171575,-7.2046571878587));
#132350=CARTESIAN_POINT('Ctrl Pts',(21.6613674114336,-0.23147970068488,
-7.19887484487606));
#132351=CARTESIAN_POINT('Ctrl Pts',(21.6905147517321,-0.237949377262141,
-7.19697507338289));
#132352=CARTESIAN_POINT('Ctrl Pts',(21.7492376808955,-0.248818246759099,
-7.19323519072459));
#132353=CARTESIAN_POINT('Ctrl Pts',(21.7787945913569,-0.253212450465656,
-7.19139632435182));
#132354=CARTESIAN_POINT('Ctrl Pts',(21.9175884525327,-0.268844003782043,
-7.18292820284992));
#132355=CARTESIAN_POINT('Ctrl Pts',(22.0278267950562,-0.266869947744044,
-7.17673034198916));
#132356=CARTESIAN_POINT('Ctrl Pts',(22.1686816030147,-0.245873999258075,
-7.16845195434581));
#132357=CARTESIAN_POINT('Ctrl Pts',(22.2007356751181,-0.239820572247473,
-7.16653915378911));
#132358=CARTESIAN_POINT('Ctrl Pts',(22.2562405272078,-0.227097918076251,
-7.16312433805001));
#132359=CARTESIAN_POINT('Ctrl Pts',(22.2797994072487,-0.220976961557628,
-7.16164183438522));
#132360=CARTESIAN_POINT('Ctrl Pts',(22.3188292636876,-0.209624457519522,
-7.15910836628414));
#132361=CARTESIAN_POINT('Ctrl Pts',(22.3344011562343,-0.204766381414831,
-7.15807567944551));
#132362=CARTESIAN_POINT('Ctrl Pts',(22.363536087041,-0.195054599578651,
-7.15610141683161));
#132363=CARTESIAN_POINT('Ctrl Pts',(22.3771172669733,-0.190268191947343,
-7.15516422911284));
#132364=CARTESIAN_POINT('Ctrl Pts',(22.3906127227906,-0.185251306681596,
-7.15421791561113));
#132365=CARTESIAN_POINT('Origin',(21.9499999789786,0.999999999999992,-6.00000000000001));
#132366=CARTESIAN_POINT('',(22.3906127230289,-0.185251306593042,-6.65225448505536));
#132367=CARTESIAN_POINT('',(22.3905561784951,-0.18502046241637,-6.79053837538029));
#132368=CARTESIAN_POINT('',(22.3906127231008,-0.185251306566283,-6.00000000000001));
#132369=CARTESIAN_POINT('',(20.6856937166152,0.999065229854255,-6.94375443275021));
#132370=CARTESIAN_POINT('Ctrl Pts',(22.3905561778436,-0.185020462657188,
-6.79053837542619));
#132371=CARTESIAN_POINT('Ctrl Pts',(22.3439699936583,-0.20224093581996,
-6.79382028946338));
#132372=CARTESIAN_POINT('Ctrl Pts',(22.2963454492253,-0.216746426185838,
-6.79706020776744));
#132373=CARTESIAN_POINT('Ctrl Pts',(22.2480258339149,-0.228436764308156,
-6.80023594852031));
#132374=CARTESIAN_POINT('Ctrl Pts',(22.199718524656,-0.240124125132281,
-6.80341088047474));
#132375=CARTESIAN_POINT('Ctrl Pts',(22.1507165053392,-0.248997734601995,
-6.80652166575826));
#132376=CARTESIAN_POINT('Ctrl Pts',(22.1013714506626,-0.254991265143792,
-6.80957082217001));
#132377=CARTESIAN_POINT('Ctrl Pts',(22.051984798257,-0.26098984821335,-6.81262254901122));
#132378=CARTESIAN_POINT('Ctrl Pts',(22.002254556072,-0.264103293065579,
-6.81561267971874));
#132379=CARTESIAN_POINT('Ctrl Pts',(21.952541740764,-0.264300704134091,
-6.81856747133101));
#132380=CARTESIAN_POINT('Ctrl Pts',(21.9028067785013,-0.26449820314882,
-6.82152357929674));
#132381=CARTESIAN_POINT('Ctrl Pts',(21.8530893382183,-0.261776695821649,
-6.82444463309553));
#132382=CARTESIAN_POINT('Ctrl Pts',(21.8037586542992,-0.256145149757803,
-6.8273773218159));
#132383=CARTESIAN_POINT('Ctrl Pts',(21.7543405399351,-0.250503622713768,
-6.83031520824001));
#132384=CARTESIAN_POINT('Ctrl Pts',(21.7053107951687,-0.241941155643439,
-6.83326533420195));
#132385=CARTESIAN_POINT('Ctrl Pts',(21.6570461311386,-0.230513961479585,
-6.83628857712534));
#132386=CARTESIAN_POINT('Ctrl Pts',(21.6291010198181,-0.223897646637129,
-6.83803902668799));
#132387=CARTESIAN_POINT('Ctrl Pts',(21.6014124921128,-0.216321883951753,
-6.83981421545855));
#132388=CARTESIAN_POINT('Ctrl Pts',(21.5740537671172,-0.207806077291614,
-6.84162671206072));
#132389=CARTESIAN_POINT('Ctrl Pts',(21.5740375959949,-0.207801043791291,
-6.84162778338639));
#132390=CARTESIAN_POINT('Ctrl Pts',(21.5740214249876,-0.207796009962646,
-6.84162885472508));
#132391=CARTESIAN_POINT('Ctrl Pts',(21.5740052540952,-0.207790975805693,
-6.84162992607682));
#132392=CARTESIAN_POINT('Ctrl Pts',(21.5301887526272,-0.194150470342384,
-6.84453285090531));
#132393=CARTESIAN_POINT('Ctrl Pts',(21.4870600614421,-0.178042935966803,
-6.84753884171575));
#132394=CARTESIAN_POINT('Ctrl Pts',(21.4448958919887,-0.159584333445583,
-6.85058879476411));
#132395=CARTESIAN_POINT('Ctrl Pts',(21.4403540045181,-0.157595988919839,
-6.85091733303999));
#132396=CARTESIAN_POINT('Ctrl Pts',(21.4358233375632,-0.155580404652721,
-6.85124638142775));
#132397=CARTESIAN_POINT('Ctrl Pts',(21.4313042568956,-0.153537755545344,
-6.85157586605306));
#132398=CARTESIAN_POINT('Ctrl Pts',(21.3861311093499,-0.133119246495114,
-6.85486942478502));
#132399=CARTESIAN_POINT('Ctrl Pts',(21.3421117789209,-0.10999206023659,
-6.85820602282507));
#132400=CARTESIAN_POINT('Ctrl Pts',(21.2995639830833,-0.0843384566189006,
-6.86152689828285));
#132401=CARTESIAN_POINT('Ctrl Pts',(21.2570558557206,-0.0587087705581764,
-6.86484467759752));
#132402=CARTESIAN_POINT('Ctrl Pts',(21.2160163016383,-0.0305576030157111,
-6.86814647008664));
#132403=CARTESIAN_POINT('Ctrl Pts',(21.1767369068999,-9.51095119867129E-5,
-6.87139508591847));
#132404=CARTESIAN_POINT('Ctrl Pts',(21.1374777418491,0.030351695187625,
-6.87464202864704));
#132405=CARTESIAN_POINT('Ctrl Pts',(21.0999768602153,0.0631073930715781,
-6.87783575437138));
#132406=CARTESIAN_POINT('Ctrl Pts',(21.0645022911954,0.0979357489692311,
-6.88096336386761));
#132407=CARTESIAN_POINT('Ctrl Pts',(21.0271682715109,0.134589683339287,
-6.88425491152339));
#132408=CARTESIAN_POINT('Ctrl Pts',(20.9920788931084,0.173539570838059,
-6.88747304910112));
#132409=CARTESIAN_POINT('Ctrl Pts',(20.9595186796348,0.214478450135798,
-6.89063209350199));
#132410=CARTESIAN_POINT('Ctrl Pts',(20.928552990418,0.253412488889815,-6.89363643458897));
#132411=CARTESIAN_POINT('Ctrl Pts',(20.8998748503192,0.294145362371813,
-6.89658775113724));
#132412=CARTESIAN_POINT('Ctrl Pts',(20.8737024166744,0.336384547288791,
-6.89952161411312));
#132413=CARTESIAN_POINT('Ctrl Pts',(20.8475141232985,0.378649327919265,
-6.90245725492435));
#132414=CARTESIAN_POINT('Ctrl Pts',(20.8238350245176,0.422422397756516,
-6.90537583380583));
#132415=CARTESIAN_POINT('Ctrl Pts',(20.802852535304,0.467380785622911,-6.90833104940879));
#132416=CARTESIAN_POINT('Ctrl Pts',(20.7834786740189,0.508892427128444,
-6.91105970264801));
#132417=CARTESIAN_POINT('Ctrl Pts',(20.7664038099828,0.551415116425624,
-6.91382017768355));
#132418=CARTESIAN_POINT('Ctrl Pts',(20.7517458282314,0.594668391099852,
-6.9166624960234));
#132419=CARTESIAN_POINT('Ctrl Pts',(20.7505025216512,0.598337182747256,
-6.91690358467768));
#132420=CARTESIAN_POINT('Ctrl Pts',(20.7492765785363,0.602011249014336,
-6.91714526216378));
#132421=CARTESIAN_POINT('Ctrl Pts',(20.7480680571252,0.605690429331247,
-6.91738755900762));
#132422=CARTESIAN_POINT('Ctrl Pts',(20.7457352261486,0.612792418367502,
-6.91785526903547));
#132423=CARTESIAN_POINT('Ctrl Pts',(20.7434673324641,0.619913322422839,
-6.91832529279064));
#132424=CARTESIAN_POINT('Ctrl Pts',(20.7412647880579,0.627051853772677,
-6.9187978518838));
#132425=CARTESIAN_POINT('Ctrl Pts',(20.7412597946966,0.627068037449193,
-6.9187989232167));
#132426=CARTESIAN_POINT('Ctrl Pts',(20.7412548016711,0.627084221216311,
-6.91879999456263));
#132427=CARTESIAN_POINT('Ctrl Pts',(20.7412498089815,0.627100405074025,
-6.91880106592159));
#132428=CARTESIAN_POINT('Ctrl Pts',(20.7269381749478,0.673491722735542,
-6.92187213556098));
#132429=CARTESIAN_POINT('Ctrl Pts',(20.7153550167606,0.720746816475562,
-6.92505507810059));
#132430=CARTESIAN_POINT('Ctrl Pts',(20.7065458452856,0.768570366770981,
-6.92828331058919));
#132431=CARTESIAN_POINT('Ctrl Pts',(20.7046661143239,0.778775118539138,
-6.92897216181401));
#132432=CARTESIAN_POINT('Ctrl Pts',(20.7029127089235,0.789005565373911,
-6.92966307520232));
#132433=CARTESIAN_POINT('Ctrl Pts',(20.7012860861758,0.799258531203285,
-6.93035540384252));
#132434=CARTESIAN_POINT('Ctrl Pts',(20.6932986460189,0.849605147289468,
-6.93375504496431));
#132435=CARTESIAN_POINT('Ctrl Pts',(20.6883673085457,0.900501158509976,
-6.93718806872723));
#132436=CARTESIAN_POINT('Ctrl Pts',(20.6865206510876,0.951614527893218,
-6.94059901766862));
#132437=CARTESIAN_POINT('Ctrl Pts',(20.6862523792291,0.959039986546106,
-6.94109454086807));
#132438=CARTESIAN_POINT('Ctrl Pts',(20.6860492463712,0.966469951088698,
-6.94158959818679));
#132439=CARTESIAN_POINT('Ctrl Pts',(20.6859113746941,0.973903318693967,
-6.94208401959448));
#132440=CARTESIAN_POINT('Ctrl Pts',(20.6857558836499,0.982286636539075,
-6.94264162578728));
#132441=CARTESIAN_POINT('Ctrl Pts',(20.6856832995832,0.990674430511361,
-6.943198488816));
#132442=CARTESIAN_POINT('Ctrl Pts',(20.6856937166151,0.999065229854251,
-6.94375443275022));
#132443=CARTESIAN_POINT('Ctrl Pts',(20.685693716616,0.999065230477396,-6.94375443279149));
#132444=CARTESIAN_POINT('Ctrl Pts',(20.6857551278917,1.0485312865077,-6.94703187426906));
#132445=CARTESIAN_POINT('Ctrl Pts',(20.6887020793451,1.09803110754432,-6.95027188392369));
#132446=CARTESIAN_POINT('Ctrl Pts',(20.6945091701822,1.14721024717709,-6.95344961851266));
#132447=CARTESIAN_POINT('Ctrl Pts',(20.7003144327648,1.19637390367318,-6.95662635265104));
#132448=CARTESIAN_POINT('Ctrl Pts',(20.7089780416456,1.24521705585266,-6.95974083149961));
#132449=CARTESIAN_POINT('Ctrl Pts',(20.7204397803494,1.29338962554135,-6.96279253068962));
#132450=CARTESIAN_POINT('Ctrl Pts',(20.7319109841211,1.34160197598738,-6.96584674996327));
#132451=CARTESIAN_POINT('Ctrl Pts',(20.7461850959508,1.38914253792151,-6.9688382028184));
#132452=CARTESIAN_POINT('Ctrl Pts',(20.7631656009654,1.43566531597457,-6.97178998233388));
#132453=CARTESIAN_POINT('Ctrl Pts',(20.7801530496552,1.48220711814135,-6.97474296889227));
#132454=CARTESIAN_POINT('Ctrl Pts',(20.7998493943831,1.52773010249413,-6.97765653747682));
#132455=CARTESIAN_POINT('Ctrl Pts',(20.8221185135132,1.57189499446312,-6.98057444667909));
#132456=CARTESIAN_POINT('Ctrl Pts',(20.8444291451012,1.61614221538313,-6.98349779523359));
#132457=CARTESIAN_POINT('Ctrl Pts',(20.869322573561,1.65902587372874,-6.98642602058845));
#132458=CARTESIAN_POINT('Ctrl Pts',(20.8966168887807,1.7002163716426,-6.98941784958919));
#132459=CARTESIAN_POINT('Ctrl Pts',(20.9161665316061,1.72971920091432,-6.99156075692679));
#132460=CARTESIAN_POINT('Ctrl Pts',(20.9369469521193,1.7583535746909,-6.9937366703361));
#132461=CARTESIAN_POINT('Ctrl Pts',(20.9588752605237,1.78600436831953,-6.99596900134297));
#132462=CARTESIAN_POINT('Ctrl Pts',(20.958885784244,1.7860176383454,-6.99597007267172));
#132463=CARTESIAN_POINT('Ctrl Pts',(20.9588963082288,1.78603090814513,-6.99597114401347));
#132464=CARTESIAN_POINT('Ctrl Pts',(20.9589068324779,1.78604417771874,-6.99597221536821));
#132465=CARTESIAN_POINT('Ctrl Pts',(20.9874231821028,1.82199921804461,-6.99887514232692));
#132466=CARTESIAN_POINT('Ctrl Pts',(21.0179928358731,1.85642349262579,-7.00188113528414));
#132467=CARTESIAN_POINT('Ctrl Pts',(21.0504078929258,1.8891006848048,-7.00493109083005));
#132468=CARTESIAN_POINT('Ctrl Pts',(21.0538996320004,1.89262066098736,-7.0052596310186));
#132469=CARTESIAN_POINT('Ctrl Pts',(21.0574127359555,1.89612035267063,-7.00558868132818));
#132470=CARTESIAN_POINT('Ctrl Pts',(21.0609469098073,1.89959948170392,-7.00591816788382));
#132471=CARTESIAN_POINT('Ctrl Pts',(21.0962747177362,1.93437705841731,-7.00921173470899));
#132472=CARTESIAN_POINT('Ctrl Pts',(21.1337132810345,1.96710208179375,-7.01254834138308));
#132473=CARTESIAN_POINT('Ctrl Pts',(21.1729780749988,1.99754388043512,-7.01586922582333));
#132474=CARTESIAN_POINT('Ctrl Pts',(21.2122062616413,2.02795729760271,-7.01918701413921));
#132475=CARTESIAN_POINT('Ctrl Pts',(21.2532571421861,2.05609203131309,-7.02248881597173));
#132476=CARTESIAN_POINT('Ctrl Pts',(21.2958295897617,2.08175183975354,-7.02573744114571));
#132477=CARTESIAN_POINT('Ctrl Pts',(21.3383801118927,2.10739843301043,-7.02898439322933));
#132478=CARTESIAN_POINT('Ctrl Pts',(21.3824506079409,2.13057272766119,-7.03217812830337));
#132479=CARTESIAN_POINT('Ctrl Pts',(21.4277241149225,2.15110985535873,-7.03530574671623));
#132480=CARTESIAN_POINT('Ctrl Pts',(21.4753706061152,2.17272342451209,-7.03859729740664));
#132481=CARTESIAN_POINT('Ctrl Pts',(21.5243496983534,2.19141570151684,-7.04181543782941));
#132482=CARTESIAN_POINT('Ctrl Pts',(21.5742725134357,2.20703192480476,-7.04497448422916));
#132483=CARTESIAN_POINT('Ctrl Pts',(21.6217506221013,2.22188342596689,-7.04797883300236));
#132484=CARTESIAN_POINT('Ctrl Pts',(21.6700821660592,2.23395277606183,-7.0509301562539));
#132485=CARTESIAN_POINT('Ctrl Pts',(21.7189156529662,2.24314191431671,-7.05386402443837));
#132486=CARTESIAN_POINT('Ctrl Pts',(21.7677787313942,2.25233662089355,-7.05679967045252));
#132487=CARTESIAN_POINT('Ctrl Pts',(21.8171443403872,2.25864714910988,-7.05971825303604));
#132488=CARTESIAN_POINT('Ctrl Pts',(21.8666436667313,2.2620150884441,-7.06267347039033));
#132489=CARTESIAN_POINT('Ctrl Pts',(21.9123482058553,2.26512483005954,-7.06540213070079));
#132490=CARTESIAN_POINT('Ctrl Pts',(21.9581672161228,2.26572567292485,-7.06816261126618));
#132491=CARTESIAN_POINT('Ctrl Pts',(22.0037965948361,2.26380874167111,-7.07100493365448));
#132492=CARTESIAN_POINT('Ctrl Pts',(22.0076668306934,2.26364614958058,-7.07124601644665));
#132493=CARTESIAN_POINT('Ctrl Pts',(22.0115357284369,2.26346546078326,-7.07148768802967));
#132494=CARTESIAN_POINT('Ctrl Pts',(22.0154031173103,2.26326667882846,-7.07172997892714));
#132495=CARTESIAN_POINT('Ctrl Pts',(22.0228682888261,2.26288297255133,-7.07219766996248));
#132496=CARTESIAN_POINT('Ctrl Pts',(22.0303276993002,2.26243188135987,-7.07266767448959));
#132497=CARTESIAN_POINT('Ctrl Pts',(22.0377799992292,2.26191348507893,-7.07314021409209));
#132498=CARTESIAN_POINT('Ctrl Pts',(22.0377968933154,2.26191230989388,-7.07314128532176));
#132499=CARTESIAN_POINT('Ctrl Pts',(22.0378137873651,2.26191113436296,-7.07314235656445));
#132500=CARTESIAN_POINT('Ctrl Pts',(22.0378306813782,2.26190995848617,-7.07314342782018));
#132501=CARTESIAN_POINT('Ctrl Pts',(22.08361093453,2.25872350796018,-7.07604637089033));
#132502=CARTESIAN_POINT('Ctrl Pts',(22.1292898167375,2.25297790701657,-7.07905237820387));
#132503=CARTESIAN_POINT('Ctrl Pts',(22.1745713474598,2.24472229803669,-7.08210234591501));
#132504=CARTESIAN_POINT('Ctrl Pts',(22.1794486211828,2.24383308638455,-7.08243085794047));
#132505=CARTESIAN_POINT('Ctrl Pts',(22.1843212476966,2.24291478795741,-7.08275987997004));
#132506=CARTESIAN_POINT('Ctrl Pts',(22.1891888308828,2.24196748872918,-7.08308933814804));
#132507=CARTESIAN_POINT('Ctrl Pts',(22.2378496331668,2.23249742141138,-7.08638290266398));
#132508=CARTESIAN_POINT('Ctrl Pts',(22.2860112071759,2.22012577175817,-7.08971950473026));
#132509=CARTESIAN_POINT('Ctrl Pts',(22.3333224062371,2.20495675917564,-7.09304038328605));
#132510=CARTESIAN_POINT('Ctrl Pts',(22.3805894975061,2.18980188852287,-7.09635816581756));
#132511=CARTESIAN_POINT('Ctrl Pts',(22.4270079592013,2.17185513983666,-7.09965996060118));
#132512=CARTESIAN_POINT('Ctrl Pts',(22.4722456518536,2.15125389476901,-7.10290857893874));
#132513=CARTESIAN_POINT('Ctrl Pts',(22.5174600471837,2.13066325930182,-7.10615552424428));
#132514=CARTESIAN_POINT('Ctrl Pts',(22.5614949388929,2.10742092666226,-7.10934925276055));
#132515=CARTESIAN_POINT('Ctrl Pts',(22.604035107296,2.08169508090793,-7.11247686661958));
#132516=CARTESIAN_POINT('Ctrl Pts',(22.6488046503027,2.05462103768905,-7.11576838727938));
#132517=CARTESIAN_POINT('Ctrl Pts',(22.6919184439548,2.02479597004318,-7.11898650106652));
#132518=CARTESIAN_POINT('Ctrl Pts',(22.7330289434229,1.99245308442595,-7.12214552604287));
#132519=CARTESIAN_POINT('Ctrl Pts',(22.7721265717464,1.9616937860196,-7.12514987738834));
#132520=CARTESIAN_POINT('Ctrl Pts',(22.8094122162172,1.92865729892989,-7.12810120709323));
#132521=CARTESIAN_POINT('Ctrl Pts',(22.8446062298037,1.8935780652595,-7.13103508730942));
#132522=CARTESIAN_POINT('Ctrl Pts',(22.8798215691838,1.85847757534628,-7.13397074530875));
#132523=CARTESIAN_POINT('Ctrl Pts',(22.9129423386157,1.82133161119038,-7.13688934548987));
#132524=CARTESIAN_POINT('Ctrl Pts',(22.9437117976406,1.78241132324634,-7.13984458737692));
#132525=CARTESIAN_POINT('Ctrl Pts',(22.9721220955032,1.74647513819684,-7.1425732444586));
#132526=CARTESIAN_POINT('Ctrl Pts',(22.9985279273012,1.70902578404918,-7.14533372713626));
#132527=CARTESIAN_POINT('Ctrl Pts',(23.0227500061312,1.67030904664563,-7.148176055919));
#132528=CARTESIAN_POINT('Ctrl Pts',(23.02480474488,1.66702473809689,-7.14841716829948));
#132529=CARTESIAN_POINT('Ctrl Pts',(23.0268437980163,1.66373129740975,-7.14865886964349));
#132530=CARTESIAN_POINT('Ctrl Pts',(23.0288670718732,1.66042886747209,-7.14890119048505));
#132531=CARTESIAN_POINT('Ctrl Pts',(23.0327715173278,1.65405594987828,-7.14936881304894));
#132532=CARTESIAN_POINT('Ctrl Pts',(23.0366171472399,1.64764968808478,-7.14983874853652));
#132533=CARTESIAN_POINT('Ctrl Pts',(23.0404032646256,1.64121123969717,-7.15031121842487));
#132534=CARTESIAN_POINT('Ctrl Pts',(23.0404118505076,1.64119663905169,-7.15031228985776));
#132535=CARTESIAN_POINT('Ctrl Pts',(23.0404204360835,1.64118203824067,-7.15031336130368));
#132536=CARTESIAN_POINT('Ctrl Pts',(23.0404290213534,1.64116743726415,-7.15031443276264));
#132537=CARTESIAN_POINT('Ctrl Pts',(23.0636891555693,1.60160890523665,-7.15321734431571));
#132538=CARTESIAN_POINT('Ctrl Pts',(23.0847813867873,1.5606868188613,-7.15622332121024));
#132539=CARTESIAN_POINT('Ctrl Pts',(23.1035788700111,1.51867306745788,-7.15927325930162));
#132540=CARTESIAN_POINT('Ctrl Pts',(23.1056039194408,1.51414693370333,-7.15960182857439));
#132541=CARTESIAN_POINT('Ctrl Pts',(23.1076023427295,1.50960817985568,-7.15993090804821));
#132542=CARTESIAN_POINT('Ctrl Pts',(23.1095739866974,1.50505718142626,-7.16026042382627));
#132543=CARTESIAN_POINT('Ctrl Pts',(23.1292807058241,1.45956963435734,-7.16355395703598));
#132544=CARTESIAN_POINT('Ctrl Pts',(23.1463121274894,1.41285302083312,-7.16689052733892));
#132545=CARTESIAN_POINT('Ctrl Pts',(23.160555635742,1.36525587302037,-7.17021137308667));
#132546=CARTESIAN_POINT('Ctrl Pts',(23.1747858651263,1.3177030988439,-7.17352912289258));
#132547=CARTESIAN_POINT('Ctrl Pts',(23.1862336914812,1.26927145254509,-7.17683088390998));
#132548=CARTESIAN_POINT('Ctrl Pts',(23.1948245979885,1.22031254384211,-7.18007946634394));
#132549=CARTESIAN_POINT('Ctrl Pts',(23.2034110807242,1.17137884587059,-7.18332637596407));
#132550=CARTESIAN_POINT('Ctrl Pts',(23.2091436674003,1.12191842475156,-7.18652006664586));
#132551=CARTESIAN_POINT('Ctrl Pts',(23.2119828137938,1.07228635432059,-7.18964763895261));
#132552=CARTESIAN_POINT('Ctrl Pts',(23.2149708425993,1.02005162050749,-7.19293921847983));
#132553=CARTESIAN_POINT('Ctrl Pts',(23.2147535520184,0.967626754614273,
-7.19615738227058));
#132554=CARTESIAN_POINT('Ctrl Pts',(23.2113267459532,0.915430297146576,
-7.19931644801464));
#132555=CARTESIAN_POINT('Ctrl Pts',(23.2080678248899,0.86579103205804,-7.20232074580628));
#132556=CARTESIAN_POINT('Ctrl Pts',(23.201906219855,0.816358453725433,-7.20527201699764));
#132557=CARTESIAN_POINT('Ctrl Pts',(23.1928771501315,0.767495764724232,
-7.20820583271065));
#132558=CARTESIAN_POINT('Ctrl Pts',(23.1838426076001,0.71860345848436,-7.21114142670319));
#132559=CARTESIAN_POINT('Ctrl Pts',(23.1719366878453,0.670281923275512,
-7.2140599568284));
#132560=CARTESIAN_POINT('Ctrl Pts',(23.1572378379234,0.62289622656633,-7.21701512218833));
#132561=CARTESIAN_POINT('Ctrl Pts',(23.1436658154371,0.579143161212322,
-7.21974374183739));
#132562=CARTESIAN_POINT('Ctrl Pts',(23.1277123164478,0.536187580615072,
-7.22250418228607));
#132563=CARTESIAN_POINT('Ctrl Pts',(23.1094786702379,0.494316340902381,
-7.22534646665043));
#132564=CARTESIAN_POINT('Ctrl Pts',(23.1079321580124,0.490764973097593,
-7.22558753897723));
#132565=CARTESIAN_POINT('Ctrl Pts',(23.1063692490606,0.487221375408037,
-7.22582920007457));
#132566=CARTESIAN_POINT('Ctrl Pts',(23.1047900082331,0.483685705815835,
-7.22607148046424));
#132567=CARTESIAN_POINT('Ctrl Pts',(23.101740083699,0.476857408797344,-7.22653938687329));
#132568=CARTESIAN_POINT('Ctrl Pts',(23.0986293235844,0.470058800527314,
-7.22700960902506));
#132569=CARTESIAN_POINT('Ctrl Pts',(23.0954582895556,0.46329111275518,-7.22748236882627));
#132570=CARTESIAN_POINT('Ctrl Pts',(23.0954511030209,0.463275775101049,
-7.22748344024484));
#132571=CARTESIAN_POINT('Ctrl Pts',(23.0954439161766,0.463260437605711,
-7.22748451167644));
#132572=CARTESIAN_POINT('Ctrl Pts',(23.0954367290228,0.463245100269174,
-7.22748558312107));
#132573=CARTESIAN_POINT('Ctrl Pts',(23.0759885435365,0.421742807111391,
-7.23038487461292));
#132574=CARTESIAN_POINT('Ctrl Pts',(23.0541955748594,0.381254633016138,
-7.2333870240812));
#132575=CARTESIAN_POINT('Ctrl Pts',(23.0302100424038,0.342038699230848,
-7.2364330315869));
#132576=CARTESIAN_POINT('Ctrl Pts',(23.0282976945341,0.338912043294594,
-7.23667588739907));
#132577=CARTESIAN_POINT('Ctrl Pts',(23.0263714334915,0.335793487179436,
-7.23691902200578));
#132578=CARTESIAN_POINT('Ctrl Pts',(23.0244313492434,0.332683167846775,
-7.23716240550476));
#132579=CARTESIAN_POINT('Ctrl Pts',(22.9981951656695,0.29062163929907,-7.24045373378824));
#132580=CARTESIAN_POINT('Ctrl Pts',(22.9694263119232,0.250063447762252,
-7.24378997834366));
#132581=CARTESIAN_POINT('Ctrl Pts',(22.9383478845116,0.211299474319808,
-7.24711185102367));
#132582=CARTESIAN_POINT('Ctrl Pts',(22.9073006248753,0.172574376294066,
-7.25043039228088));
#132583=CARTESIAN_POINT('Ctrl Pts',(22.8739486232003,0.13563964686214,-7.25373429046647));
#132584=CARTESIAN_POINT('Ctrl Pts',(22.8385390936182,0.100756320054096,
-7.25698571893782));
#132585=CARTESIAN_POINT('Ctrl Pts',(22.8031397311405,0.0658830092623621,
-7.26023621382961));
#132586=CARTESIAN_POINT('Ctrl Pts',(22.7656840675728,0.0330598495998048,
-7.26343416853049));
#132587=CARTESIAN_POINT('Ctrl Pts',(22.7264421556169,0.00252111828283075,
-7.26656599894528));
#132588=CARTESIAN_POINT('Ctrl Pts',(22.6872079281136,-0.0280116328608765,
-7.26969721607694));
#132589=CARTESIAN_POINT('Ctrl Pts',(22.6461881210261,-0.0562607641338967,
-7.27276238169854));
#132590=CARTESIAN_POINT('Ctrl Pts',(22.6036756059344,-0.082018775347772,
-7.27577250159465));
#132591=CARTESIAN_POINT('Ctrl Pts',(22.5611291330222,-0.107797361348121,
-7.27878502589123));
#132592=CARTESIAN_POINT('Ctrl Pts',(22.5170874833382,-0.13108059782982,
-7.28174260914648));
#132593=CARTESIAN_POINT('Ctrl Pts',(22.4718681260937,-0.151689667592821,
-7.28467914380461));
#132594=CARTESIAN_POINT('Ctrl Pts',(22.4451788861354,-0.163853493921597,
-7.28641233690846));
#132595=CARTESIAN_POINT('Ctrl Pts',(22.4180798423309,-0.175086317613026,
-7.28813862593899));
#132596=CARTESIAN_POINT('Ctrl Pts',(22.3906403691454,-0.185356836028299,
-7.28986813301021));
#132597=CARTESIAN_POINT('Ctrl Pts',(22.3906127227906,-0.185251306681596,
-7.15421791561113));
#132598=CARTESIAN_POINT('Ctrl Pts',(22.3963865089124,-0.183104923268248,
-7.15381305253448));
#132599=CARTESIAN_POINT('Ctrl Pts',(22.4021446040177,-0.180916353269807,
-7.15340651779141));
#132600=CARTESIAN_POINT('Ctrl Pts',(22.4974886487836,-0.143877849688105,
-7.1466312728536));
#132601=CARTESIAN_POINT('Ctrl Pts',(22.5828282425092,-0.0989673465778473,
-7.13995318145344));
#132602=CARTESIAN_POINT('Ctrl Pts',(22.7055482856947,-0.0153089157280206,
-7.12993909527289));
#132603=CARTESIAN_POINT('Ctrl Pts',(22.7469681914671,0.0168681629758805,
-7.12646807965307));
#132604=CARTESIAN_POINT('Ctrl Pts',(22.8082537735905,0.0709040978539566,
-7.12119935494327));
#132605=CARTESIAN_POINT('Ctrl Pts',(22.8295525623377,0.0910411210818873,
-7.11933950438369));
#132606=CARTESIAN_POINT('Ctrl Pts',(22.871585102151,0.133643274251094,-7.11560107051006));
#132607=CARTESIAN_POINT('Ctrl Pts',(22.8922427104079,0.15615642476928,-7.11372630343523));
#132608=CARTESIAN_POINT('Ctrl Pts',(22.9574869606839,0.232648087821485,
-7.10764917212118));
#132609=CARTESIAN_POINT('Ctrl Pts',(22.9984101846094,0.289580172405581,
-7.10358548663138));
#132610=CARTESIAN_POINT('Ctrl Pts',(23.072345242098,0.412854521249262,-7.09529103843624));
#132611=CARTESIAN_POINT('Ctrl Pts',(23.1046673072505,0.479288879500483,
-7.09107723958861));
#132612=CARTESIAN_POINT('Ctrl Pts',(23.1389392649683,0.56886719174341,-7.08529140007046));
#132613=CARTESIAN_POINT('Ctrl Pts',(23.1463173960146,0.589784659058625,
-7.08393279762197));
#132614=CARTESIAN_POINT('Ctrl Pts',(23.158206153192,0.626544511255371,-7.08151495742629));
#132615=CARTESIAN_POINT('Ctrl Pts',(23.1629640934315,0.642300241452674,
-7.08046809863432));
#132616=CARTESIAN_POINT('Ctrl Pts',(23.1749718169935,0.685061957637121,
-7.07760142930103));
#132617=CARTESIAN_POINT('Ctrl Pts',(23.1816351708149,0.712221459791249,
-7.07575535289521));
#132618=CARTESIAN_POINT('Ctrl Pts',(23.203857975858,0.817812575233972,-7.06853396277475));
#132619=CARTESIAN_POINT('Ctrl Pts',(23.2128665995165,0.897432126960158,
-7.0630090361043));
#132620=CARTESIAN_POINT('Ctrl Pts',(23.215019269856,1.01769492812765,-7.05486999779951));
#132621=CARTESIAN_POINT('Ctrl Pts',(23.2138114256659,1.05803438076521,-7.05217190181311));
#132622=CARTESIAN_POINT('Ctrl Pts',(23.2079990946158,1.13261433088414,-7.04725922220962));
#132623=CARTESIAN_POINT('Ctrl Pts',(23.2039167964405,1.1668571285292,-7.04503324036443));
#132624=CARTESIAN_POINT('Ctrl Pts',(23.1939624687753,1.22871782296008,-7.04106150457622));
#132625=CARTESIAN_POINT('Ctrl Pts',(23.1885558222564,1.25638668499816,-7.03930323746905));
#132626=CARTESIAN_POINT('Ctrl Pts',(23.1734549661269,1.32194059829662,-7.0351692499306));
#132627=CARTESIAN_POINT('Ctrl Pts',(23.1629196905066,1.35960261735808,-7.03282040298909));
#132628=CARTESIAN_POINT('Ctrl Pts',(23.1223165566055,1.48248658654174,-7.0251667183367));
#132629=CARTESIAN_POINT('Ctrl Pts',(23.0848703744882,1.56496751080769,-7.02006338298117));
#132630=CARTESIAN_POINT('Ctrl Pts',(23.018098585617,1.67809252021458,-7.01239182177738));
#132631=CARTESIAN_POINT('Ctrl Pts',(22.99553433456,1.71239133048874,-7.00996088770126));
#132632=CARTESIAN_POINT('Ctrl Pts',(22.9608713578482,1.75987821054881,-7.00635347643586));
#132633=CARTESIAN_POINT('Ctrl Pts',(22.9500967330442,1.77400404954302,-7.00524755386539));
#132634=CARTESIAN_POINT('Ctrl Pts',(22.9273605293499,1.80254424848222,-7.00293425551295));
#132635=CARTESIAN_POINT('Ctrl Pts',(22.9153693172436,1.81692892310139,-7.00172542550888));
#132636=CARTESIAN_POINT('Ctrl Pts',(22.866589267801,1.87287141437836,-6.99686839863679));
#132637=CARTESIAN_POINT('Ctrl Pts',(22.8274031403086,1.91225166181806,-6.99309977126369));
#132638=CARTESIAN_POINT('Ctrl Pts',(22.7131658491625,2.01286537602583,-6.98271086244623));
#132639=CARTESIAN_POINT('Ctrl Pts',(22.6334605288347,2.06827231163822,-6.97611228950282));
#132640=CARTESIAN_POINT('Ctrl Pts',(22.5213521311855,2.12847068837013,-6.96785931357987));
#132641=CARTESIAN_POINT('Ctrl Pts',(22.4939830176899,2.14191596731054,-6.96591374833515));
#132642=CARTESIAN_POINT('Ctrl Pts',(22.4393668850518,2.16633666194278,-6.96215815956609));
#132643=CARTESIAN_POINT('Ctrl Pts',(22.4121708293295,2.17737822759954,-6.96034692672753));
#132644=CARTESIAN_POINT('Ctrl Pts',(22.3349542145218,2.20563961126037,-6.95534762334885));
#132645=CARTESIAN_POINT('Ctrl Pts',(22.2842010377944,2.22068304692898,-6.95222759534592));
#132646=CARTESIAN_POINT('Ctrl Pts',(22.1371485266208,2.25440663767665,-6.94345124070746));
#132647=CARTESIAN_POINT('Ctrl Pts',(22.0394357345041,2.26513154795565,-6.93794718681885));
#132648=CARTESIAN_POINT('Ctrl Pts',(21.9199669069424,2.26432629184898,-6.93072511192586));
#132649=CARTESIAN_POINT('Ctrl Pts',(21.8984654055484,2.26363247000938,-6.92940483284868));
#132650=CARTESIAN_POINT('Ctrl Pts',(21.8604483318462,2.26143387185808,-6.92701816159079));
#132651=CARTESIAN_POINT('Ctrl Pts',(21.8439259107583,2.26015201157404,-6.92596228362889));
#132652=CARTESIAN_POINT('Ctrl Pts',(21.7982629451956,2.25570504719778,-6.92299679427486));
#132653=CARTESIAN_POINT('Ctrl Pts',(21.7692012973077,2.25185097393195,-6.92105736487237));
#132654=CARTESIAN_POINT('Ctrl Pts',(21.696613600545,2.23964441021518,-6.9161212406612));
#132655=CARTESIAN_POINT('Ctrl Pts',(21.6533428573753,2.23000698680476,-6.91309542446328));
#132656=CARTESIAN_POINT('Ctrl Pts',(21.5317557998315,2.19613651961983,-6.90447520369459));
#132657=CARTESIAN_POINT('Ctrl Pts',(21.4551553100821,2.16653458018866,-6.89891502349031));
#132658=CARTESIAN_POINT('Ctrl Pts',(21.3536001712636,2.11547050081701,-6.89150827998112));
#132659=CARTESIAN_POINT('Ctrl Pts',(21.3257951654428,2.10015262423619,-6.88947397030077));
#132660=CARTESIAN_POINT('Ctrl Pts',(21.2739805442903,2.06901012222855,-6.8856647425911));
#132661=CARTESIAN_POINT('Ctrl Pts',(21.2498769318876,2.05338161859388,-6.88388462258408));
#132662=CARTESIAN_POINT('Ctrl Pts',(21.1887028702218,2.01068875622358,-6.8793296808101));
#132663=CARTESIAN_POINT('Ctrl Pts',(21.1525354679066,1.98240317723918,-6.87660049088308));
#132664=CARTESIAN_POINT('Ctrl Pts',(21.0660967739793,1.90687536981503,-6.86987776175335));
#132665=CARTESIAN_POINT('Ctrl Pts',(21.0180038698156,1.85737451268228,-6.86595206847186));
#132666=CARTESIAN_POINT('Ctrl Pts',(20.9445941419729,1.76829934022167,-6.85924854932783));
#132667=CARTESIAN_POINT('Ctrl Pts',(20.9170119033821,1.73079383200894,-6.85651503189649));
#132668=CARTESIAN_POINT('Ctrl Pts',(20.8812538929564,1.67608944724294,-6.85252525943183));
#132669=CARTESIAN_POINT('Ctrl Pts',(20.8713009601347,1.66009353286491,-6.85135820117931));
#132670=CARTESIAN_POINT('Ctrl Pts',(20.8527068172351,1.6286657019775,-6.8490526053752));
#132671=CARTESIAN_POINT('Ctrl Pts',(20.8440248971968,1.61326328403275,-6.8479165160438));
#132672=CARTESIAN_POINT('Ctrl Pts',(20.8166975525861,1.56231390591735,-6.84415034578213));
#132673=CARTESIAN_POINT('Ctrl Pts',(20.7994221081287,1.52606210176704,-6.84145871909278));
#132674=CARTESIAN_POINT('Ctrl Pts',(20.7509371966222,1.41045475984126,-6.83295770041728));
#132675=CARTESIAN_POINT('Ctrl Pts',(20.7260013998426,1.32871605246627,-6.82708106795391));
#132676=CARTESIAN_POINT('Ctrl Pts',(20.7012940701894,1.20365947452558,-6.8185858665388));
#132677=CARTESIAN_POINT('Ctrl Pts',(20.6951888115559,1.16184306796678,-6.8158209408496));
#132678=CARTESIAN_POINT('Ctrl Pts',(20.6884970714627,1.09152628403947,-6.81129810265361));
#132679=CARTESIAN_POINT('Ctrl Pts',(20.6867596803886,1.06317272302595,-6.80950804890915));
#132680=CARTESIAN_POINT('Ctrl Pts',(20.6850738156102,1.00190778767717,-6.80570397500247));
#132681=CARTESIAN_POINT('Ctrl Pts',(20.685451990105,0.969008127792423,-6.80370086054496));
#132682=CARTESIAN_POINT('Ctrl Pts',(20.6889935345336,0.898950803247316,
-6.79949479316228));
#132683=CARTESIAN_POINT('Ctrl Pts',(20.6925179295186,0.861842986321424,
-6.7973028541908));
#132684=CARTESIAN_POINT('Ctrl Pts',(20.7104488830827,0.733568411109644,
-6.78976070684839));
#132685=CARTESIAN_POINT('Ctrl Pts',(20.7331824769302,0.643874770766013,
-6.78456552064773));
#132686=CARTESIAN_POINT('Ctrl Pts',(20.7743138370979,0.533779686459548,
-6.77753390829196));
#132687=CARTESIAN_POINT('Ctrl Pts',(20.7838683191025,0.51037151850517,-6.77599745183441));
#132688=CARTESIAN_POINT('Ctrl Pts',(20.8007334967601,0.472351385461223,
-6.77340899431203));
#132689=CARTESIAN_POINT('Ctrl Pts',(20.8076369258322,0.457567420316831,
-6.77237783259001));
#132690=CARTESIAN_POINT('Ctrl Pts',(20.8254131762144,0.421344301150035,
-6.7697876802359));
#132691=CARTESIAN_POINT('Ctrl Pts',(20.836613790816,0.400075902066019,-6.76821255840321));
#132692=CARTESIAN_POINT('Ctrl Pts',(20.8641128378357,0.351284455593395,
-6.76449142200549));
#132693=CARTESIAN_POINT('Ctrl Pts',(20.8808632207748,0.32403467279011,-6.76233025450739));
#132694=CARTESIAN_POINT('Ctrl Pts',(20.9474008643691,0.224460394373303,
-6.7541831645393));
#132695=CARTESIAN_POINT('Ctrl Pts',(21.0036489697528,0.156738807302235,
-6.74814774155795));
#132696=CARTESIAN_POINT('Ctrl Pts',(21.0933645015358,0.0691133248970699,
-6.73985523634111));
#132697=CARTESIAN_POINT('Ctrl Pts',(21.1214269165456,0.0440494411410075,
-6.73741120008417));
#132698=CARTESIAN_POINT('Ctrl Pts',(21.1723565606275,0.00249218114765082,
-6.73322401034571));
#132699=CARTESIAN_POINT('Ctrl Pts',(21.1947341116024,-0.0145564527277919,
-6.73146054951477));
#132700=CARTESIAN_POINT('Ctrl Pts',(21.2466254174067,-0.0514212512889634,
-6.72752940875522));
#132701=CARTESIAN_POINT('Ctrl Pts',(21.2764436592025,-0.0707682455996173,
-6.72537950856607));
#132702=CARTESIAN_POINT('Ctrl Pts',(21.3436034248488,-0.110426309120024,
-6.72073426415478));
#132703=CARTESIAN_POINT('Ctrl Pts',(21.38123348881,-0.130162987160132,-6.71825671179315));
#132704=CARTESIAN_POINT('Ctrl Pts',(21.4924773583885,-0.181543219386842,
-6.71116278146636));
#132705=CARTESIAN_POINT('Ctrl Pts',(21.5681861558721,-0.208133907758561,
-6.70661885548462));
#132706=CARTESIAN_POINT('Ctrl Pts',(21.6703019322688,-0.233434882759522,
-6.70032254202073));
#132707=CARTESIAN_POINT('Ctrl Pts',(21.694883819683,-0.238752666230422,
-6.69879366072573));
#132708=CARTESIAN_POINT('Ctrl Pts',(21.7356526564801,-0.246307270359711,
-6.69621274823031));
#132709=CARTESIAN_POINT('Ctrl Pts',(21.7517528162549,-0.248969410577584,
-6.6951811815374));
#132710=CARTESIAN_POINT('Ctrl Pts',(21.7918239997672,-0.254800802836197,
-6.69258130711573));
#132711=CARTESIAN_POINT('Ctrl Pts',(21.8158405486243,-0.25759523402539,
-6.69099652089502));
#132712=CARTESIAN_POINT('Ctrl Pts',(21.8720660704988,-0.262508526584901,
-6.68724567675781));
#132713=CARTESIAN_POINT('Ctrl Pts',(21.9043057432556,-0.264085953687192,
-6.68506416753593));
#132714=CARTESIAN_POINT('Ctrl Pts',(22.0243936500095,-0.265361582990704,
-6.67689295696047));
#132715=CARTESIAN_POINT('Ctrl Pts',(22.1120879124508,-0.257141564761878,
-6.67085666184916));
#132716=CARTESIAN_POINT('Ctrl Pts',(22.2348177933554,-0.232571167358713,
-6.66258516992038));
#132717=CARTESIAN_POINT('Ctrl Pts',(22.2710698533072,-0.223628801507223,
-6.66016111164593));
#132718=CARTESIAN_POINT('Ctrl Pts',(22.3338561783121,-0.205157907870959,
-6.65599388783242));
#132719=CARTESIAN_POINT('Ctrl Pts',(22.3605652756198,-0.196322487082332,
-6.65423114745454));
#132720=CARTESIAN_POINT('Ctrl Pts',(22.3881777505251,-0.186154364635265,
-6.65241463787186));
#132721=CARTESIAN_POINT('Ctrl Pts',(22.3893955932103,-0.185703770054698,
-6.65233453257165));
#132722=CARTESIAN_POINT('Ctrl Pts',(22.3906127229569,-0.185251306619802,
-6.65225448505536));
#132723=CARTESIAN_POINT('Origin',(21.9499999789786,0.999999999999992,-6.00000000000001));
#132724=CARTESIAN_POINT('',(22.3906127230461,-0.185251306586623,-6.15441073460198));
#132725=CARTESIAN_POINT('',(22.3906686070801,-0.185465307370993,-6.2896766972819));
#132726=CARTESIAN_POINT('',(22.3906127231008,-0.185251306566283,-6.00000000000001));
#132727=CARTESIAN_POINT('',(22.908116131701,1.82521129893649,-6.00000000000001));
#132728=CARTESIAN_POINT('Ctrl Pts',(22.3906127229914,-0.185251306606962,
-6.15441073460198));
#132729=CARTESIAN_POINT('Ctrl Pts',(22.4057011923799,-0.179642224496554,
-6.15337585754839));
#132730=CARTESIAN_POINT('Ctrl Pts',(22.4206806463947,-0.173745732741962,
-6.15232558575311));
#132731=CARTESIAN_POINT('Ctrl Pts',(22.4576526446442,-0.158370580821461,
-6.14968303259365));
#132732=CARTESIAN_POINT('Ctrl Pts',(22.4794955608251,-0.148550359902258,
-6.1480767831395));
#132733=CARTESIAN_POINT('Ctrl Pts',(22.5513072346985,-0.113781092920369,
-6.14267246581676));
#132734=CARTESIAN_POINT('Ctrl Pts',(22.5999008878328,-0.0861433318381266,
-6.13881400970775));
#132735=CARTESIAN_POINT('Ctrl Pts',(22.7063613905894,-0.015884069010359,
-6.13006915257598));
#132736=CARTESIAN_POINT('Ctrl Pts',(22.7627535715962,0.0286415226550085,
-6.12522290339564));
#132737=CARTESIAN_POINT('Ctrl Pts',(22.8368763351462,0.0981661737317596,
-6.11860992756174));
#132738=CARTESIAN_POINT('Ctrl Pts',(22.8579495235599,0.119385561944241,
-6.11669608585324));
#132739=CARTESIAN_POINT('Ctrl Pts',(22.8970511659868,0.161655977368502,
-6.11307156243022));
#132740=CARTESIAN_POINT('Ctrl Pts',(22.9151786762439,0.18259134058388,-6.11135729054517));
#132741=CARTESIAN_POINT('Ctrl Pts',(22.9607684632705,0.238876208560583,
-6.10693888225787));
#132742=CARTESIAN_POINT('Ctrl Pts',(22.9870677755454,0.275118416270965,
-6.10427981671326));
#132743=CARTESIAN_POINT('Ctrl Pts',(23.0478711257816,0.369014067598781,
-6.09773532268297));
#132744=CARTESIAN_POINT('Ctrl Pts',(23.0798069369696,0.428160380031941,
-6.09391526460624));
#132745=CARTESIAN_POINT('Ctrl Pts',(23.1259659390328,0.532778844877155,
-6.08728611650922));
#132746=CARTESIAN_POINT('Ctrl Pts',(23.1425955202437,0.577026498993845,
-6.08451587356466));
#132747=CARTESIAN_POINT('Ctrl Pts',(23.1622512866886,0.639790576151933,
-6.08050092457355));
#132748=CARTESIAN_POINT('Ctrl Pts',(23.1674025017133,0.657603928892554,
-6.07935201345799));
#132749=CARTESIAN_POINT('Ctrl Pts',(23.1766212926487,0.692326984305418,
-6.07708267067493));
#132750=CARTESIAN_POINT('Ctrl Pts',(23.1807353231366,0.709220090239246,
-6.07596501277343));
#132751=CARTESIAN_POINT('Ctrl Pts',(23.1922838535727,0.761288044280355,
-6.07248866640026));
#132752=CARTESIAN_POINT('Ctrl Pts',(23.1985673161203,0.796697812072016,
-6.07008113187139));
#132753=CARTESIAN_POINT('Ctrl Pts',(23.2116825207765,0.894730342318195,
-6.06336937998488));
#132754=CARTESIAN_POINT('Ctrl Pts',(23.2153587510691,0.957672476655,-6.05901261864392));
#132755=CARTESIAN_POINT('Ctrl Pts',(23.2131961310744,1.09023716025245,-6.04994062542701));
#132756=CARTESIAN_POINT('Ctrl Pts',(23.2063134732515,1.15964331065296,-6.04525385919441));
#132757=CARTESIAN_POINT('Ctrl Pts',(23.1877691925515,1.26074208526004,-6.03856247798658));
#132758=CARTESIAN_POINT('Ctrl Pts',(23.1805085603149,1.29310064875821,-6.03644018423112));
#132759=CARTESIAN_POINT('Ctrl Pts',(23.1635107776574,1.356984199452,-6.0322773043734));
#132760=CARTESIAN_POINT('Ctrl Pts',(23.1537954632829,1.38848792858206,-6.03023791503399));
#132761=CARTESIAN_POINT('Ctrl Pts',(23.1310276328374,1.45321682865112,-6.02605223181921));
#132762=CARTESIAN_POINT('Ctrl Pts',(23.1177774201401,1.48634133539319,-6.02391286682768));
#132763=CARTESIAN_POINT('Ctrl Pts',(23.0616144632079,1.61116036503629,-6.01577950387353));
#132764=CARTESIAN_POINT('Ctrl Pts',(23.0091579730641,1.69812949140097,-6.00997918615594));
#132765=CARTESIAN_POINT('Ctrl Pts',(22.9343556261016,1.79399011384819,-6.00254541175663));
#132766=CARTESIAN_POINT('Ctrl Pts',(22.9214265697249,1.80975714108992,-6.00128356337885));
#132767=CARTESIAN_POINT('Ctrl Pts',(22.9081161317008,1.82521129893667,-6.));
#132768=CARTESIAN_POINT('',(20.9988875029867,1.83390743487766,-6.00000965788105));
#132769=CARTESIAN_POINT('Origin',(21.9499999789786,0.999999999999992,-6.00000000000001));
#132770=CARTESIAN_POINT('Ctrl Pts',(20.9988875029867,1.83390743487766,-6.00000965788105));
#132771=CARTESIAN_POINT('Ctrl Pts',(21.0286901916504,1.86779465086861,-6.00298051266928));
#132772=CARTESIAN_POINT('Ctrl Pts',(21.0603844609322,1.90012375983217,-6.00600667165696));
#132773=CARTESIAN_POINT('Ctrl Pts',(21.09376706437,1.9306946394671,-6.00903840021643));
#132774=CARTESIAN_POINT('Ctrl Pts',(21.1299596154473,1.96383879267031,-6.01232532152996));
#132775=CARTESIAN_POINT('Ctrl Pts',(21.1681370950843,1.99491683397022,-6.01561839937007));
#132776=CARTESIAN_POINT('Ctrl Pts',(21.2080211602335,2.02370881328864,-6.01887262241129));
#132777=CARTESIAN_POINT('Ctrl Pts',(21.2478716347671,2.0524765438174,-6.022124104725));
#132778=CARTESIAN_POINT('Ctrl Pts',(21.2894257342513,2.0789621813169,-6.0253366302436));
#132779=CARTESIAN_POINT('Ctrl Pts',(21.3323868181518,2.10297735669125,-6.02848774538209));
#132780=CARTESIAN_POINT('Ctrl Pts',(21.3753306942387,2.12698291292599,-6.03163759835963));
#132781=CARTESIAN_POINT('Ctrl Pts',(21.4196803982476,2.1485199368721,-6.03472607855688));
#132782=CARTESIAN_POINT('Ctrl Pts',(21.46512147125,2.16743080065149,-6.03775449719176));
#132783=CARTESIAN_POINT('Ctrl Pts',(21.5105945642123,2.18635498993266,-6.04078504979568));
#132784=CARTESIAN_POINT('Ctrl Pts',(21.5571605595361,2.20264911447047,-6.04375558047421));
#132785=CARTESIAN_POINT('Ctrl Pts',(21.6044863659149,2.2161876712167,-6.04669034846989));
#132786=CARTESIAN_POINT('Ctrl Pts',(21.6518292233586,2.22973110578392,-6.04962617383625));
#132787=CARTESIAN_POINT('Ctrl Pts',(21.6999324250985,2.24051662077448,-6.05252650726871));
#132788=CARTESIAN_POINT('Ctrl Pts',(21.7484446496936,2.2484552726454,-6.05543547749697));
#132789=CARTESIAN_POINT('Ctrl Pts',(21.7970413041404,2.25640774081118,-6.05834951044759));
#132790=CARTESIAN_POINT('Ctrl Pts',(21.8460482988538,2.26150284578719,-6.06127273889257));
#132791=CARTESIAN_POINT('Ctrl Pts',(21.8950953201096,2.26369509549222,-6.06426330924486));
#132792=CARTESIAN_POINT('Ctrl Pts',(21.9256270201211,2.26505976777263,-6.0661249349771));
#132793=CARTESIAN_POINT('Ctrl Pts',(21.9561738762397,2.2653004590272,-6.06801291925003));
#132794=CARTESIAN_POINT('Ctrl Pts',(21.986643756937,2.26441650318461,-6.06994229671044));
#132795=CARTESIAN_POINT('Ctrl Pts',(21.986660132454,2.26441602811763,-6.06994333362141));
#132796=CARTESIAN_POINT('Ctrl Pts',(21.9866765079491,2.264415552726,-6.06994437054433));
#132797=CARTESIAN_POINT('Ctrl Pts',(21.9866928834221,2.26441507700973,-6.06994540747922));
#132798=CARTESIAN_POINT('Ctrl Pts',(22.0326809237129,2.2630790997727,-6.07285748232858));
#132799=CARTESIAN_POINT('Ctrl Pts',(22.0786682668699,2.25916991357468,-6.07587157755844));
#132800=CARTESIAN_POINT('Ctrl Pts',(22.1243556678835,2.25272547701368,-6.07892867334182));
#132801=CARTESIAN_POINT('Ctrl Pts',(22.1291582634149,2.2520480468788,-6.07925003096389));
#132802=CARTESIAN_POINT('Ctrl Pts',(22.133957507768,2.25134263235827,-6.07957186373863));
#132803=CARTESIAN_POINT('Ctrl Pts',(22.1387530280941,2.25060929931715,-6.07989410311142));
#132804=CARTESIAN_POINT('Ctrl Pts',(22.1878297144056,2.24310447123295,-6.08319185591832));
#132805=CARTESIAN_POINT('Ctrl Pts',(22.2365212677171,2.23267260072574,-6.08653164154161));
#132806=CARTESIAN_POINT('Ctrl Pts',(22.2844718942759,2.21940438098023,-6.08985504759089));
#132807=CARTESIAN_POINT('Ctrl Pts',(22.3323791486108,2.20614816258353,-6.09317544755826));
#132808=CARTESIAN_POINT('Ctrl Pts',(22.3795469665926,2.19006100091275,-6.09647920494974));
#132809=CARTESIAN_POINT('Ctrl Pts',(22.4256372421703,2.17126745842227,-6.09972950322665));
#132810=CARTESIAN_POINT('Ctrl Pts',(22.4717048879636,2.15248314334057,-6.10297820564525));
#132811=CARTESIAN_POINT('Ctrl Pts',(22.516696097646,2.13099517083427,-6.10617340736871));
#132812=CARTESIAN_POINT('Ctrl Pts',(22.5602884459666,2.10695954641308,-6.1093025953749));
#132813=CARTESIAN_POINT('Ctrl Pts',(22.6060509761539,2.08172734327377,-6.11258756546968));
#132814=CARTESIAN_POINT('Ctrl Pts',(22.6502716692536,2.05368713042489,-6.11579961957646));
#132815=CARTESIAN_POINT('Ctrl Pts',(22.6925957272256,2.02305700606354,-6.11895337160971));
#132816=CARTESIAN_POINT('Ctrl Pts',(22.7329495418233,1.99385275631031,-6.12196031212854));
#132817=CARTESIAN_POINT('Ctrl Pts',(22.7715791222734,1.96229419772647,-6.12491466625996));
#132818=CARTESIAN_POINT('Ctrl Pts',(22.8081948530333,1.92860496734828,-6.1278522924454));
#132819=CARTESIAN_POINT('Ctrl Pts',(22.8448331350749,1.89489498809229,-6.13079172788697));
#132820=CARTESIAN_POINT('Ctrl Pts',(22.8794546905557,1.85905144030258,-6.1337148321294));
#132821=CARTESIAN_POINT('Ctrl Pts',(22.9117913162614,1.82133568321041,-6.13667550720105));
#132822=CARTESIAN_POINT('Ctrl Pts',(22.9415978529287,1.78657089028073,-6.13940453251391));
#132823=CARTESIAN_POINT('Ctrl Pts',(22.9694631685719,1.75021490169197,-6.14216607008642));
#132824=CARTESIAN_POINT('Ctrl Pts',(22.9951985991147,1.7125056088617,-6.14500991311024));
#132825=CARTESIAN_POINT('Ctrl Pts',(22.9974292928614,1.70923704556444,-6.1452564115257));
#132826=CARTESIAN_POINT('Ctrl Pts',(22.9996440150743,1.70595830355076,-6.1455035283072));
#132827=CARTESIAN_POINT('Ctrl Pts',(23.0018426600711,1.70266953085443,-6.14575129588088));
#132828=CARTESIAN_POINT('Ctrl Pts',(23.0057821587272,1.69677675797102,-6.14619524204998));
#132829=CARTESIAN_POINT('Ctrl Pts',(23.0096699883344,1.69085189810752,-6.14664128249749));
#132830=CARTESIAN_POINT('Ctrl Pts',(23.0135055153554,1.68489591262325,-6.14708960513326));
#132831=CARTESIAN_POINT('Ctrl Pts',(23.013514654098,1.68488172155684,-6.14709067333202));
#132832=CARTESIAN_POINT('Ctrl Pts',(23.0135237925438,1.68486753031373,-6.14709174154373));
#132833=CARTESIAN_POINT('Ctrl Pts',(23.0135329306927,1.68485333889393,-6.14709280976841));
#132834=CARTESIAN_POINT('Ctrl Pts',(23.0383604653831,1.64629651813792,-6.14999508084554));
#132835=CARTESIAN_POINT('Ctrl Pts',(23.0610808588401,1.60628993946131,-6.15300039228515));
#132836=CARTESIAN_POINT('Ctrl Pts',(23.0815561499041,1.56509966304113,-6.15604955149147));
#132837=CARTESIAN_POINT('Ctrl Pts',(23.0837750031228,1.56063598156621,-6.15637998082204));
#132838=CARTESIAN_POINT('Ctrl Pts',(23.0859674949999,1.55615844960958,-6.15671092507817));
#132839=CARTESIAN_POINT('Ctrl Pts',(23.0881334539325,1.55166744219402,-6.15704230893076));
#132840=CARTESIAN_POINT('Ctrl Pts',(23.1096475742327,1.50705899078141,-6.16033389122385));
#132841=CARTESIAN_POINT('Ctrl Pts',(23.1285441657354,1.46111522005574,-6.16366829876123));
#132842=CARTESIAN_POINT('Ctrl Pts',(23.1446964210521,1.41417901002546,-6.16698677355879));
#132843=CARTESIAN_POINT('Ctrl Pts',(23.1608334138497,1.36728715075519,-6.17030211267753));
#132844=CARTESIAN_POINT('Ctrl Pts',(23.1742315647608,1.31940476171366,-6.17360125719417));
#132845=CARTESIAN_POINT('Ctrl Pts',(23.1848019649728,1.27087942969894,-6.1768470231628));
#132846=CARTESIAN_POINT('Ctrl Pts',(23.195366813583,1.22237958331531,-6.18009108444666));
#132847=CARTESIAN_POINT('Ctrl Pts',(23.2031069616019,1.17323747086701,-6.18328172876644));
#132848=CARTESIAN_POINT('Ctrl Pts',(23.2079682928694,1.12380562289868,-6.18640604697854));
#132849=CARTESIAN_POINT('Ctrl Pts',(23.2128291111351,1.07437899132607,-6.18953003549064));
#132850=CARTESIAN_POINT('Ctrl Pts',(23.2148116257186,1.02466270822257,-6.19258776206157));
#132851=CARTESIAN_POINT('Ctrl Pts',(23.2138965373217,0.975014523593003,
-6.1955908500668));
#132852=CARTESIAN_POINT('Ctrl Pts',(23.2129805785505,0.925319116745311,
-6.19859679441971));
#132853=CARTESIAN_POINT('Ctrl Pts',(23.209161243197,0.875692002999865,-6.20154819210288));
#132854=CARTESIAN_POINT('Ctrl Pts',(23.2024566986069,0.826496664179489,
-6.20447946551915));
#132855=CARTESIAN_POINT('Ctrl Pts',(23.195748241031,0.777272613392309,-6.20741244971995));
#132856=CARTESIAN_POINT('Ctrl Pts',(23.1861507743226,0.728481007109299,
-6.21032568483769));
#132857=CARTESIAN_POINT('Ctrl Pts',(23.1737252053094,0.680489037516421,
-6.21327203773247));
#132858=CARTESIAN_POINT('Ctrl Pts',(23.1621874248703,0.635926023346594,
-6.21600787805978));
#132859=CARTESIAN_POINT('Ctrl Pts',(23.1482108799797,0.592052120796729,
-6.21877285073307));
#132860=CARTESIAN_POINT('Ctrl Pts',(23.1318842122252,0.549162471506275,
-6.22161761851486));
#132861=CARTESIAN_POINT('Ctrl Pts',(23.1305985213221,0.545785001421174,
-6.22184163802168));
#132862=CARTESIAN_POINT('Ctrl Pts',(23.1292982629967,0.542413608841275,
-6.22206615235655));
#132863=CARTESIAN_POINT('Ctrl Pts',(23.1279834833797,0.539048424415133,
-6.22229118625981));
#132864=CARTESIAN_POINT('Ctrl Pts',(23.124196597574,0.529355872924713,-6.22293933875854));
#132865=CARTESIAN_POINT('Ctrl Pts',(23.1202893850572,0.519715057120877,
-6.22359181589556));
#132866=CARTESIAN_POINT('Ctrl Pts',(23.1162632099014,0.510129357139251,
-6.22424921766053));
#132867=CARTESIAN_POINT('Ctrl Pts',(23.1162565869514,0.510113588920277,
-6.22425029906877));
#132868=CARTESIAN_POINT('Ctrl Pts',(23.1162499636796,0.510097820850403,
-6.22425138049034));
#132869=CARTESIAN_POINT('Ctrl Pts',(23.1162433400858,0.510082052929644,
-6.22425246192524));
#132870=CARTESIAN_POINT('Ctrl Pts',(23.0984965463045,0.467834588966754,
-6.22714998294805));
#132871=CARTESIAN_POINT('Ctrl Pts',(23.0783667308209,0.426505274501597,
-6.23015061953357));
#132872=CARTESIAN_POINT('Ctrl Pts',(23.0559954974735,0.386357985883809,
-6.23319539900638));
#132873=CARTESIAN_POINT('Ctrl Pts',(23.0542030444861,0.38314125990796,-6.23343935623384));
#132874=CARTESIAN_POINT('Ctrl Pts',(23.0523962263639,0.37993213579517,-6.23368359684601));
#132875=CARTESIAN_POINT('Ctrl Pts',(23.0505751287022,0.376730756018156,
-6.23392809050927));
#132876=CARTESIAN_POINT('Ctrl Pts',(23.0260598235902,0.333634329250968,
-6.23721942236857));
#132877=CARTESIAN_POINT('Ctrl Pts',(22.9989521667812,0.291938164542877,
-6.24055601012744));
#132878=CARTESIAN_POINT('Ctrl Pts',(22.9694634631529,0.251942012917784,
-6.24387848847534));
#132879=CARTESIAN_POINT('Ctrl Pts',(22.940003946175,0.211985447763226,-6.24719767837709));
#132880=CARTESIAN_POINT('Ctrl Pts',(22.9081683055633,0.173725286597264,
-6.25050248569246));
#132881=CARTESIAN_POINT('Ctrl Pts',(22.8741931459292,0.137432405205992,
-6.25375499851268));
#132882=CARTESIAN_POINT('Ctrl Pts',(22.8402243688189,0.101146341742298,
-6.25700690032059));
#132883=CARTESIAN_POINT('Ctrl Pts',(22.8041169244941,0.0668267464994518,
-6.26020642568044));
#132884=CARTESIAN_POINT('Ctrl Pts',(22.7661313802783,0.0347187356368984,
-6.26333990837154));
#132885=CARTESIAN_POINT('Ctrl Pts',(22.7281530948429,0.00261686039791348,
-6.2664727922753));
#132886=CARTESIAN_POINT('Ctrl Pts',(22.6882973927823,-0.0272741915223843,
-6.26953970530947));
#132887=CARTESIAN_POINT('Ctrl Pts',(22.6468487220025,-0.0547351490927038,
-6.27255159353335));
#132888=CARTESIAN_POINT('Ctrl Pts',(22.6053564963114,-0.0822249630666226,
-6.27556664669647));
#132889=CARTESIAN_POINT('Ctrl Pts',(22.562267857641,-0.107279327169208,
-6.27852675107654));
#132890=CARTESIAN_POINT('Ctrl Pts',(22.5178932287369,-0.129706502125296,
-6.2814657934101));
#132891=CARTESIAN_POINT('Ctrl Pts',(22.4765123176448,-0.150620636075763,
-6.28420655434724));
#132892=CARTESIAN_POINT('Ctrl Pts',(22.434013247025,-0.169250079969709,
-6.28692948158993));
#132893=CARTESIAN_POINT('Ctrl Pts',(22.3906686070801,-0.185465307370996,
-6.2896766972819));
#132894=CARTESIAN_POINT('Origin',(21.9499999789786,0.999999999999992,-4.89578827641128));
#132895=CARTESIAN_POINT('',(22.8894915957587,2.22401164291841,-7.78024830238043));
#132896=CARTESIAN_POINT('',(22.889491610182,2.22401163184779,-7.82252261963806));
#132897=CARTESIAN_POINT('',(22.8894916101512,2.22401163187148,-4.89578827641128));
#132898=CARTESIAN_POINT('',(22.3485138208359,-0.490649428218508,-8.00000000000001));
#132899=CARTESIAN_POINT('Ctrl Pts',(22.889491610182,2.22401163184779,-7.82252261963806));
#132900=CARTESIAN_POINT('Ctrl Pts',(22.8898635485898,2.22372615006616,-7.82254904469854));
#132901=CARTESIAN_POINT('Ctrl Pts',(22.8902353594378,2.22344049679263,-7.82257547297005));
#132902=CARTESIAN_POINT('Ctrl Pts',(22.9584420387731,2.17098949790154,-7.82742584661769));
#132903=CARTESIAN_POINT('Ctrl Pts',(23.0218183424636,2.11327304613071,-7.83235239300052));
#132904=CARTESIAN_POINT('Ctrl Pts',(23.1068674277578,2.02178972213453,-7.83935303997649));
#132905=CARTESIAN_POINT('Ctrl Pts',(23.1325426168569,1.99196261873962,-7.84152587714254));
#132906=CARTESIAN_POINT('Ctrl Pts',(23.1683716943707,1.94696864979136,-7.84461104845634));
#132907=CARTESIAN_POINT('Ctrl Pts',(23.1794407656144,1.93255277116917,-7.84557223559737));
#132908=CARTESIAN_POINT('Ctrl Pts',(23.2000218049921,1.90474530731534,-7.84736979107497));
#132909=CARTESIAN_POINT('Ctrl Pts',(23.2095790772173,1.89139168657683,-7.84820843300643));
#132910=CARTESIAN_POINT('Ctrl Pts',(23.2361293666813,1.85301520523579,-7.85055550327267));
#132911=CARTESIAN_POINT('Ctrl Pts',(23.2526030596146,1.82764072472637,-7.85203360653475));
#132912=CARTESIAN_POINT('Ctrl Pts',(23.2911235882287,1.76430495959742,-7.85558658151277));
#132913=CARTESIAN_POINT('Ctrl Pts',(23.3123173991765,1.72585549298537,-7.85762877496279));
#132914=CARTESIAN_POINT('Ctrl Pts',(23.3846576998291,1.58025425398773,-7.8651233531947));
#132915=CARTESIAN_POINT('Ctrl Pts',(23.4250265827451,1.46822364563206,-7.87046371008796));
#132916=CARTESIAN_POINT('Ctrl Pts',(23.4599090754759,1.31964723972354,-7.8778737839146));
#132917=CARTESIAN_POINT('Ctrl Pts',(23.4665712002994,1.28637624954946,-7.87955029503946));
#132918=CARTESIAN_POINT('Ctrl Pts',(23.4765429513912,1.22636255077981,-7.88261868401024));
#132919=CARTESIAN_POINT('Ctrl Pts',(23.4802590236487,1.19970125063584,-7.88399722774642));
#132920=CARTESIAN_POINT('Ctrl Pts',(23.4870124430072,1.13983186497366,-7.88713193073266));
#132921=CARTESIAN_POINT('Ctrl Pts',(23.4896744184964,1.10659578293834,-7.88889896610823));
#132922=CARTESIAN_POINT('Ctrl Pts',(23.4949036162639,0.996644662793407,
-7.89483554001359));
#132923=CARTESIAN_POINT('Ctrl Pts',(23.4928250647758,0.919830638399253,
-7.89913529926684));
#132924=CARTESIAN_POINT('Ctrl Pts',(23.4750586052286,0.745570115913723,
-7.90909402318625));
#132925=CARTESIAN_POINT('Ctrl Pts',(23.4557265847982,0.648820166733901,
-7.91477608861073));
#132926=CARTESIAN_POINT('Ctrl Pts',(23.4214552654331,0.535156542065498,
-7.92121807243912));
#132927=CARTESIAN_POINT('Ctrl Pts',(23.4152197841016,0.51586045315267,-7.92230257536467));
#132928=CARTESIAN_POINT('Ctrl Pts',(23.4033404750406,0.481433768169408,
-7.92421382447387));
#132929=CARTESIAN_POINT('Ctrl Pts',(23.397836830251,0.466260367432381,-7.92504717392675));
#132930=CARTESIAN_POINT('Ctrl Pts',(23.3831498789931,0.427668883517724,
-7.92714785785703));
#132931=CARTESIAN_POINT('Ctrl Pts',(23.3736303738123,0.40438420925236,-7.9283978513551));
#132932=CARTESIAN_POINT('Ctrl Pts',(23.3505507784266,0.351650659952187,
-7.93120874318343));
#132933=CARTESIAN_POINT('Ctrl Pts',(23.3366233219783,0.322375256239287,
-7.9327546230739));
#132934=CARTESIAN_POINT('Ctrl Pts',(23.279694037837,0.211828629361794,-7.93860553967999));
#132935=CARTESIAN_POINT('Ctrl Pts',(23.2303838546479,0.134021665293877,
-7.94276242087797));
#132936=CARTESIAN_POINT('Ctrl Pts',(23.1338177743768,0.00809238171863846,
-7.95015372417362));
#132937=CARTESIAN_POINT('Ctrl Pts',(23.0898044425818,-0.0421852376196696,
-7.95331877871642));
#132938=CARTESIAN_POINT('Ctrl Pts',(23.0183295296939,-0.113871633295997,
-7.95829426390745));
#132939=CARTESIAN_POINT('Ctrl Pts',(22.9931722255307,-0.137466264300778,
-7.96001769657505));
#132940=CARTESIAN_POINT('Ctrl Pts',(22.9434664337016,-0.181047686565909,
-7.9633821547244));
#132941=CARTESIAN_POINT('Ctrl Pts',(22.9190518222137,-0.201160936123177,
-7.96501734641841));
#132942=CARTESIAN_POINT('Ctrl Pts',(22.8545967442228,-0.251015550072751,
-7.96929485261125));
#132943=CARTESIAN_POINT('Ctrl Pts',(22.8137030758859,-0.279590405128052,
-7.97197238475304));
#132944=CARTESIAN_POINT('Ctrl Pts',(22.6679253088973,-0.371278140795948,
-7.98137216582847));
#132945=CARTESIAN_POINT('Ctrl Pts',(22.5569746768909,-0.423868254770818,
-7.98831317868678));
#132946=CARTESIAN_POINT('Ctrl Pts',(22.423651150773,-0.468617633822337,
-7.99588534263564));
#132947=CARTESIAN_POINT('Ctrl Pts',(22.4062179835011,-0.474126304133557,
-7.99686039556757));
#132948=CARTESIAN_POINT('Ctrl Pts',(22.3753503458647,-0.483280039559475,
-7.99855641085894));
#132949=CARTESIAN_POINT('Ctrl Pts',(22.3619568853333,-0.487055526676146,
-7.99928234965091));
#132950=CARTESIAN_POINT('Ctrl Pts',(22.3485138208359,-0.490649428218505,
-8.));
#132951=CARTESIAN_POINT('',(21.5504184355883,-0.491444307170665,-7.99938271504714));
#132952=CARTESIAN_POINT('Origin',(21.9499999789786,0.999999999999992,-8.00000000000001));
#132953=CARTESIAN_POINT('Ctrl Pts',(21.5507417872889,-0.49045023277154,
-7.99877818246404));
#132954=CARTESIAN_POINT('Ctrl Pts',(21.684483670055,-0.526276683794352,
-7.99205016521409));
#132955=CARTESIAN_POINT('Ctrl Pts',(21.8224480500903,-0.543942214410516,
-7.98592091362909));
#132956=CARTESIAN_POINT('Ctrl Pts',(22.0076445340552,-0.542630388429268,
-7.97709993740197));
#132957=CARTESIAN_POINT('Ctrl Pts',(22.0543175938958,-0.540178169116188,
-7.97483282718998));
#132958=CARTESIAN_POINT('Ctrl Pts',(22.1300476144749,-0.532741075226077,
-7.97104119923413));
#132959=CARTESIAN_POINT('Ctrl Pts',(22.1592005200333,-0.529034776397013,
-7.96955425248215));
#132960=CARTESIAN_POINT('Ctrl Pts',(22.2185250141901,-0.519764318499925,
-7.96646495803174));
#132961=CARTESIAN_POINT('Ctrl Pts',(22.2486719472076,-0.514128187063365,
-7.96486109129298));
#132962=CARTESIAN_POINT('Ctrl Pts',(22.3349526873501,-0.495320509388373,
-7.96016768204963));
#132963=CARTESIAN_POINT('Ctrl Pts',(22.3905386526835,-0.47989753293824,
-7.95701473113232));
#132964=CARTESIAN_POINT('Ctrl Pts',(22.5298702510011,-0.432691552635531,
-7.94881084346073));
#132965=CARTESIAN_POINT('Ctrl Pts',(22.6119540851012,-0.396664012856216,
-7.94368124252772));
#132966=CARTESIAN_POINT('Ctrl Pts',(22.7178990892324,-0.338715415524575,
-7.93690452528127));
#132967=CARTESIAN_POINT('Ctrl Pts',(22.7448882674401,-0.322868389504563,
-7.93516484143859));
#132968=CARTESIAN_POINT('Ctrl Pts',(22.7920362356633,-0.293220577486188,
-7.93212352032235));
#132969=CARTESIAN_POINT('Ctrl Pts',(22.8123845719503,-0.279741166603724,
-7.93081020265514));
#132970=CARTESIAN_POINT('Ctrl Pts',(22.8458680156909,-0.256399130905018,
-7.92865873181386));
#132971=CARTESIAN_POINT('Ctrl Pts',(22.8591798284966,-0.2468000552734,-7.92780650899487));
#132972=CARTESIAN_POINT('Ctrl Pts',(22.8904231188431,-0.223504089348374,
-7.92581458781756));
#132973=CARTESIAN_POINT('Ctrl Pts',(22.9082116631827,-0.209623248594206,
-7.92468586685922));
#132974=CARTESIAN_POINT('Ctrl Pts',(22.9815050389257,-0.149798734799642,
-7.92002979168096));
#132975=CARTESIAN_POINT('Ctrl Pts',(23.034064820614,-0.100383923271257,
-7.91667454246241));
#132976=CARTESIAN_POINT('Ctrl Pts',(23.1475970402999,0.0224162361659275,
-7.90891702684744));
#132977=CARTESIAN_POINT('Ctrl Pts',(23.2056052200213,0.0981335695832763,
-7.90453139757395));
#132978=CARTESIAN_POINT('Ctrl Pts',(23.2755930363982,0.209449138652271,
-7.89814265424258));
#132979=CARTESIAN_POINT('Ctrl Pts',(23.2938290078715,0.24086172682944,-7.89634763221282));
#132980=CARTESIAN_POINT('Ctrl Pts',(23.324084694423,0.297491370902265,-7.89310749174407));
#132981=CARTESIAN_POINT('Ctrl Pts',(23.336559926694,0.322446632448505,-7.89167838397129));
#132982=CARTESIAN_POINT('Ctrl Pts',(23.3628895160827,0.378892212641739,
-7.8884373539397));
#132983=CARTESIAN_POINT('Ctrl Pts',(23.3763807425985,0.410534641874167,
-7.88661461070158));
#132984=CARTESIAN_POINT('Ctrl Pts',(23.4145875705298,0.509156971457689,
-7.88091183326549));
#132985=CARTESIAN_POINT('Ctrl Pts',(23.4357205178586,0.577416881690707,
-7.87693014128697));
#132986=CARTESIAN_POINT('Ctrl Pts',(23.473692996158,0.738942701068894,-7.86752949903149));
#132987=CARTESIAN_POINT('Ctrl Pts',(23.4868258235285,0.832792439124259,
-7.86207848972414));
#132988=CARTESIAN_POINT('Ctrl Pts',(23.4925210920485,0.953460837313003,
-7.85543830034237));
#132989=CARTESIAN_POINT('Ctrl Pts',(23.4930894613947,0.979695454057876,
-7.85401775081592));
#132990=CARTESIAN_POINT('Ctrl Pts',(23.4929258171609,1.02225335893383,-7.85176374258021));
#132991=CARTESIAN_POINT('Ctrl Pts',(23.4926041471341,1.0385721741514,-7.85091175838352));
#132992=CARTESIAN_POINT('Ctrl Pts',(23.4912966068882,1.07530848984636,-7.84902399298244));
#132993=CARTESIAN_POINT('Ctrl Pts',(23.490163938166,1.09571686872353,-7.84799522589264));
#132994=CARTESIAN_POINT('Ctrl Pts',(23.4844035555486,1.17205844097231,-7.84420258776438));
#132995=CARTESIAN_POINT('Ctrl Pts',(23.4771308214474,1.22775148193488,-7.84154707939638));
#132996=CARTESIAN_POINT('Ctrl Pts',(23.4515938273841,1.3646610016949,-7.83504905181641));
#132997=CARTESIAN_POINT('Ctrl Pts',(23.4297677109401,1.44502724139663,-7.83125538581598));
#132998=CARTESIAN_POINT('Ctrl Pts',(23.3835267062311,1.57330813667429,-7.82481894732443));
#132999=CARTESIAN_POINT('Ctrl Pts',(23.3629035441215,1.62240179620157,-7.82225978846643));
#133000=CARTESIAN_POINT('Ctrl Pts',(23.3268218294822,1.69720958368327,-7.81814280302905));
#133001=CARTESIAN_POINT('Ctrl Pts',(23.3130805107826,1.72370638247791,-7.81664007640385));
#133002=CARTESIAN_POINT('Ctrl Pts',(23.2844661838071,1.77517261073433,-7.8136237035442));
#133003=CARTESIAN_POINT('Ctrl Pts',(23.269638969942,1.80015337106273,-7.81211204137438));
#133004=CARTESIAN_POINT('Ctrl Pts',(23.2290208064344,1.86438378038673,-7.80809379194539));
#133005=CARTESIAN_POINT('Ctrl Pts',(23.2021289864727,1.90289864861316,-7.80554994523843));
#133006=CARTESIAN_POINT('Ctrl Pts',(23.1339596224093,1.99161757948425,-7.79936801720477));
#133007=CARTESIAN_POINT('Ctrl Pts',(23.0911854309392,2.04055788104414,-7.79568842927852));
#133008=CARTESIAN_POINT('Ctrl Pts',(22.9966083279801,2.13590115824035,-7.78803989644304));
#133009=CARTESIAN_POINT('Ctrl Pts',(22.9445002796644,2.18178966106186,-7.78407766963962));
#133010=CARTESIAN_POINT('Ctrl Pts',(22.8894915957587,2.22401164291842,-7.78024830238043));
#133011=CARTESIAN_POINT('Origin',(21.9499999789786,0.999999999999992,-4.89578827641128));
#133012=CARTESIAN_POINT('',(22.8894915988056,2.22401164057975,-7.28231538991333));
#133013=CARTESIAN_POINT('',(22.889491673488,2.22401158325724,-7.32301705809308));
#133014=CARTESIAN_POINT('',(22.8894916101512,2.22401163187148,-4.89578827641128));
#133015=CARTESIAN_POINT('',(20.4070000765807,0.999451182879079,-7.64468155021554));
#133016=CARTESIAN_POINT('Ctrl Pts',(22.889491673488,2.22401158325724,-7.32301705809308));
#133017=CARTESIAN_POINT('Ctrl Pts',(22.9174806528591,2.20252860546791,-7.32465069545391));
#133018=CARTESIAN_POINT('Ctrl Pts',(22.9447372388077,2.18008218588996,-7.32628495168413));
#133019=CARTESIAN_POINT('Ctrl Pts',(23.0197626922916,2.11384526528419,-7.33096307828763));
#133020=CARTESIAN_POINT('Ctrl Pts',(23.0655639624875,2.06796984703058,-7.3340413964136));
#133021=CARTESIAN_POINT('Ctrl Pts',(23.1289816116115,1.99590515951898,-7.33877506694343));
#133022=CARTESIAN_POINT('Ctrl Pts',(23.1489002156125,1.97183477725879,-7.34034038117292));
#133023=CARTESIAN_POINT('Ctrl Pts',(23.1856445951545,1.92458136313975,-7.34339398889923));
#133024=CARTESIAN_POINT('Ctrl Pts',(23.2025823945152,1.90150178568562,-7.34487714599291));
#133025=CARTESIAN_POINT('Ctrl Pts',(23.2430084589554,1.8430765515422,-7.34861675317297));
#133026=CARTESIAN_POINT('Ctrl Pts',(23.2656981967317,1.80720924795092,-7.35089993945748));
#133027=CARTESIAN_POINT('Ctrl Pts',(23.343388625699,1.67240211298067,-7.35943294626908));
#133028=CARTESIAN_POINT('Ctrl Pts',(23.3889349482176,1.56843495398951,-7.36595299097858));
#133029=CARTESIAN_POINT('Ctrl Pts',(23.4328651501621,1.42792563815277,-7.37426533489055));
#133030=CARTESIAN_POINT('Ctrl Pts',(23.4419514411839,1.39508289850369,-7.37617185478681));
#133031=CARTESIAN_POINT('Ctrl Pts',(23.4559961654803,1.33688310572054,-7.3794593624945));
#133032=CARTESIAN_POINT('Ctrl Pts',(23.4614191737601,1.31165188862252,-7.38085507067608));
#133033=CARTESIAN_POINT('Ctrl Pts',(23.469205645451,1.27041507889937,-7.38307596209645));
#133034=CARTESIAN_POINT('Ctrl Pts',(23.4719546191998,1.25448834457933,-7.38391895058142));
#133035=CARTESIAN_POINT('Ctrl Pts',(23.4776546813915,1.21805746436626,-7.38581159163521));
#133036=CARTESIAN_POINT('Ctrl Pts',(23.4804440729965,1.19753202611035,-7.38685345524712));
#133037=CARTESIAN_POINT('Ctrl Pts',(23.4895700144441,1.11848163026228,-7.39079267040249));
#133038=CARTESIAN_POINT('Ctrl Pts',(23.4929694967009,1.05966462694489,-7.39357090071966));
#133039=CARTESIAN_POINT('Ctrl Pts',(23.4930614715204,0.880834542133844,
-7.40190366196691));
#133040=CARTESIAN_POINT('Ctrl Pts',(23.4791348666175,0.761284932770572,
-7.40735185444612));
#133041=CARTESIAN_POINT('Ctrl Pts',(23.4437488052126,0.611803904543438,
-7.41486325513049));
#133042=CARTESIAN_POINT('Ctrl Pts',(23.4349265867479,0.579316586949283,
-7.41653677307096));
#133043=CARTESIAN_POINT('Ctrl Pts',(23.4168013484243,0.520278644999048,
-7.41966737658068));
#133044=CARTESIAN_POINT('Ctrl Pts',(23.407821005861,0.493643840414046,-7.42111398176074));
#133045=CARTESIAN_POINT('Ctrl Pts',(23.3852925784078,0.432404852236581,
-7.42452567038954));
#133046=CARTESIAN_POINT('Ctrl Pts',(23.3712122651412,0.398016246501824,
-7.42650678676884));
#133047=CARTESIAN_POINT('Ctrl Pts',(23.337797951035,0.324132601264742,-7.43090906588496));
#133048=CARTESIAN_POINT('Ctrl Pts',(23.3179893484773,0.28488837636492,-7.43334264362142));
#133049=CARTESIAN_POINT('Ctrl Pts',(23.236198919598,0.138716953140601,-7.44274398069557));
#133050=CARTESIAN_POINT('Ctrl Pts',(23.1631330001449,0.0385303398521764,
-7.44994267268712));
#133051=CARTESIAN_POINT('Ctrl Pts',(23.0643556210841,-0.0674810929042513,
-7.45781349628265));
#133052=CARTESIAN_POINT('Ctrl Pts',(23.0494852719459,-0.0827910963252965,
-7.4589561060049));
#133053=CARTESIAN_POINT('Ctrl Pts',(23.0227871258641,-0.109161240994213,
-7.46092699576836));
#133054=CARTESIAN_POINT('Ctrl Pts',(23.0110954006843,-0.120351487063606,
-7.46176363932748));
#133055=CARTESIAN_POINT('Ctrl Pts',(22.981368965395,-0.147919990082372,
-7.46382778665516));
#133056=CARTESIAN_POINT('Ctrl Pts',(22.9631189616701,-0.164058561511551,
-7.46503989993721));
#133057=CARTESIAN_POINT('Ctrl Pts',(22.9205753568766,-0.199921262072684,
-7.46776183320603));
#133058=CARTESIAN_POINT('Ctrl Pts',(22.8960484320435,-0.219352322342665,
-7.46925776557148));
#133059=CARTESIAN_POINT('Ctrl Pts',(22.7994993422812,-0.291173631194641,
-7.4749384043586));
#133060=CARTESIAN_POINT('Ctrl Pts',(22.7235842798912,-0.33803835266542,
-7.47898627597311));
#133061=CARTESIAN_POINT('Ctrl Pts',(22.5901404182338,-0.405244647338239,
-7.4859933365481));
#133062=CARTESIAN_POINT('Ctrl Pts',(22.5346883073623,-0.42920643891053,
-7.48887462363873));
#133063=CARTESIAN_POINT('Ctrl Pts',(22.4490338252202,-0.46039827214964,
-7.4933776447817));
#133064=CARTESIAN_POINT('Ctrl Pts',(22.4197814008684,-0.470069096749479,
-7.49492378896884));
#133065=CARTESIAN_POINT('Ctrl Pts',(22.3626510756701,-0.487076964808972,
-7.49796886546628));
#133066=CARTESIAN_POINT('Ctrl Pts',(22.334818380678,-0.494521155600971,
-7.49946373531877));
#133067=CARTESIAN_POINT('Ctrl Pts',(22.2640441314933,-0.511342491691904,
-7.50329856917447));
#133068=CARTESIAN_POINT('Ctrl Pts',(22.220881979117,-0.519671781551221,
-7.50566853636649));
#133069=CARTESIAN_POINT('Ctrl Pts',(22.0689622849165,-0.542310778490602,
-7.51411276100414));
#133070=CARTESIAN_POINT('Ctrl Pts',(21.959089791038,-0.546863974449758,
-7.52042763261872));
#133071=CARTESIAN_POINT('Ctrl Pts',(21.8040087556298,-0.536759606479476,
-7.52920406591462));
#133072=CARTESIAN_POINT('Ctrl Pts',(21.7584916095135,-0.531753435522759,
-7.53175848313519));
#133073=CARTESIAN_POINT('Ctrl Pts',(21.6929704889091,-0.521580267026578,
-7.53534778085406));
#133074=CARTESIAN_POINT('Ctrl Pts',(21.6727430030873,-0.518024807557795,
-7.53644348220558));
#133075=CARTESIAN_POINT('Ctrl Pts',(21.6364961700584,-0.510904835171577,
-7.53837748730586));
#133076=CARTESIAN_POINT('Ctrl Pts',(21.6204535767768,-0.507487061365945,
-7.53922228011786));
#133077=CARTESIAN_POINT('Ctrl Pts',(21.5786297080394,-0.497877137387341,
-7.54139966970917));
#133078=CARTESIAN_POINT('Ctrl Pts',(21.5529485722373,-0.49127533430978,
-7.5427123542691));
#133079=CARTESIAN_POINT('Ctrl Pts',(21.49333990079,-0.474302659211232,-7.54572781863924));
#133080=CARTESIAN_POINT('Ctrl Pts',(21.4595742432316,-0.463417085448077,
-7.5474118348925));
#133081=CARTESIAN_POINT('Ctrl Pts',(21.3059050064523,-0.407959393115651,
-7.55507887264987));
#133082=CARTESIAN_POINT('Ctrl Pts',(21.1914675442868,-0.349754408263219,
-7.56084381663139));
#133083=CARTESIAN_POINT('Ctrl Pts',(21.0567624245766,-0.25864260638842,
-7.56877479948666));
#133084=CARTESIAN_POINT('Ctrl Pts',(21.0286687306386,-0.238225768625484,
-7.57049700206357));
#133085=CARTESIAN_POINT('Ctrl Pts',(20.9791109395356,-0.199589215092315,
-7.5736763646391));
#133086=CARTESIAN_POINT('Ctrl Pts',(20.9574109658991,-0.181696549192534,
-7.5751210249888));
#133087=CARTESIAN_POINT('Ctrl Pts',(20.9090664583786,-0.139562669637341,
-7.57846754215476));
#133088=CARTESIAN_POINT('Ctrl Pts',(20.8827581931345,-0.114962049900615,
-7.58038305171594));
#133089=CARTESIAN_POINT('Ctrl Pts',(20.8278163997992,-0.0598589172470465,
-7.58459582033289));
#133090=CARTESIAN_POINT('Ctrl Pts',(20.7995141819669,-0.0290670452530772,
-7.58690328428394));
#133091=CARTESIAN_POINT('Ctrl Pts',(20.7048788467948,0.0826829521462757,
-7.59509720996102));
#133092=CARTESIAN_POINT('Ctrl Pts',(20.6455600305647,0.169197788408244,
-7.60114996977033));
#133093=CARTESIAN_POINT('Ctrl Pts',(20.5787194885078,0.291720585798969,
-7.60893121394299));
#133094=CARTESIAN_POINT('Ctrl Pts',(20.5630314206416,0.322956109743386,
-7.61085024488963));
#133095=CARTESIAN_POINT('Ctrl Pts',(20.5410739466015,0.370647397965778,
-7.61365723245521));
#133096=CARTESIAN_POINT('Ctrl Pts',(20.5340036243639,0.38672058250917,-7.61458287806887));
#133097=CARTESIAN_POINT('Ctrl Pts',(20.520303458396,0.419366463448125,-7.61641708828457));
#133098=CARTESIAN_POINT('Ctrl Pts',(20.5136837186262,0.435940517543099,
-7.61732503682478));
#133099=CARTESIAN_POINT('Ctrl Pts',(20.4941171895752,0.487509680540059,
-7.62008920803211));
#133100=CARTESIAN_POINT('Ctrl Pts',(20.4821503907886,0.522863799232232,
-7.62189887160568));
#133101=CARTESIAN_POINT('Ctrl Pts',(20.4287708368372,0.701672871395411,
-7.63078168924784));
#133102=CARTESIAN_POINT('Ctrl Pts',(20.4070531773116,0.850158423141492,
-7.6373883095844));
#133103=CARTESIAN_POINT('Ctrl Pts',(20.4070000765807,0.999451182879078,
-7.64468155021554));
#133104=CARTESIAN_POINT('Ctrl Pts',(20.4070000761094,0.999452509765842,
-7.64468161503654));
#133105=CARTESIAN_POINT('Ctrl Pts',(20.4069914884943,1.02365511365021,-7.64586395966915));
#133106=CARTESIAN_POINT('Ctrl Pts',(20.4075523420559,1.0478539923095,-7.64706070389743));
#133107=CARTESIAN_POINT('Ctrl Pts',(20.4098303397597,1.09659975623545,-7.6495067341467));
#133108=CARTESIAN_POINT('Ctrl Pts',(20.4115658938258,1.12113839695251,-7.65075618920184));
#133109=CARTESIAN_POINT('Ctrl Pts',(20.4167554741822,1.17588051974584,-7.65358872521351));
#133110=CARTESIAN_POINT('Ctrl Pts',(20.4205169287147,1.20604393197918,-7.65518047584784));
#133111=CARTESIAN_POINT('Ctrl Pts',(20.4334913207319,1.28984679235276,-7.65969431087745));
#133112=CARTESIAN_POINT('Ctrl Pts',(20.4446539627764,1.3431358168734,-7.66267158712686));
#133113=CARTESIAN_POINT('Ctrl Pts',(20.4842124700803,1.49222414245962,-7.67127933065706));
#133114=CARTESIAN_POINT('Ctrl Pts',(20.5191225231289,1.58600828362626,-7.67704303295215));
#133115=CARTESIAN_POINT('Ctrl Pts',(20.5757445171939,1.70223815246044,-7.68430550542341));
#133116=CARTESIAN_POINT('Ctrl Pts',(20.5893997189086,1.72834303462435,-7.68594337704621));
#133117=CARTESIAN_POINT('Ctrl Pts',(20.6152059849074,1.77441545386583,-7.68882741006617));
#133118=CARTESIAN_POINT('Ctrl Pts',(20.6270792470567,1.79452825563682,-7.69008402747835));
#133119=CARTESIAN_POINT('Ctrl Pts',(20.6479170113864,1.82806343534428,-7.69216538973155));
#133120=CARTESIAN_POINT('Ctrl Pts',(20.6566429198552,1.84162739480979,-7.69300271689554));
#133121=CARTESIAN_POINT('Ctrl Pts',(20.6780538700932,1.873789856518,-7.69497760930347));
#133122=CARTESIAN_POINT('Ctrl Pts',(20.6909358458058,1.89225177079883,-7.69610370305999));
#133123=CARTESIAN_POINT('Ctrl Pts',(20.7487534790556,1.97136657519879,-7.70092546515341));
#133124=CARTESIAN_POINT('Ctrl Pts',(20.7977043778059,2.02896198846566,-7.70442897853137));
#133125=CARTESIAN_POINT('Ctrl Pts',(20.898527760055,2.13132889495774,-7.71108426465713));
#133126=CARTESIAN_POINT('Ctrl Pts',(20.9495448845472,2.17668522573863,-7.71423041094079));
#133127=CARTESIAN_POINT('Ctrl Pts',(21.0415676646499,2.24817327739315,-7.71976850765597));
#133128=CARTESIAN_POINT('Ctrl Pts',(21.081112541018,2.27601721332088,-7.72210935365691));
#133129=CARTESIAN_POINT('Ctrl Pts',(21.1467554493328,2.31776900427268,-7.72598116723772));
#133130=CARTESIAN_POINT('Ctrl Pts',(21.1720603481634,2.33286410094567,-7.72747033571417));
#133131=CARTESIAN_POINT('Ctrl Pts',(21.2240474592773,2.36189095116137,-7.73053078079335));
#133132=CARTESIAN_POINT('Ctrl Pts',(21.2507360896607,2.37578482245284,-7.73210246767179));
#133133=CARTESIAN_POINT('Ctrl Pts',(21.3258391274469,2.41213279801038,-7.73653177117818));
#133134=CARTESIAN_POINT('Ctrl Pts',(21.3750349785873,2.43286784019779,-7.73944173894915));
#133135=CARTESIAN_POINT('Ctrl Pts',(21.5164731889253,2.48402276129025,-7.74780912558417));
#133136=CARTESIAN_POINT('Ctrl Pts',(21.6106532633793,2.50834714407414,-7.75339476799625));
#133137=CARTESIAN_POINT('Ctrl Pts',(21.738434647399,2.52876942832236,-7.76068203807632));
#133138=CARTESIAN_POINT('Ctrl Pts',(21.7705384172451,2.53286971983794,-7.76248719636736));
#133139=CARTESIAN_POINT('Ctrl Pts',(21.8275932519181,2.53833953472043,-7.76562606886156));
#133140=CARTESIAN_POINT('Ctrl Pts',(21.852493391881,2.54011834796466,-7.76697271342015));
#133141=CARTESIAN_POINT('Ctrl Pts',(21.8938578065908,2.54206602592885,-7.76915985300163));
#133142=CARTESIAN_POINT('Ctrl Pts',(21.9102997637596,2.54257690982044,-7.77001565020145));
#133143=CARTESIAN_POINT('Ctrl Pts',(21.9485699524295,2.54315366347932,-7.77197567170477));
#133144=CARTESIAN_POINT('Ctrl Pts',(21.9703967204295,2.54301955099044,-7.7730705618745));
#133145=CARTESIAN_POINT('Ctrl Pts',(22.0924079379571,2.53968024761724,-7.77909704930489));
#133146=CARTESIAN_POINT('Ctrl Pts',(22.192104685531,2.52718175694384,-7.78367956488091));
#133147=CARTESIAN_POINT('Ctrl Pts',(22.3415418178797,2.49343491596646,-7.79082096802479));
#133148=CARTESIAN_POINT('Ctrl Pts',(22.3925562044891,2.47912017361101,-7.79330709691478));
#133149=CARTESIAN_POINT('Ctrl Pts',(22.4822656362566,2.44889014326399,-7.79786208085157));
#133150=CARTESIAN_POINT('Ctrl Pts',(22.5212404332267,2.43397119329344,-7.79990532598986));
#133151=CARTESIAN_POINT('Ctrl Pts',(22.5860208528212,2.40611380343839,-7.80344086774118));
#133152=CARTESIAN_POINT('Ctrl Pts',(22.6121555307083,2.39399729967823,-7.80490705909161));
#133153=CARTESIAN_POINT('Ctrl Pts',(22.6667068889749,2.36682603588452,-7.80805986555164));
#133154=CARTESIAN_POINT('Ctrl Pts',(22.6950226131164,2.35160026961135,-7.8097515732248));
#133155=CARTESIAN_POINT('Ctrl Pts',(22.7807550611733,2.3019878029393,-7.81505186375773));
#133156=CARTESIAN_POINT('Ctrl Pts',(22.836421930236,2.26474532986395,-7.81875218487559));
#133157=CARTESIAN_POINT('Ctrl Pts',(22.889491610182,2.22401163184779,-7.82252261963806));
#133158=CARTESIAN_POINT('',(20.4070004000582,1.00121065507753,-7.60402771031333));
#133159=CARTESIAN_POINT('Ctrl Pts',(22.8894915957587,2.22401164291842,-7.78024830238043));
#133160=CARTESIAN_POINT('Ctrl Pts',(22.880257682641,2.23109914409893,-7.77960549397171));
#133161=CARTESIAN_POINT('Ctrl Pts',(22.8709420309963,2.23808333424448,-7.77896653901388));
#133162=CARTESIAN_POINT('Ctrl Pts',(22.8435437238085,2.25814403624021,-7.77711690966168));
#133163=CARTESIAN_POINT('Ctrl Pts',(22.8252564149561,2.27093395165168,-7.77591928997979));
#133164=CARTESIAN_POINT('Ctrl Pts',(22.793323012972,2.29225146272404,-7.77389927352338));
#133165=CARTESIAN_POINT('Ctrl Pts',(22.7798107599659,2.30096951712248,-7.7730663387722));
#133166=CARTESIAN_POINT('Ctrl Pts',(22.7463339099439,2.32183478920938,-7.7710542050887));
#133167=CARTESIAN_POINT('Ctrl Pts',(22.7262256245581,2.33374240125316,-7.76988840332241));
#133168=CARTESIAN_POINT('Ctrl Pts',(22.6801787966661,2.35961583585793,-7.76729710652219));
#133169=CARTESIAN_POINT('Ctrl Pts',(22.6540950310548,2.37330500137809,-7.76588352073751));
#133170=CARTESIAN_POINT('Ctrl Pts',(22.5586012495163,2.41998515159651,-7.760848482913));
#133171=CARTESIAN_POINT('Ctrl Pts',(22.4871420125279,2.44852769964705,-7.7573364284221));
#133172=CARTESIAN_POINT('Ctrl Pts',(22.3462507685608,2.4929361219175,-7.75046208951894));
#133173=CARTESIAN_POINT('Ctrl Pts',(22.2772657339821,2.50955920336922,-7.74711737841442));
#133174=CARTESIAN_POINT('Ctrl Pts',(22.1755363456467,2.52676973305955,-7.74204962671551));
#133175=CARTESIAN_POINT('Ctrl Pts',(22.1435263310517,2.53115637404756,-7.74043681604782));
#133176=CARTESIAN_POINT('Ctrl Pts',(22.0832329886062,2.53749807259431,-7.73735346166105));
#133177=CARTESIAN_POINT('Ctrl Pts',(22.0549874927621,2.5396846585077,-7.73589047344871));
#133178=CARTESIAN_POINT('Ctrl Pts',(21.9870832276432,2.54306419921142,-7.73232370777881));
#133179=CARTESIAN_POINT('Ctrl Pts',(21.9474087683684,2.54350744100091,-7.73019897156096));
#133180=CARTESIAN_POINT('Ctrl Pts',(21.8590267161619,2.54108724920566,-7.72537508504436));
#133181=CARTESIAN_POINT('Ctrl Pts',(21.8103835658148,2.53744359000075,-7.72265822272179));
#133182=CARTESIAN_POINT('Ctrl Pts',(21.6762829786785,2.52098179466736,-7.71503687152916));
#133183=CARTESIAN_POINT('Ctrl Pts',(21.5916049749986,2.50328291115702,-7.71006754088825));
#133184=CARTESIAN_POINT('Ctrl Pts',(21.4740633261771,2.46821365983889,-7.70321950518927));
#133185=CARTESIAN_POINT('Ctrl Pts',(21.4396487033743,2.45660871563313,-7.70122249865693));
#133186=CARTESIAN_POINT('Ctrl Pts',(21.3890485483809,2.43753197216848,-7.69832881259261));
#133187=CARTESIAN_POINT('Ctrl Pts',(21.3725322363799,2.43097719747414,-7.69739125950921));
#133188=CARTESIAN_POINT('Ctrl Pts',(21.3397321112258,2.41729949552865,-7.69554858472773));
#133189=CARTESIAN_POINT('Ctrl Pts',(21.3234507545024,2.41017759603771,-7.69464362410134));
#133190=CARTESIAN_POINT('Ctrl Pts',(21.2741719712013,2.38759971781135,-7.69192417094538));
#133191=CARTESIAN_POINT('Ctrl Pts',(21.241594383403,2.37125428239819,-7.6901534763187));
#133192=CARTESIAN_POINT('Ctrl Pts',(21.1572101034558,2.32510458212038,-7.68556538245284));
#133193=CARTESIAN_POINT('Ctrl Pts',(21.1065029389211,2.29341842461624,-7.68280539233803));
#133194=CARTESIAN_POINT('Ctrl Pts',(20.9870503155218,2.20875486251205,-7.67602597713628));
#133195=CARTESIAN_POINT('Ctrl Pts',(20.9206922636456,2.15277262916053,-7.6720045182926));
#133196=CARTESIAN_POINT('Ctrl Pts',(20.8346040841136,2.06675605876907,-7.66607649630674));
#133197=CARTESIAN_POINT('Ctrl Pts',(20.8106717726939,2.04115681254455,-7.66434053421702));
#133198=CARTESIAN_POINT('Ctrl Pts',(20.7692000002589,1.99365282861371,-7.66115272455574));
#133199=CARTESIAN_POINT('Ctrl Pts',(20.7513470825887,1.97204199505773,-7.65971416377032));
#133200=CARTESIAN_POINT('Ctrl Pts',(20.7122980387137,1.92206083279264,-7.65640720418107));
#133201=CARTESIAN_POINT('Ctrl Pts',(20.6914706019602,1.8934236519855,-7.65452618947099));
#133202=CARTESIAN_POINT('Ctrl Pts',(20.648816414946,1.83032067502098,-7.65040791663656));
#133203=CARTESIAN_POINT('Ctrl Pts',(20.6273343520704,1.79565469516914,-7.64816138106526));
#133204=CARTESIAN_POINT('Ctrl Pts',(20.559384708497,1.67563148217609,-7.64045517225515));
#133205=CARTESIAN_POINT('Ctrl Pts',(20.5196136451572,1.58675573281389,-7.6348516282934));
#133206=CARTESIAN_POINT('Ctrl Pts',(20.4755583497264,1.45660814296849,-7.62713291457989));
#133207=CARTESIAN_POINT('Ctrl Pts',(20.4641486580224,1.41798967558686,-7.62490234084615));
#133208=CARTESIAN_POINT('Ctrl Pts',(20.4495810968905,1.36049322952509,-7.62170857570756));
#133209=CARTESIAN_POINT('Ctrl Pts',(20.44524292523,1.3419334220221,-7.62069684308843));
#133210=CARTESIAN_POINT('Ctrl Pts',(20.43773241531,1.30688367478168,-7.61882817541303));
#133211=CARTESIAN_POINT('Ctrl Pts',(20.4344833899312,1.29041393168936,-7.61796791226469));
#133212=CARTESIAN_POINT('Ctrl Pts',(20.4262000145396,1.24449007017566,-7.61561161196411));
#133213=CARTESIAN_POINT('Ctrl Pts',(20.421751238443,1.21493652510305,-7.61414308772383));
#133214=CARTESIAN_POINT('Ctrl Pts',(20.4107765321421,1.12419665233873,-7.60973178671522));
#133215=CARTESIAN_POINT('Ctrl Pts',(20.4070487067959,1.0627332925579,-7.60687691375844));
#133216=CARTESIAN_POINT('Ctrl Pts',(20.4070004535616,1.00121019123005,-7.60402759549201));
#133217=CARTESIAN_POINT('Ctrl Pts',(20.4070004539288,1.00121065934862,-7.60402761717198));
#133218=CARTESIAN_POINT('Ctrl Pts',(20.4069404364847,0.924717723665204,
-7.60048500117601));
#133219=CARTESIAN_POINT('Ctrl Pts',(20.4125686362602,0.848325809332539,
-7.59695636083124));
#133220=CARTESIAN_POINT('Ctrl Pts',(20.4302233931201,0.72980335152939,-7.5912204783422));
#133221=CARTESIAN_POINT('Ctrl Pts',(20.4384109065201,0.687229799530118,
-7.58910750751098));
#133222=CARTESIAN_POINT('Ctrl Pts',(20.4549766894986,0.617146204419026,
-7.58550847460207));
#133223=CARTESIAN_POINT('Ctrl Pts',(20.4623512340671,0.589423888569778,
-7.58405290486925));
#133224=CARTESIAN_POINT('Ctrl Pts',(20.4792543043622,0.532337421372184,
-7.58098187890168));
#133225=CARTESIAN_POINT('Ctrl Pts',(20.4888999288707,0.503021531856045,
-7.57936334978893));
#133226=CARTESIAN_POINT('Ctrl Pts',(20.5203199021808,0.416370147408416,
-7.57444937714896));
#133227=CARTESIAN_POINT('Ctrl Pts',(20.5446380078088,0.360026980332973,
-7.57107803141705));
#133228=CARTESIAN_POINT('Ctrl Pts',(20.6118260550235,0.226779847925846,
-7.56270836534051));
#133229=CARTESIAN_POINT('Ctrl Pts',(20.6580460495585,0.151805988023286,
-7.55764830584345));
#133230=CARTESIAN_POINT('Ctrl Pts',(20.7289220841007,0.0561856460658383,
-7.55094967865945));
#133231=CARTESIAN_POINT('Ctrl Pts',(20.7481991027466,0.0317585128412778,
-7.54921574637432));
#133232=CARTESIAN_POINT('Ctrl Pts',(20.7837969757221,-0.0106472506195487,
-7.54618603170542));
#133233=CARTESIAN_POINT('Ctrl Pts',(20.7998284621887,-0.0288551467130027,
-7.5448783394791));
#133234=CARTESIAN_POINT('Ctrl Pts',(20.8272428352801,-0.0585492067619242,
-7.54274480337316));
#133235=CARTESIAN_POINT('Ctrl Pts',(20.8383879952986,-0.0702471134814875,
-7.54190452179177));
#133236=CARTESIAN_POINT('Ctrl Pts',(20.8646837503652,-0.0969929233667788,
-7.53998452909802));
#133237=CARTESIAN_POINT('Ctrl Pts',(20.8799663594014,-0.111905089105901,
-7.53891383043223));
#133238=CARTESIAN_POINT('Ctrl Pts',(20.9613090366144,-0.18804512502939,
-7.53341560865051));
#133239=CARTESIAN_POINT('Ctrl Pts',(21.0323325260271,-0.243724353494565,
-7.529278107026));
#133240=CARTESIAN_POINT('Ctrl Pts',(21.1585262692755,-0.325926637475304,
-7.52230364504257));
#133241=CARTESIAN_POINT('Ctrl Pts',(21.2111375683254,-0.355947642740331,
-7.51949311520841));
#133242=CARTESIAN_POINT('Ctrl Pts',(21.3058427372353,-0.402836267948401,
-7.51444913056078));
#133243=CARTESIAN_POINT('Ctrl Pts',(21.3471688605105,-0.42108492783576,
-7.512253396365));
#133244=CARTESIAN_POINT('Ctrl Pts',(21.4161840954563,-0.448007752659545,
-7.50855748603983));
#133245=CARTESIAN_POINT('Ctrl Pts',(21.4434235211971,-0.457760613261931,
-7.50709185163064));
#133246=CARTESIAN_POINT('Ctrl Pts',(21.4998620271572,-0.476195052972779,
-7.50403386720214));
#133247=CARTESIAN_POINT('Ctrl Pts',(21.5290761485654,-0.48478920164567,
-7.50243957182671));
#133248=CARTESIAN_POINT('Ctrl Pts',(21.6140286215346,-0.507071644878461,
-7.49776590108286));
#133249=CARTESIAN_POINT('Ctrl Pts',(21.6702971976674,-0.51852133889621,
-7.49462252480263));
#133250=CARTESIAN_POINT('Ctrl Pts',(21.8184258495567,-0.540149775638676,
-7.48625613057676));
#133251=CARTESIAN_POINT('Ctrl Pts',(21.9107950335803,-0.545262059290152,
-7.48094034631308));
#133252=CARTESIAN_POINT('Ctrl Pts',(22.0347432075985,-0.540997279014519,
-7.47395608308751));
#133253=CARTESIAN_POINT('Ctrl Pts',(22.0663869261323,-0.53893088758926,
-7.47218768193824));
#133254=CARTESIAN_POINT('Ctrl Pts',(22.1224052819572,-0.533534881598952,
-7.46910604169119));
#133255=CARTESIAN_POINT('Ctrl Pts',(22.1468063855873,-0.530594716047843,
-7.46778035822661));
#133256=CARTESIAN_POINT('Ctrl Pts',(22.1871447371499,-0.524753513699698,
-7.46562754772565));
#133257=CARTESIAN_POINT('Ctrl Pts',(22.2031239743921,-0.522182387121726,
-7.46478535310051));
#133258=CARTESIAN_POINT('Ctrl Pts',(22.2398899888756,-0.515671535944335,
-7.46287308136835));
#133259=CARTESIAN_POINT('Ctrl Pts',(22.2606412090513,-0.51155500434557,
-7.46181157540772));
#133260=CARTESIAN_POINT('Ctrl Pts',(22.402259150928,-0.480421673714395,
-7.45465113225172));
#133261=CARTESIAN_POINT('Ctrl Pts',(22.5195860978097,-0.439362599838922,
-7.44910884886831));
#133262=CARTESIAN_POINT('Ctrl Pts',(22.6866857263994,-0.357213365843605,
-7.44039011852325));
#133263=CARTESIAN_POINT('Ctrl Pts',(22.7409003166773,-0.326352063248985,
-7.43742069907414));
#133264=CARTESIAN_POINT('Ctrl Pts',(22.8190349341517,-0.275376948805524,
-7.43281614404673));
#133265=CARTESIAN_POINT('Ctrl Pts',(22.8444561289702,-0.257678873593203,
-7.43126296786823));
#133266=CARTESIAN_POINT('Ctrl Pts',(22.8920837958749,-0.222346100866249,
-7.42823567730313));
#133267=CARTESIAN_POINT('Ctrl Pts',(22.9143705766032,-0.204840705467908,
-7.42676667744416));
#133268=CARTESIAN_POINT('Ctrl Pts',(22.9690042151343,-0.159440733914313,
-7.4230264266045));
#133269=CARTESIAN_POINT('Ctrl Pts',(23.0006972133969,-0.130799421437278,
-7.42072732038427));
#133270=CARTESIAN_POINT('Ctrl Pts',(23.106417467474,-0.0269731518823635,
-7.41259669149464));
#133271=CARTESIAN_POINT('Ctrl Pts',(23.1738932938146,0.0544542401824089,
-7.40654052091814));
#133272=CARTESIAN_POINT('Ctrl Pts',(23.2535312802292,0.173512248879439,
-7.39842681675134));
#133273=CARTESIAN_POINT('Ctrl Pts',(23.2733737991496,0.20567146503963,-7.39630328286484));
#133274=CARTESIAN_POINT('Ctrl Pts',(23.3056473382805,0.262550262435295,
-7.39269874334556));
#133275=CARTESIAN_POINT('Ctrl Pts',(23.3186312646397,0.286935872596983,
-7.39119919578614));
#133276=CARTESIAN_POINT('Ctrl Pts',(23.3383081643222,0.326411748991351,
-7.38885869998939));
#133277=CARTESIAN_POINT('Ctrl Pts',(23.3454256109164,0.341282960369145,
-7.38799636940707));
#133278=CARTESIAN_POINT('Ctrl Pts',(23.3605946106287,0.374327014451219,
-7.38612570290247));
#133279=CARTESIAN_POINT('Ctrl Pts',(23.368535872225,0.392546388425967,-7.38512302140777));
#133280=CARTESIAN_POINT('Ctrl Pts',(23.3959012989305,0.45879568257635,-7.38156294166614));
#133281=CARTESIAN_POINT('Ctrl Pts',(23.4132568690596,0.507645691789587,
-7.37909772323242));
#133282=CARTESIAN_POINT('Ctrl Pts',(23.4586594830442,0.659232550490287,
-7.37168572094013));
#133283=CARTESIAN_POINT('Ctrl Pts',(23.4785655803018,0.764069051469471,
-7.36686324167786));
#133284=CARTESIAN_POINT('Ctrl Pts',(23.4911695183809,0.913275743994522,
-7.35969503151058));
#133285=CARTESIAN_POINT('Ctrl Pts',(23.4929962386157,0.9565625538337,-7.35758324507889));
#133286=CARTESIAN_POINT('Ctrl Pts',(23.4930024230829,1.02827377338184,-7.35399914715059));
#133287=CARTESIAN_POINT('Ctrl Pts',(23.4922204160075,1.05667400551033,-7.3525576714625));
#133288=CARTESIAN_POINT('Ctrl Pts',(23.488957872469,1.11578414100086,-7.34950475898091));
#133289=CARTESIAN_POINT('Ctrl Pts',(23.4863406531038,1.14647363838399,-7.34788989712755));
#133290=CARTESIAN_POINT('Ctrl Pts',(23.4758491210652,1.23729722655133,-7.34301712938948));
#133291=CARTESIAN_POINT('Ctrl Pts',(23.4653473529279,1.29706356196314,-7.33968549298856));
#133292=CARTESIAN_POINT('Ctrl Pts',(23.4248616387608,1.46777859122865,-7.32985116481224));
#133293=CARTESIAN_POINT('Ctrl Pts',(23.3859786537944,1.57619262085885,-7.32318266929766));
#133294=CARTESIAN_POINT('Ctrl Pts',(23.3235480041885,1.7035220866657,-7.31537606907888));
#133295=CARTESIAN_POINT('Ctrl Pts',(23.3110311094961,1.72744204167632,-7.31391246444009));
#133296=CARTESIAN_POINT('Ctrl Pts',(23.2899057577224,1.7653566217664,-7.31161137532962));
#133297=CARTESIAN_POINT('Ctrl Pts',(23.2816905682516,1.77956302467632,-7.31075382499874));
#133298=CARTESIAN_POINT('Ctrl Pts',(23.262884807307,1.81091830023135,-7.30887427813815));
#133299=CARTESIAN_POINT('Ctrl Pts',(23.2521822061575,1.82799552098128,-7.30785857812452));
#133300=CARTESIAN_POINT('Ctrl Pts',(23.2077044960095,1.89596816201364,-7.30382859710218));
#133301=CARTESIAN_POINT('Ctrl Pts',(23.1712534058312,1.94505068856687,-7.30094689308019));
#133302=CARTESIAN_POINT('Ctrl Pts',(23.059824766865,2.07784054179424,-7.29287211099152));
#133303=CARTESIAN_POINT('Ctrl Pts',(22.9785112118013,2.15568452861694,-7.28776613946278));
#133304=CARTESIAN_POINT('Ctrl Pts',(22.8894915988056,2.22401164057974,-7.28231538991333));
#133305=CARTESIAN_POINT('Origin',(21.9499999789786,0.999999999999992,-4.89578827641128));
#133306=CARTESIAN_POINT('',(22.8894916066884,2.22401163452936,-6.78051560659813));
#133307=CARTESIAN_POINT('',(22.8894530727892,2.22394970963619,-6.82271760993144));
#133308=CARTESIAN_POINT('',(22.8894916101512,2.22401163187148,-4.89578827641128));
#133309=CARTESIAN_POINT('',(20.406507169633,1.00049669003439,-7.14664979013704));
#133310=CARTESIAN_POINT('Ctrl Pts',(22.8894530727892,2.22394970963619,-6.82271760993144));
#133311=CARTESIAN_POINT('Ctrl Pts',(22.9353005742457,2.18892258955494,-6.82591636290728));
#133312=CARTESIAN_POINT('Ctrl Pts',(22.9791500519513,2.15135845546692,-6.829135128161));
#133313=CARTESIAN_POINT('Ctrl Pts',(23.0207002168903,2.11149723851871,-6.83231403385656));
#133314=CARTESIAN_POINT('Ctrl Pts',(23.059743469323,2.07404103207845,-6.83530114155428));
#133315=CARTESIAN_POINT('Ctrl Pts',(23.0967567332383,2.03455601206123,-6.83825257867589));
#133316=CARTESIAN_POINT('Ctrl Pts',(23.1315058091072,1.99327445448767,-6.8411059364984));
#133317=CARTESIAN_POINT('Ctrl Pts',(23.1337965278077,1.99055310338541,-6.84129403474158));
#133318=CARTESIAN_POINT('Ctrl Pts',(23.1360774251152,1.98782393969824,-6.84148170676424));
#133319=CARTESIAN_POINT('Ctrl Pts',(23.1383484415223,1.98508702747687,-6.84166893468789));
#133320=CARTESIAN_POINT('Ctrl Pts',(23.1454578829252,1.97651909419329,-6.84225505372602));
#133321=CARTESIAN_POINT('Ctrl Pts',(23.1524703651171,1.9678754174032,-6.84283679013381));
#133322=CARTESIAN_POINT('Ctrl Pts',(23.1593839597114,1.95915822782426,-6.84341356061474));
#133323=CARTESIAN_POINT('Ctrl Pts',(23.1593944945009,1.95914494475483,-6.84341443948542));
#133324=CARTESIAN_POINT('Ctrl Pts',(23.1594050290725,1.95913166150046,-6.84341531834532));
#133325=CARTESIAN_POINT('Ctrl Pts',(23.1594155634263,1.95911837806115,-6.84341619719443));
#133326=CARTESIAN_POINT('Ctrl Pts',(23.1918413993482,1.91823057129339,-6.84612138611208));
#133327=CARTESIAN_POINT('Ctrl Pts',(23.2222034754519,1.8755861315841,-6.84872442054874));
#133328=CARTESIAN_POINT('Ctrl Pts',(23.2503299501565,1.83143439238815,-6.85127679550709));
#133329=CARTESIAN_POINT('Ctrl Pts',(23.2531698104295,1.826976500973,-6.85153450246546));
#133330=CARTESIAN_POINT('Ctrl Pts',(23.2559868805442,1.82250328730227,-6.85179169297886));
#133331=CARTESIAN_POINT('Ctrl Pts',(23.2587809847565,1.81801503743372,-6.85204842005146));
#133332=CARTESIAN_POINT('Ctrl Pts',(23.2892065310885,1.76914160826103,-6.85484397127236));
#133333=CARTESIAN_POINT('Ctrl Pts',(23.3169092064515,1.71847955854335,-6.85758527374401));
#133334=CARTESIAN_POINT('Ctrl Pts',(23.3417102552614,1.66638007405639,-6.86033245303685));
#133335=CARTESIAN_POINT('Ctrl Pts',(23.3664883206591,1.61432887075016,-6.8630770864876));
#133336=CARTESIAN_POINT('Ctrl Pts',(23.3883705234435,1.56084319642377,-6.8658280233161));
#133337=CARTESIAN_POINT('Ctrl Pts',(23.4072216783572,1.5062830451516,-6.86862842195339));
#133338=CARTESIAN_POINT('Ctrl Pts',(23.4260624850877,1.45175284421613,-6.87142728333537));
#133339=CARTESIAN_POINT('Ctrl Pts',(23.4418758252863,1.39614949199035,-6.87427578780015));
#133340=CARTESIAN_POINT('Ctrl Pts',(23.4545649487095,1.33983891959706,-6.87719525329033));
#133341=CARTESIAN_POINT('Ctrl Pts',(23.4672518996907,1.28353798785837,-6.88011421895326));
#133342=CARTESIAN_POINT('Ctrl Pts',(23.4768158231066,1.22653014248622,-6.88310421089122));
#133343=CARTESIAN_POINT('Ctrl Pts',(23.48319543489,1.16918611634482,-6.88616236731445));
#133344=CARTESIAN_POINT('Ctrl Pts',(23.4895806266956,1.11179193340039,-6.88922319859956));
#133345=CARTESIAN_POINT('Ctrl Pts',(23.4927759120905,1.0540609865502,-6.8923522795552));
#133346=CARTESIAN_POINT('Ctrl Pts',(23.4927545859088,0.996369469660129,
-6.8955221021616));
#133347=CARTESIAN_POINT('Ctrl Pts',(23.4927332500643,0.938651813220718,
-6.89869336098843));
#133348=CARTESIAN_POINT('Ctrl Pts',(23.4894921934945,0.880973587000663,
-6.90190520900859));
#133349=CARTESIAN_POINT('Ctrl Pts',(23.4830409884787,0.823716243544801,
-6.90510708351915));
#133350=CARTESIAN_POINT('Ctrl Pts',(23.4765785699948,0.76635937552023,-6.90831452351985));
#133351=CARTESIAN_POINT('Ctrl Pts',(23.4668943892679,0.709424848678099,
-6.91151154679704));
#133352=CARTESIAN_POINT('Ctrl Pts',(23.4540392373995,0.653301300146426,
-6.91462863265755));
#133353=CARTESIAN_POINT('Ctrl Pts',(23.4456805697153,0.616808686427064,
-6.9166554220038));
#133354=CARTESIAN_POINT('Ctrl Pts',(23.4359820907259,0.580659069910008,
-6.91864801976249));
#133355=CARTESIAN_POINT('Ctrl Pts',(23.4249687810269,0.544960262964138,
-6.92058471113213));
#133356=CARTESIAN_POINT('Ctrl Pts',(23.4249637831682,0.544944062784526,
-6.92058559000599));
#133357=CARTESIAN_POINT('Ctrl Pts',(23.4249587850337,0.544927862679981,
-6.92058646886906));
#133358=CARTESIAN_POINT('Ctrl Pts',(23.4249537866235,0.544911662650505,
-6.92058734772135));
#133359=CARTESIAN_POINT('Ctrl Pts',(23.409568224219,0.495046494521923,-6.92329253521352));
#133360=CARTESIAN_POINT('Ctrl Pts',(23.3915668267523,0.445890046649582,
-6.92589556871675));
#133361=CARTESIAN_POINT('Ctrl Pts',(23.3710580569309,0.397725042837229,
-6.92844794313227));
#133362=CARTESIAN_POINT('Ctrl Pts',(23.3689873456662,0.392861961490763,
-6.92870564900639));
#133363=CARTESIAN_POINT('Ctrl Pts',(23.3668911097967,0.388009011609156,
-6.92896283844364));
#133364=CARTESIAN_POINT('Ctrl Pts',(23.364769485865,0.383166499898504,-6.92921956444747));
#133365=CARTESIAN_POINT('Ctrl Pts',(23.3416666234825,0.33043525004452,-6.93201511433164));
#133366=CARTESIAN_POINT('Ctrl Pts',(23.3155488213821,0.278938233791786,
-6.93475641593523));
#133367=CARTESIAN_POINT('Ctrl Pts',(23.2866046352174,0.229021473990792,
-6.9375035946566));
#133368=CARTESIAN_POINT('Ctrl Pts',(23.2576872709693,0.179150970911703,
-6.94024822763016));
#133369=CARTESIAN_POINT('Ctrl Pts',(23.225949226306,0.130857646564572,-6.94299916427836));
#133370=CARTESIAN_POINT('Ctrl Pts',(23.1916109603711,0.0844565701330748,
-6.94579956288904));
#133371=CARTESIAN_POINT('Ctrl Pts',(23.1572915429672,0.0380809635996349,
-6.94859842433997));
#133372=CARTESIAN_POINT('Ctrl Pts',(23.1203750226841,-0.00640459895006078,
-6.95144692903123));
#133373=CARTESIAN_POINT('Ctrl Pts',(23.0811084900701,-0.0487133903317922,
-6.95436639478018));
#133374=CARTESIAN_POINT('Ctrl Pts',(23.0418486787455,-0.0910149396779262,
-6.95728536080143));
#133375=CARTESIAN_POINT('Ctrl Pts',(23.0002397802386,-0.131140525167259,
-6.96027535313538));
#133376=CARTESIAN_POINT('Ctrl Pts',(22.9565529012732,-0.168829955070649,
-6.9633335098726));
#133377=CARTESIAN_POINT('Ctrl Pts',(22.9128278086591,-0.206552352553033,
-6.96639434163101));
#133378=CARTESIAN_POINT('Ctrl Pts',(22.8670210906049,-0.241834309659026,
-6.96952342298557));
#133379=CARTESIAN_POINT('Ctrl Pts',(22.8194279119882,-0.274441065500062,
-6.97269324578701));
#133380=CARTESIAN_POINT('Ctrl Pts',(22.7718131679043,-0.307062596145898,
-6.97586450490162));
#133381=CARTESIAN_POINT('Ctrl Pts',(22.7224102051567,-0.337006360951613,
-6.9790763530086));
#133382=CARTESIAN_POINT('Ctrl Pts',(22.6715390404077,-0.364064545154381,
-6.9822782272528));
#133383=CARTESIAN_POINT('Ctrl Pts',(22.6205794492212,-0.391169763051821,
-6.98548566713195));
#133384=CARTESIAN_POINT('Ctrl Pts',(22.5681462911772,-0.41537899686547,
-6.98868268993298));
#133385=CARTESIAN_POINT('Ctrl Pts',(22.5145888174665,-0.436514364241684,
-6.99179977477122));
#133386=CARTESIAN_POINT('Ctrl Pts',(22.479764718626,-0.45025698635479,-6.99382656324685));
#133387=CARTESIAN_POINT('Ctrl Pts',(22.44446584951,-0.462700634545866,-6.99581915991031));
#133388=CARTESIAN_POINT('Ctrl Pts',(22.4087952549026,-0.473804944237803,
-6.99775584990608));
#133389=CARTESIAN_POINT('Ctrl Pts',(22.408779067629,-0.473809983360409,
-6.99775672877371));
#133390=CARTESIAN_POINT('Ctrl Pts',(22.4087628802613,-0.473815022213182,
-6.99775760763055));
#133391=CARTESIAN_POINT('Ctrl Pts',(22.4087466927996,-0.47382006079611,
-6.99775848647662));
#133392=CARTESIAN_POINT('Ctrl Pts',(22.3589199269531,-0.48932936652176,
-7.0004636701555));
#133393=CARTESIAN_POINT('Ctrl Pts',(22.3081984348818,-0.502280486332587,
-7.00306669948927));
#133394=CARTESIAN_POINT('Ctrl Pts',(22.2568767273539,-0.512602995713214,
-7.00561906908348));
#133395=CARTESIAN_POINT('Ctrl Pts',(22.2516948146702,-0.513645251414825,
-7.00587677984586));
#133396=CARTESIAN_POINT('Ctrl Pts',(22.2465068235975,-0.514660725305008,
-7.0061339741432));
#133397=CARTESIAN_POINT('Ctrl Pts',(22.2413130843257,-0.515649356552682,
-7.00639070498193));
#133398=CARTESIAN_POINT('Ctrl Pts',(22.1847583086682,-0.526414590518925,
-7.00918625443655));
#133399=CARTESIAN_POINT('Ctrl Pts',(22.127516529053,-0.533995289840677,
-7.01192755471752));
#133400=CARTESIAN_POINT('Ctrl Pts',(22.0699797563789,-0.538351291058253,
-7.01467473145523));
#133401=CARTESIAN_POINT('Ctrl Pts',(22.0124963031947,-0.542703255557179,
-7.01741936237649));
#133402=CARTESIAN_POINT('Ctrl Pts',(21.9547185440105,-0.543836966660925,
-7.02017029631679));
#133403=CARTESIAN_POINT('Ctrl Pts',(21.8970310019311,-0.541756077642057,
-7.02297069195622));
#133404=CARTESIAN_POINT('Ctrl Pts',(21.8393751265965,-0.539676330897219,
-7.02576955035883));
#133405=CARTESIAN_POINT('Ctrl Pts',(21.7818094141064,-0.534385802431919,
-7.02861805173894));
#133406=CARTESIAN_POINT('Ctrl Pts',(21.7247100723998,-0.525926137154944,
-7.0315375144116));
#133407=CARTESIAN_POINT('Ctrl Pts',(21.6676205061858,-0.517467920185284,
-7.03445647726788));
#133408=CARTESIAN_POINT('Ctrl Pts',(21.6109971680635,-0.505841786149631,
-7.03744646666923));
#133409=CARTESIAN_POINT('Ctrl Pts',(21.5552079618626,-0.491124193051166,
-7.04050462127644));
#133410=CARTESIAN_POINT('Ctrl Pts',(21.4993699590489,-0.476393727055949,
-7.04356545073055));
#133411=CARTESIAN_POINT('Ctrl Pts',(21.4443675607246,-0.45856637310289,
-7.04669453057846));
#133412=CARTESIAN_POINT('Ctrl Pts',(21.3905613013614,-0.437752812222422,
-7.04986435329719));
#133413=CARTESIAN_POINT('Ctrl Pts',(21.3367306628793,-0.416929820909862,
-7.05303561223331));
#133414=CARTESIAN_POINT('Ctrl Pts',(21.2840972842237,-0.393117722594224,
-7.05624746158659));
#133415=CARTESIAN_POINT('Ctrl Pts',(21.233013529593,-0.366462932744109,
-7.05944933916246));
#133416=CARTESIAN_POINT('Ctrl Pts',(21.1818409821029,-0.339761812019858,
-7.06265678218408));
#133417=CARTESIAN_POINT('Ctrl Pts',(21.1322236049285,-0.310207692293406,
-7.06585381022509));
#133418=CARTESIAN_POINT('Ctrl Pts',(21.0845056074429,-0.277988026804604,
-7.06897090306744));
#133419=CARTESIAN_POINT('Ctrl Pts',(21.0534789061002,-0.25703849012744,
-7.07099766684156));
#133420=CARTESIAN_POINT('Ctrl Pts',(21.0232550309494,-0.234962852301261,
-7.07299024097854));
#133421=CARTESIAN_POINT('Ctrl Pts',(20.9939255402615,-0.21182327068612,
-7.07492691175894));
#133422=CARTESIAN_POINT('Ctrl Pts',(20.9939122314531,-0.211812770665437,
-7.07492779055976));
#133423=CARTESIAN_POINT('Ctrl Pts',(20.9938989228132,-0.211802270414054,
-7.07492866934983));
#133424=CARTESIAN_POINT('Ctrl Pts',(20.9938856143419,-0.211791769931971,
-7.07492954812917));
#133425=CARTESIAN_POINT('Ctrl Pts',(20.9531641999186,-0.179662273484807,
-7.07761844729391));
#133426=CARTESIAN_POINT('Ctrl Pts',(20.9140198227237,-0.145368622016484,
-7.0802067852082));
#133427=CARTESIAN_POINT('Ctrl Pts',(20.876677017731,-0.109110200271477,
-7.08274496610853));
#133428=CARTESIAN_POINT('Ctrl Pts',(20.8724589226394,-0.105014592809239,
-7.0830316689526));
#133429=CARTESIAN_POINT('Ctrl Pts',(20.8682638249325,-0.100893970305654,
-7.08331773184006));
#133430=CARTESIAN_POINT('Ctrl Pts',(20.8640920555125,-0.0967486611347506,
-7.08360322741416));
#133431=CARTESIAN_POINT('Ctrl Pts',(20.8236204324131,-0.0565337370805138,
-7.08637290812002));
#133432=CARTESIAN_POINT('Ctrl Pts',(20.7853427847753,-0.0139899011780043,
-7.08908987158476));
#133433=CARTESIAN_POINT('Ctrl Pts',(20.7495112547215,0.0305884202616647,
-7.09181249410042));
#133434=CARTESIAN_POINT('Ctrl Pts',(20.7137122859447,0.0751262319305429,
-7.09453264248044));
#133435=CARTESIAN_POINT('Ctrl Pts',(20.6803547176496,0.12169444025125,-7.09725886511378));
#133436=CARTESIAN_POINT('Ctrl Pts',(20.6496504682484,0.169979289696589,
-7.10003321935231));
#133437=CARTESIAN_POINT('Ctrl Pts',(20.6189619168207,0.218239452842812,
-7.10280615516375));
#133438=CARTESIAN_POINT('Ctrl Pts',(20.5909237821157,0.26821427989406,-7.10562740367482));
#133439=CARTESIAN_POINT('Ctrl Pts',(20.5657116524017,0.31957489765083,-7.10851795047218));
#133440=CARTESIAN_POINT('Ctrl Pts',(20.5397449316027,0.3724727224869,-7.11149501042289));
#133441=CARTESIAN_POINT('Ctrl Pts',(20.5167759968454,0.4268404724139,-7.11454579998516));
#133442=CARTESIAN_POINT('Ctrl Pts',(20.4969590545714,0.482304349981721,
-7.117667332509));
#133443=CARTESIAN_POINT('Ctrl Pts',(20.4777036213231,0.536196669867898,
-7.12070041704414));
#133444=CARTESIAN_POINT('Ctrl Pts',(20.4614239473617,0.591123785151236,
-7.1238001322834));
#133445=CARTESIAN_POINT('Ctrl Pts',(20.4482274795238,0.646730635327404,
-7.1269396055833));
#133446=CARTESIAN_POINT('Ctrl Pts',(20.4344537770139,0.704769818331229,
-7.13021640448148));
#133447=CARTESIAN_POINT('Ctrl Pts',(20.4240393927185,0.763549646139969,
-7.13353646981584));
#133448=CARTESIAN_POINT('Ctrl Pts',(20.4170658700461,0.822652418007863,
-7.1368436453435));
#133449=CARTESIAN_POINT('Ctrl Pts',(20.4105353527739,0.878000581433825,
-7.13994072667823));
#133450=CARTESIAN_POINT('Ctrl Pts',(20.4070225510227,0.9336325600701,-7.14302605898205));
#133451=CARTESIAN_POINT('Ctrl Pts',(20.4065569725966,0.989191189421772,
-7.14603652038649));
#133452=CARTESIAN_POINT('Ctrl Pts',(20.4065253895308,0.992960075069953,
-7.1462407386135));
#133453=CARTESIAN_POINT('Ctrl Pts',(20.4065078194293,0.996728640647018,
-7.14644461230347));
#133454=CARTESIAN_POINT('Ctrl Pts',(20.4065042675225,1.00049678240474,-7.14664812175195));
#133455=CARTESIAN_POINT('Ctrl Pts',(20.4070000539504,1.00048100217607,-7.14693314283738));
#133456=CARTESIAN_POINT('Ctrl Pts',(20.4070043911558,1.01439426051975,-7.1476949496416));
#133457=CARTESIAN_POINT('Ctrl Pts',(20.407196912604,1.02830727097016,-7.14845039496485));
#133458=CARTESIAN_POINT('Ctrl Pts',(20.4079245187433,1.05489128412844,-7.14987943904459));
#133459=CARTESIAN_POINT('Ctrl Pts',(20.4084276730568,1.06756199170956,-7.15055429935513));
#133460=CARTESIAN_POINT('Ctrl Pts',(20.4098781160518,1.09542107250405,-7.15202227234891));
#133461=CARTESIAN_POINT('Ctrl Pts',(20.4108939396218,1.11060366610524,-7.15281144404058));
#133462=CARTESIAN_POINT('Ctrl Pts',(20.4139675239172,1.1481860864981,-7.15473853162009));
#133463=CARTESIAN_POINT('Ctrl Pts',(20.4162906839258,1.17056000144823,-7.15586353571352));
#133464=CARTESIAN_POINT('Ctrl Pts',(20.428221908484,1.26526058343634,-7.16055938457115));
#133465=CARTESIAN_POINT('Ctrl Pts',(20.4424645642558,1.33691282787775,-7.16395161044413));
#133466=CARTESIAN_POINT('Ctrl Pts',(20.486812221479,1.49896218641207,-7.171735707453));
#133467=CARTESIAN_POINT('Ctrl Pts',(20.5203145467133,1.58811568222157,-7.17611228865077));
#133468=CARTESIAN_POINT('Ctrl Pts',(20.5775637714579,1.70609576792949,-7.18248265732038));
#133469=CARTESIAN_POINT('Ctrl Pts',(20.5944589210291,1.73801123191433,-7.18426702960988));
#133470=CARTESIAN_POINT('Ctrl Pts',(20.6264530411218,1.79363753481879,-7.18750492596221));
#133471=CARTESIAN_POINT('Ctrl Pts',(20.641109876985,1.81758400588174,-7.18894307646896));
#133472=CARTESIAN_POINT('Ctrl Pts',(20.6752139039797,1.87003404101473,-7.19219913200481));
#133473=CARTESIAN_POINT('Ctrl Pts',(20.6949799735352,1.89831136945066,-7.19402780813477));
#133474=CARTESIAN_POINT('Ctrl Pts',(20.760025369074,1.98502373309913,-7.19987446489188));
#133475=CARTESIAN_POINT('Ctrl Pts',(20.8085610868534,2.04087786893519,-7.20400382444038));
#133476=CARTESIAN_POINT('Ctrl Pts',(20.9260377573493,2.15793083873767,-7.21340732637559));
#133477=CARTESIAN_POINT('Ctrl Pts',(20.996839496075,2.21687649802452,-7.21869957929475));
#133478=CARTESIAN_POINT('Ctrl Pts',(21.093578709451,2.28376409378472,-7.22515581461593));
#133479=CARTESIAN_POINT('Ctrl Pts',(21.1150501889081,2.29783150945306,-7.22654367599907));
#133480=CARTESIAN_POINT('Ctrl Pts',(21.1507059531751,2.31994065801378,-7.22876351807761));
#133481=CARTESIAN_POINT('Ctrl Pts',(21.1646835567014,2.32830435881413,-7.22961279108647));
#133482=CARTESIAN_POINT('Ctrl Pts',(21.1968941645141,2.34689175921865,-7.23152070578121));
#133483=CARTESIAN_POINT('Ctrl Pts',(21.2152069359682,2.3569690649454,-7.23257141180791));
#133484=CARTESIAN_POINT('Ctrl Pts',(21.330729481491,2.4175150867158,-7.23902375517673));
#133485=CARTESIAN_POINT('Ctrl Pts',(21.4328864049288,2.45789000708564,-7.24398205208198));
#133486=CARTESIAN_POINT('Ctrl Pts',(21.5877825352006,2.50075510905614,-7.25145444036878));
#133487=CARTESIAN_POINT('Ctrl Pts',(21.6377455394643,2.51194053415837,-7.25385495133468));
#133488=CARTESIAN_POINT('Ctrl Pts',(21.7284574103357,2.52755984617057,-7.25828065783118));
#133489=CARTESIAN_POINT('Ctrl Pts',(21.7690022432529,2.5328925879683,-7.26028219069691));
#133490=CARTESIAN_POINT('Ctrl Pts',(21.8380335002001,2.5391950696334,-7.26375619811298));
#133491=CARTESIAN_POINT('Ctrl Pts',(21.8664226439939,2.54099729167704,-7.26520356024424));
#133492=CARTESIAN_POINT('Ctrl Pts',(21.9265847735143,2.5431492069447,-7.26831680433476));
#133493=CARTESIAN_POINT('Ctrl Pts',(21.9583510938058,2.54330418833115,-7.26998775709018));
#133494=CARTESIAN_POINT('Ctrl Pts',(22.0531076809942,2.54084090078519,-7.27505765183627));
#133495=CARTESIAN_POINT('Ctrl Pts',(22.1159519210039,2.53534379580097,-7.27853586058876));
#133496=CARTESIAN_POINT('Ctrl Pts',(22.2756294975527,2.5114574332279,-7.28761557897988));
#133497=CARTESIAN_POINT('Ctrl Pts',(22.3713598290015,2.4876133666492,-7.2933017009994));
#133498=CARTESIAN_POINT('Ctrl Pts',(22.4954884057359,2.44374342304794,-7.30062487629376));
#133499=CARTESIAN_POINT('Ctrl Pts',(22.5264478703202,2.43166364364086,-7.30244512223817));
#133500=CARTESIAN_POINT('Ctrl Pts',(22.5728997393109,2.41178757881728,-7.30514245397109));
#133501=CARTESIAN_POINT('Ctrl Pts',(22.5886900177701,2.40471470046022,-7.30605319238636));
#133502=CARTESIAN_POINT('Ctrl Pts',(22.6209306996614,2.3896171445202,-7.30789516424898));
#133503=CARTESIAN_POINT('Ctrl Pts',(22.6373637520081,2.38156250015455,-7.30882474280428));
#133504=CARTESIAN_POINT('Ctrl Pts',(22.6894322662673,2.35488206608178,-7.31175195686221));
#133505=CARTESIAN_POINT('Ctrl Pts',(22.7244862699264,2.33515426687521,-7.31369512460448));
#133506=CARTESIAN_POINT('Ctrl Pts',(22.8038542486379,2.2863083304854,-7.31811685197965));
#133507=CARTESIAN_POINT('Ctrl Pts',(22.847497344002,2.25624438587793,-7.32056596815938));
#133508=CARTESIAN_POINT('Ctrl Pts',(22.889491673488,2.22401158325724,-7.32301705809308));
#133509=CARTESIAN_POINT('',(20.4070004162552,0.998856448297238,-7.10475668005849));
#133510=CARTESIAN_POINT('Ctrl Pts',(22.8894915988056,2.22401164057974,-7.28231538991332));
#133511=CARTESIAN_POINT('Ctrl Pts',(22.8845521534573,2.22780291784992,-7.28201294331082));
#133512=CARTESIAN_POINT('Ctrl Pts',(22.8795889774586,2.23156489550419,-7.2817095323024));
#133513=CARTESIAN_POINT('Ctrl Pts',(22.847518386252,2.25556927291874,-7.27975172234917));
#133514=CARTESIAN_POINT('Ctrl Pts',(22.8197764516961,2.27494398920208,-7.27807039357847));
#133515=CARTESIAN_POINT('Ctrl Pts',(22.7678965287784,2.30869471919725,-7.27493424659343));
#133516=CARTESIAN_POINT('Ctrl Pts',(22.7439596224551,2.32335353945117,-7.27349029773104));
#133517=CARTESIAN_POINT('Ctrl Pts',(22.6877197826458,2.35571922192614,-7.2700991669245));
#133518=CARTESIAN_POINT('Ctrl Pts',(22.6551569074382,2.37293792112831,-7.26813656518618));
#133519=CARTESIAN_POINT('Ctrl Pts',(22.5829802384274,2.40785829621056,-7.26378668078137));
#133520=CARTESIAN_POINT('Ctrl Pts',(22.5431731816798,2.42508741940847,-7.2613875777753));
#133521=CARTESIAN_POINT('Ctrl Pts',(22.3918745258154,2.48313345571084,-7.25229932018913));
#133522=CARTESIAN_POINT('Ctrl Pts',(22.2765227071108,2.51271940634196,-7.24539632296005));
#133523=CARTESIAN_POINT('Ctrl Pts',(22.1346929324414,2.53210167666293,-7.23755978498624));
#133524=CARTESIAN_POINT('Ctrl Pts',(22.1103868020574,2.53483654670601,-7.2362407854107));
#133525=CARTESIAN_POINT('Ctrl Pts',(22.0699147763377,2.53841834537676,-7.23409516525903));
#133526=CARTESIAN_POINT('Ctrl Pts',(22.0537834117036,2.5395907328649,-7.2332537102185));
#133527=CARTESIAN_POINT('Ctrl Pts',(22.0160523422047,2.54173713380429,-7.23131853736766));
#133528=CARTESIAN_POINT('Ctrl Pts',(21.9944455685431,2.54251125812968,-7.23023437542709));
#133529=CARTESIAN_POINT('Ctrl Pts',(21.9465009345402,2.54322067734371,-7.22786853579623));
#133530=CARTESIAN_POINT('Ctrl Pts',(21.9201664354746,2.54293628292467,-7.22659568585361));
#133531=CARTESIAN_POINT('Ctrl Pts',(21.8337807617944,2.53979067647612,-7.22247311583009));
#133532=CARTESIAN_POINT('Ctrl Pts',(21.7738872481558,2.53409487411891,-7.21969710898256));
#133533=CARTESIAN_POINT('Ctrl Pts',(21.6293358048462,2.51176897379883,-7.2129251630867));
#133534=CARTESIAN_POINT('Ctrl Pts',(21.5454489901307,2.49151204561127,-7.20892673403416));
#133535=CARTESIAN_POINT('Ctrl Pts',(21.4304439485781,2.45331970299062,-7.20302424726479));
#133536=CARTESIAN_POINT('Ctrl Pts',(21.3975795635323,2.44114818497966,-7.20128829740587));
#133537=CARTESIAN_POINT('Ctrl Pts',(21.339229658987,2.41724865750151,-7.1981009189788));
#133538=CARTESIAN_POINT('Ctrl Pts',(21.3135952965397,2.40592428453362,-7.19666279535045));
#133539=CARTESIAN_POINT('Ctrl Pts',(21.2563222745226,2.37873566840239,-7.19335746594781));
#133540=CARTESIAN_POINT('Ctrl Pts',(21.2248932823828,2.3624686500678,-7.19147767220279));
#133541=CARTESIAN_POINT('Ctrl Pts',(21.1585368424642,2.32517729039153,-7.18736236635965));
#133542=CARTESIAN_POINT('Ctrl Pts',(21.1238274549572,2.30382029918256,-7.18511759622543));
#133543=CARTESIAN_POINT('Ctrl Pts',(21.0094425457237,2.2270353756561,-7.17742075223178));
#133544=CARTESIAN_POINT('Ctrl Pts',(20.9341652709363,2.16547954528211,-7.17182521054017));
#133545=CARTESIAN_POINT('Ctrl Pts',(20.8365114712754,2.06893233229076,-7.16411099494136));
#133546=CARTESIAN_POINT('Ctrl Pts',(20.8089731332872,2.03948599251083,-7.16187772940895));
#133547=CARTESIAN_POINT('Ctrl Pts',(20.7701502146398,1.99456877543557,-7.15868092404283));
#133548=CARTESIAN_POINT('Ctrl Pts',(20.7579504382081,1.97991350308562,-7.15766873883154));
#133549=CARTESIAN_POINT('Ctrl Pts',(20.7355219492455,1.95193178733353,-7.15579926067446));
#133550=CARTESIAN_POINT('Ctrl Pts',(20.7252336620435,1.93865781349616,-7.15493863562881));
#133551=CARTESIAN_POINT('Ctrl Pts',(20.6972397547846,1.90129594063933,-7.15258127533428));
#133552=CARTESIAN_POINT('Ctrl Pts',(20.6800135590714,1.87685645464419,-7.15111206340992));
#133553=CARTESIAN_POINT('Ctrl Pts',(20.6399169138774,1.81630688266772,-7.14760704139548));
#133554=CARTESIAN_POINT('Ctrl Pts',(20.6178152417466,1.77971706097726,-7.14559999690437));
#133555=CARTESIAN_POINT('Ctrl Pts',(20.5412923362039,1.6402562397643,-7.1381936448793));
#133556=CARTESIAN_POINT('Ctrl Pts',(20.4970433166301,1.53226058919941,-7.13289999536883));
#133557=CARTESIAN_POINT('Ctrl Pts',(20.4560352108718,1.38741181727617,-7.12555046086082));
#133558=CARTESIAN_POINT('Ctrl Pts',(20.4478160809911,1.35420611659052,-7.12385242583675));
#133559=CARTESIAN_POINT('Ctrl Pts',(20.4349336714764,1.29358895426854,-7.12071470938939));
#133560=CARTESIAN_POINT('Ctrl Pts',(20.4298948956972,1.26627204453838,-7.11928706560123));
#133561=CARTESIAN_POINT('Ctrl Pts',(20.4214036547572,1.21207531645098,-7.11642319191832));
#133562=CARTESIAN_POINT('Ctrl Pts',(20.4179166107863,1.18521095877565,-7.11498855704211));
#133563=CARTESIAN_POINT('Ctrl Pts',(20.4096768020266,1.10530330344337,-7.11067492792935));
#133564=CARTESIAN_POINT('Ctrl Pts',(20.4069609369192,1.05209452824687,-7.10774097361327));
#133565=CARTESIAN_POINT('Ctrl Pts',(20.4070004029467,0.998856162050184,
-7.10475668494137));
#133566=CARTESIAN_POINT('Ctrl Pts',(20.4070004027354,0.998856447117781,
-7.1047567009209));
#133567=CARTESIAN_POINT('Ctrl Pts',(20.4070509525418,0.9306494309019,-7.1009333413968));
#133568=CARTESIAN_POINT('Ctrl Pts',(20.4116240317839,0.862522408636186,
-7.09703298057708));
#133569=CARTESIAN_POINT('Ctrl Pts',(20.4262633056739,0.753352816772122,
-7.09077819504367));
#133570=CARTESIAN_POINT('Ctrl Pts',(20.4335309269496,0.712024010642907,
-7.08841037679596));
#133571=CARTESIAN_POINT('Ctrl Pts',(20.4487726883061,0.642175256369573,
-7.08445610803221));
#133572=CARTESIAN_POINT('Ctrl Pts',(20.4558997436795,0.613494358933053,
-7.08284653533944));
#133573=CARTESIAN_POINT('Ctrl Pts',(20.468349154306,0.568908175950438,-7.0803843563375));
#133574=CARTESIAN_POINT('Ctrl Pts',(20.4731143669726,0.552855390044602,
-7.07950627917967));
#133575=CARTESIAN_POINT('Ctrl Pts',(20.4838952644542,0.518592061803567,
-7.07765407945101));
#133576=CARTESIAN_POINT('Ctrl Pts',(20.4899908035707,0.500410258706161,
-7.07668394218358));
#133577=CARTESIAN_POINT('Ctrl Pts',(20.510185875544,0.443702353444211,-7.07368512557166));
#133578=CARTESIAN_POINT('Ctrl Pts',(20.5254842771696,0.405620360842853,
-7.071710668315));
#133579=CARTESIAN_POINT('Ctrl Pts',(20.5768797550957,0.291107417325853,
-7.06577414664544));
#133580=CARTESIAN_POINT('Ctrl Pts',(20.617749939527,0.216993945476465,-7.06192599283445));
#133581=CARTESIAN_POINT('Ctrl Pts',(20.7004798554822,0.0923743172461711,
-7.05493606753585));
#133582=CARTESIAN_POINT('Ctrl Pts',(20.7398687909791,0.040486334191363,
-7.0518437130033));
#133583=CARTESIAN_POINT('Ctrl Pts',(20.8028326728216,-0.0323912474073396,
-7.04709530335299));
#133584=CARTESIAN_POINT('Ctrl Pts',(20.8239637528491,-0.0553988669875149,
-7.04553045741632));
#133585=CARTESIAN_POINT('Ctrl Pts',(20.8657220878292,-0.0981829553572622,
-7.04248109803501));
#133586=CARTESIAN_POINT('Ctrl Pts',(20.8862290540689,-0.118058867736983,
-7.04100182502386));
#133587=CARTESIAN_POINT('Ctrl Pts',(20.9383559252877,-0.165848753205058,
-7.03728038176894));
#133588=CARTESIAN_POINT('Ctrl Pts',(20.9705899017304,-0.193055943279883,
-7.03501195960825));
#133589=CARTESIAN_POINT('Ctrl Pts',(21.0936050258876,-0.288539093483138,
-7.02647505636288));
#133590=CARTESIAN_POINT('Ctrl Pts',(21.1907230058785,-0.348050194545007,
-7.01993246464822));
#133591=CARTESIAN_POINT('Ctrl Pts',(21.3243259083336,-0.410866099597751,
-7.011596241665));
#133592=CARTESIAN_POINT('Ctrl Pts',(21.3556506367177,-0.424345550700895,
-7.00968819907164));
#133593=CARTESIAN_POINT('Ctrl Pts',(21.4114278316744,-0.446186380588833,
-7.00639883959606));
#133594=CARTESIAN_POINT('Ctrl Pts',(21.4356919064804,-0.454992217573493,
-7.00500276792051));
#133595=CARTESIAN_POINT('Ctrl Pts',(21.4754759321275,-0.468310787723789,
-7.00278232797752));
#133596=CARTESIAN_POINT('Ctrl Pts',(21.4908650874757,-0.473195460255269,
-7.00194012234738));
#133597=CARTESIAN_POINT('Ctrl Pts',(21.5261146013529,-0.483777916261725,
-7.0000508846564));
#133598=CARTESIAN_POINT('Ctrl Pts',(21.5460175944571,-0.489319988870331,
-6.99901155844509));
#133599=CARTESIAN_POINT('Ctrl Pts',(21.6735683421865,-0.522091719025388,
-6.99249103803639));
#133600=CARTESIAN_POINT('Ctrl Pts',(21.7837887111138,-0.538036552840913,
-6.98746920792789));
#133601=CARTESIAN_POINT('Ctrl Pts',(21.945419728441,-0.543825203860573,
-6.97994681118554));
#133602=CARTESIAN_POINT('Ctrl Pts',(21.9961217408377,-0.543142788714532,
-6.9775679413078));
#133603=CARTESIAN_POINT('Ctrl Pts',(22.0872402683269,-0.537421343486204,
-6.97317628028501));
#133604=CARTESIAN_POINT('Ctrl Pts',(22.1276654537821,-0.533275559687159,
-6.97118650990352));
#133605=CARTESIAN_POINT('Ctrl Pts',(22.195974581872,-0.523532395917599,
-6.96772754909587));
#133606=CARTESIAN_POINT('Ctrl Pts',(22.2239537962885,-0.518750684793128,
-6.96628297967836));
#133607=CARTESIAN_POINT('Ctrl Pts',(22.2829535253383,-0.506984109268314,
-6.96317116043018));
#133608=CARTESIAN_POINT('Ctrl Pts',(22.3139217498944,-0.499806629533253,
-6.96149869766345));
#133609=CARTESIAN_POINT('Ctrl Pts',(22.4094051788206,-0.474545117238194,
-6.95621489133463));
#133610=CARTESIAN_POINT('Ctrl Pts',(22.4729748481352,-0.453214447024215,
-6.95251021870147));
#133611=CARTESIAN_POINT('Ctrl Pts',(22.6098273250283,-0.397148542494041,
-6.94417563933477));
#133612=CARTESIAN_POINT('Ctrl Pts',(22.6821713982143,-0.360632524233955,
-6.93952423402196));
#133613=CARTESIAN_POINT('Ctrl Pts',(22.7875780215223,-0.296577189991489,
-6.93259221955281));
#133614=CARTESIAN_POINT('Ctrl Pts',(22.8229167152729,-0.273053899500617,
-6.93024082535303));
#133615=CARTESIAN_POINT('Ctrl Pts',(22.8722546767471,-0.237190245306591,
-6.92696355518505));
#133616=CARTESIAN_POINT('Ctrl Pts',(22.8870691493192,-0.22600769248049,
-6.92598034644523));
#133617=CARTESIAN_POINT('Ctrl Pts',(22.9151152446012,-0.204031935546696,
-6.9241262809822));
#133618=CARTESIAN_POINT('Ctrl Pts',(22.9283760894639,-0.19328143437829,
-6.92325334198535));
#133619=CARTESIAN_POINT('Ctrl Pts',(22.9658106850263,-0.161889779435671,
-6.92079173926943));
#133620=CARTESIAN_POINT('Ctrl Pts',(22.9895298441754,-0.140717817380733,
-6.91923506165352));
#133621=CARTESIAN_POINT('Ctrl Pts',(23.0911481809923,-0.044208231348577,
-6.91249658121761));
#133622=CARTESIAN_POINT('Ctrl Pts',(23.1616420068988,0.0384822650013561,
-6.90761411827222));
#133623=CARTESIAN_POINT('Ctrl Pts',(23.246756380588,0.162710095104583,-6.9005460540303));
#133624=CARTESIAN_POINT('Ctrl Pts',(23.2691791378977,0.198502881308005,
-6.89853939020893));
#133625=CARTESIAN_POINT('Ctrl Pts',(23.3080501397243,0.266611017828464,
-6.89473105156451));
#133626=CARTESIAN_POINT('Ctrl Pts',(23.324881975976,0.298673476871123,-6.8929422353621));
#133627=CARTESIAN_POINT('Ctrl Pts',(23.3526077823798,0.35632936563645,-6.88971494453106));
#133628=CARTESIAN_POINT('Ctrl Pts',(23.363966873702,0.381681285425901,-6.88829249959763));
#133629=CARTESIAN_POINT('Ctrl Pts',(23.3877593496193,0.438872153847334,
-6.8850705269798));
#133630=CARTESIAN_POINT('Ctrl Pts',(23.3998313437624,0.470844778175845,
-6.88326037270658));
#133631=CARTESIAN_POINT('Ctrl Pts',(23.4481802805556,0.613011181954941,
-6.87516754162936));
#133632=CARTESIAN_POINT('Ctrl Pts',(23.4730219262029,0.726682765747686,
-6.86854534014066));
#133633=CARTESIAN_POINT('Ctrl Pts',(23.4892942074949,0.884804194948909,
-6.8595146124425));
#133634=CARTESIAN_POINT('Ctrl Pts',(23.4919060433311,0.927731286423592,
-6.85708569865248));
#133635=CARTESIAN_POINT('Ctrl Pts',(23.4932915484781,1.00071371423795,-6.85304514358394));
#133636=CARTESIAN_POINT('Ctrl Pts',(23.4929858694857,1.03072662701455,-6.85140919309752));
#133637=CARTESIAN_POINT('Ctrl Pts',(23.4911436940628,1.07750853433028,-6.84891771520969));
#133638=CARTESIAN_POINT('Ctrl Pts',(23.4902078937249,1.09429309963478,-6.84803571898826));
#133639=CARTESIAN_POINT('Ctrl Pts',(23.4876280856383,1.13004226184516,-6.84618660210858));
#133640=CARTESIAN_POINT('Ctrl Pts',(23.4859071600779,1.14899791642161,-6.84522311585918));
#133641=CARTESIAN_POINT('Ctrl Pts',(23.479474269024,1.20775884398913,-6.84227644125621));
#133642=CARTESIAN_POINT('Ctrl Pts',(23.473561702995,1.24741747635017,-6.84034479976302));
#133643=CARTESIAN_POINT('Ctrl Pts',(23.4480334903751,1.38236585902902,-6.8338413094117));
#133644=CARTESIAN_POINT('Ctrl Pts',(23.4209611034105,1.47600689798692,-6.82943545975346));
#133645=CARTESIAN_POINT('Ctrl Pts',(23.3702843743358,1.60440350326869,-6.8229424583509));
#133646=CARTESIAN_POINT('Ctrl Pts',(23.3538191453811,1.64171867508635,-6.82099968666875));
#133647=CARTESIAN_POINT('Ctrl Pts',(23.3203343354426,1.71013082681355,-6.81729327346647));
#133648=CARTESIAN_POINT('Ctrl Pts',(23.3036837939901,1.74137840638692,-6.81554097997366));
#133649=CARTESIAN_POINT('Ctrl Pts',(23.2719551874492,1.79628417773131,-6.81233757809382));
#133650=CARTESIAN_POINT('Ctrl Pts',(23.2572786000605,1.82015641473043,-6.81090049815251));
#133651=CARTESIAN_POINT('Ctrl Pts',(23.2228160068598,1.87293442718122,-6.80761639848175));
#133652=CARTESIAN_POINT('Ctrl Pts',(23.2026797895514,1.90159203501022,-6.80575750412412));
#133653=CARTESIAN_POINT('Ctrl Pts',(23.1310769007845,1.99646190582334,-6.79933729399077));
#133654=CARTESIAN_POINT('Ctrl Pts',(23.0752007641256,2.05915043571072,-6.79462402470615));
#133655=CARTESIAN_POINT('Ctrl Pts',(22.9747719206674,2.15486177791452,-6.7867353945752));
#133656=CARTESIAN_POINT('Ctrl Pts',(22.933037559065,2.19058788550244,-6.78359930739587));
#133657=CARTESIAN_POINT('Ctrl Pts',(22.8894916066884,2.22401163452936,-6.78051560659813));
#133658=CARTESIAN_POINT('Origin',(21.9499999789786,0.999999999999992,-4.89578827641128));
#133659=CARTESIAN_POINT('',(22.8894915905204,2.22401164693913,-6.28210119346687));
#133660=CARTESIAN_POINT('',(22.8895004346677,2.22400481472634,-6.32268402640472));
#133661=CARTESIAN_POINT('',(22.8894916101512,2.22401163187148,-4.89578827641128));
#133662=CARTESIAN_POINT('',(20.4070005050181,0.998725889518171,-6.10421116894535));
#133663=CARTESIAN_POINT('Ctrl Pts',(22.8894915905204,2.22401164693913,-6.28210119346687));
#133664=CARTESIAN_POINT('Ctrl Pts',(22.8600553989009,2.2466054312151,-6.28033339624786));
#133665=CARTESIAN_POINT('Ctrl Pts',(22.8298085810512,2.26813397574543,-6.27853880379917));
#133666=CARTESIAN_POINT('Ctrl Pts',(22.7727444074889,2.30572384812454,-6.27516745510784));
#133667=CARTESIAN_POINT('Ctrl Pts',(22.7461660072385,2.3220978228453,-6.27360266342571));
#133668=CARTESIAN_POINT('Ctrl Pts',(22.6941902911137,2.3519822829555,-6.27054290319535));
#133669=CARTESIAN_POINT('Ctrl Pts',(22.6688757747584,2.36561076662804,-6.26905281247638));
#133670=CARTESIAN_POINT('Ctrl Pts',(22.6048225541322,2.39782019571297,-6.26527767352184));
#133671=CARTESIAN_POINT('Ctrl Pts',(22.565662336875,2.41550461754234,-6.26296501168263));
#133672=CARTESIAN_POINT('Ctrl Pts',(22.428894249053,2.47051806277432,-6.25487651315597));
#133673=CARTESIAN_POINT('Ctrl Pts',(22.3282672992176,2.49955775718204,-6.24888450310819));
#133674=CARTESIAN_POINT('Ctrl Pts',(22.1722764493203,2.52786363154342,-6.23991046985082));
#133675=CARTESIAN_POINT('Ctrl Pts',(22.1185865032598,2.5347160902759,-6.23688159576919));
#133676=CARTESIAN_POINT('Ctrl Pts',(22.0446773188154,2.54022274430607,-6.23287971266383));
#133677=CARTESIAN_POINT('Ctrl Pts',(22.0246821453628,2.5413216889432,-6.23181389362117));
#133678=CARTESIAN_POINT('Ctrl Pts',(21.9878240333186,2.54262843759522,-6.22988690615916));
#133679=CARTESIAN_POINT('Ctrl Pts',(21.9709692550235,2.54294959511889,-6.22902086504839));
#133680=CARTESIAN_POINT('Ctrl Pts',(21.9252084244684,2.54307155076537,-6.22670426894211));
#133681=CARTESIAN_POINT('Ctrl Pts',(21.8963066504455,2.54233642118829,-6.2252782296859));
#133682=CARTESIAN_POINT('Ctrl Pts',(21.8270408353905,2.53862500956103,-6.22191554811223));
#133683=CARTESIAN_POINT('Ctrl Pts',(21.7867395678952,2.53487203895624,-6.22000372970443));
#133684=CARTESIAN_POINT('Ctrl Pts',(21.6235471981066,2.51317382521763,-6.21229659923492));
#133685=CARTESIAN_POINT('Ctrl Pts',(21.502896670471,2.48201357631916,-6.20663635098878));
#133686=CARTESIAN_POINT('Ctrl Pts',(21.3574350097396,2.42504154761335,-6.1989408578269));
#133687=CARTESIAN_POINT('Ctrl Pts',(21.3279587438811,2.41242386796144,-6.19733624205496));
#133688=CARTESIAN_POINT('Ctrl Pts',(21.2728115453115,2.38675619606742,-6.19423587548501));
#133689=CARTESIAN_POINT('Ctrl Pts',(21.2470710311032,2.3738877969212,-6.19274645174937));
#133690=CARTESIAN_POINT('Ctrl Pts',(21.1849736159429,2.3406415323837,-6.18904272977856));
#133691=CARTESIAN_POINT('Ctrl Pts',(21.1490549929924,2.3194967891154,-6.18680390040954));
#133692=CARTESIAN_POINT('Ctrl Pts',(21.0699299863074,2.2684950233314,-6.18164967455186));
#133693=CARTESIAN_POINT('Ctrl Pts',(21.0273037886067,2.2378343807638,-6.17871224587833));
#133694=CARTESIAN_POINT('Ctrl Pts',(20.9029608879772,2.13839881092861,-6.16969916154285));
#133695=CARTESIAN_POINT('Ctrl Pts',(20.8267386383126,2.06326282245282,-6.1635259810367));
#133696=CARTESIAN_POINT('Ctrl Pts',(20.7453009317883,1.96436798655721,-6.15657028512496));
#133697=CARTESIAN_POINT('Ctrl Pts',(20.7320636771059,1.94759519842708,-6.15542705973641));
#133698=CARTESIAN_POINT('Ctrl Pts',(20.7097270652528,1.91805103633547,-6.15348322115078));
#133699=CARTESIAN_POINT('Ctrl Pts',(20.7004668270198,1.90540684845341,-6.15267309604488));
#133700=CARTESIAN_POINT('Ctrl Pts',(20.6782243882741,1.87404493695788,-6.15071697341251));
#133701=CARTESIAN_POINT('Ctrl Pts',(20.6654612999617,1.85517728613556,-6.14958425638012));
#133702=CARTESIAN_POINT('Ctrl Pts',(20.6375599109191,1.81189580118105,-6.14706780939901));
#133703=CARTESIAN_POINT('Ctrl Pts',(20.6226760267317,1.78732775370399,-6.14569614075528));
#133704=CARTESIAN_POINT('Ctrl Pts',(20.5721698227893,1.69845242859358,-6.14088300763944));
#133705=CARTESIAN_POINT('Ctrl Pts',(20.540465224596,1.63203187329078,-6.13755155522816));
#133706=CARTESIAN_POINT('Ctrl Pts',(20.4844006410698,1.48914690638092,-6.13049671404354));
#133707=CARTESIAN_POINT('Ctrl Pts',(20.4610212648567,1.41253730832467,-6.12677259578111));
#133708=CARTESIAN_POINT('Ctrl Pts',(20.436805875047,1.30347994205005,-6.1213120860232));
#133709=CARTESIAN_POINT('Ctrl Pts',(20.4308837375617,1.27229054016978,-6.11973400305116));
#133710=CARTESIAN_POINT('Ctrl Pts',(20.4217173393884,1.21430873009392,-6.11675935037156));
#133711=CARTESIAN_POINT('Ctrl Pts',(20.4182058996628,1.18757088729275,-6.11537175597376));
#133712=CARTESIAN_POINT('Ctrl Pts',(20.4127836711266,1.13580934329507,-6.11265134435453));
#133713=CARTESIAN_POINT('Ctrl Pts',(20.4107792170472,1.11080390447286,-6.11132187629459));
#133714=CARTESIAN_POINT('Ctrl Pts',(20.4077706531801,1.05675830852917,-6.10841482815476));
#133715=CARTESIAN_POINT('Ctrl Pts',(20.4069755445682,1.02771678371464,-6.10683182438699));
#133716=CARTESIAN_POINT('Ctrl Pts',(20.4070005508311,0.998671566178611,
-6.10522917581996));
#133717=CARTESIAN_POINT('',(21.5514861371214,-0.490649428218508,-6.00000000000001));
#133718=CARTESIAN_POINT('Ctrl Pts',(21.5514861371214,-0.490649428218532,
-6.00000000000001));
#133719=CARTESIAN_POINT('Ctrl Pts',(21.4945349590153,-0.475423961817293,
-6.00304030623798));
#133720=CARTESIAN_POINT('Ctrl Pts',(21.4384128966158,-0.456918607184443,
-6.00608061247596));
#133721=CARTESIAN_POINT('Ctrl Pts',(21.38350805469,-0.435247678874912,-6.00912091871394));
#133722=CARTESIAN_POINT('Ctrl Pts',(21.3286309055878,-0.413587680916414,
-6.01215969148671));
#133723=CARTESIAN_POINT('Ctrl Pts',(21.2749702099976,-0.388765455016415,
-6.01519846425949));
#133724=CARTESIAN_POINT('Ctrl Pts',(21.2228965519548,-0.360944380351481,
-6.01823723703227));
#133725=CARTESIAN_POINT('Ctrl Pts',(21.170835959667,-0.333130286247549,
-6.02127524734928));
#133726=CARTESIAN_POINT('Ctrl Pts',(21.1203620422553,-0.302319066725625,
-6.02431325766629));
#133727=CARTESIAN_POINT('Ctrl Pts',(21.0718214599,-0.268720413893039,-6.0273512679833));
#133728=CARTESIAN_POINT('Ctrl Pts',(21.023278430521,-0.235120067288085,
-6.03038943145223));
#133729=CARTESIAN_POINT('Ctrl Pts',(20.976669328728,-0.198732285415966,
-6.03342759492116));
#133730=CARTESIAN_POINT('Ctrl Pts',(20.9323109715251,-0.159809503370445,
-6.03646575839008));
#133731=CARTESIAN_POINT('Ctrl Pts',(20.8879370108942,-0.120873029906427,
-6.03950499055876));
#133732=CARTESIAN_POINT('Ctrl Pts',(20.84581573173,-0.079400106202768,-6.04254422272743));
#133733=CARTESIAN_POINT('Ctrl Pts',(20.8062287260957,-0.035681573206096,
-6.04558345489611));
#133734=CARTESIAN_POINT('Ctrl Pts',(20.7665859145349,0.00809858994418625,
-6.04862697147995));
#133735=CARTESIAN_POINT('Ctrl Pts',(20.7294848338383,0.0541303200353416,
-6.05167048806378));
#133736=CARTESIAN_POINT('Ctrl Pts',(20.6951676387845,0.102088646912787,
-6.05471400464761));
#133737=CARTESIAN_POINT('Ctrl Pts',(20.6608240427085,0.150083869254561,
-6.05775986268005));
#133738=CARTESIAN_POINT('Ctrl Pts',(20.6292688596443,0.200008230956686,
-6.06080572071249));
#133739=CARTESIAN_POINT('Ctrl Pts',(20.6007000136401,0.251509115928909,
-6.06385157874493));
#133740=CARTESIAN_POINT('Ctrl Pts',(20.5720768570487,0.303107906266273,
-6.06690322708258));
#133741=CARTESIAN_POINT('Ctrl Pts',(20.5464515881279,0.356288768094418,
-6.06995487542024));
#133742=CARTESIAN_POINT('Ctrl Pts',(20.5239750856165,0.410676656230577,
-6.07300652375789));
#133743=CARTESIAN_POINT('Ctrl Pts',(20.5137504352638,0.435417922774606,
-6.07439473071918));
#133744=CARTESIAN_POINT('Ctrl Pts',(20.5041767079994,0.460408731288417,
-6.07578293768047));
#133745=CARTESIAN_POINT('Ctrl Pts',(20.4952646815418,0.485612777771825,
-6.07717114464176));
#133746=CARTESIAN_POINT('Ctrl Pts',(20.4737630263397,0.546421474847099,
-6.08052041066706));
#133747=CARTESIAN_POINT('Ctrl Pts',(20.4560483133547,0.60866417772397,-6.08386967669236));
#133748=CARTESIAN_POINT('Ctrl Pts',(20.4422897149553,0.671886056744092,
-6.08721894271766));
#133749=CARTESIAN_POINT('Ctrl Pts',(20.4286352356818,0.734629499910075,
-6.09054286294533));
#133750=CARTESIAN_POINT('Ctrl Pts',(20.4188773539673,0.79833710680527,-6.09386678317299));
#133751=CARTESIAN_POINT('Ctrl Pts',(20.4131347728899,0.862543322046143,
-6.09719070340066));
#133752=CARTESIAN_POINT('Ctrl Pts',(20.4090917965417,0.907746725555561,
-6.09953085858222));
#133753=CARTESIAN_POINT('Ctrl Pts',(20.407038100011,0.953196828097098,-6.10187101376378));
#133754=CARTESIAN_POINT('Ctrl Pts',(20.4070005050181,0.99872588951817,-6.10421116894535));
#133755=CARTESIAN_POINT('',(22.3495840788696,-0.491448861522601,-6.00061432324861));
#133756=CARTESIAN_POINT('Origin',(21.9499999789786,0.999999999999992,-6.00000000000001));
#133757=CARTESIAN_POINT('Ctrl Pts',(22.3492600981242,-0.49044971644798,
-6.00122173936631));
#133758=CARTESIAN_POINT('Ctrl Pts',(22.2389460564105,-0.520000527154304,
-6.00677119856528));
#133759=CARTESIAN_POINT('Ctrl Pts',(22.1256840647128,-0.537215372964368,
-6.01190298829388));
#133760=CARTESIAN_POINT('Ctrl Pts',(21.9677427274376,-0.543520801088802,
-6.01930601480983));
#133761=CARTESIAN_POINT('Ctrl Pts',(21.9238811128887,-0.54340169363555,
-6.0213846758462));
#133762=CARTESIAN_POINT('Ctrl Pts',(21.8428736818116,-0.539727424063985,
-6.02531513175915));
#133763=CARTESIAN_POINT('Ctrl Pts',(21.8057369663867,-0.536692717851297,
-6.02715258783839));
#133764=CARTESIAN_POINT('Ctrl Pts',(21.7405056763577,-0.528976758088233,
-6.03046194549552));
#133765=CARTESIAN_POINT('Ctrl Pts',(21.7123623617402,-0.524856065847814,
-6.03191678715776));
#133766=CARTESIAN_POINT('Ctrl Pts',(21.6503648202652,-0.514020491329616,
-6.03518766512962));
#133767=CARTESIAN_POINT('Ctrl Pts',(21.6165902362738,-0.506942926832763,
-6.03701374319692));
#133768=CARTESIAN_POINT('Ctrl Pts',(21.5117169171735,-0.481268139899593,
-6.04282634549045));
#133769=CARTESIAN_POINT('Ctrl Pts',(21.4416964926351,-0.458723121755922,
-6.0469206074828));
#133770=CARTESIAN_POINT('Ctrl Pts',(21.3106334568717,-0.405937633412248,
-6.05490532750201));
#133771=CARTESIAN_POINT('Ctrl Pts',(21.2494521601919,-0.376474876570989,
-6.05877746229642));
#133772=CARTESIAN_POINT('Ctrl Pts',(21.1661251445168,-0.329348522734971,
-6.06412434161184));
#133773=CARTESIAN_POINT('Ctrl Pts',(21.1422183519377,-0.314958638490253,
-6.06566686852603));
#133774=CARTESIAN_POINT('Ctrl Pts',(21.0997017366622,-0.287769848717985,
-6.06840956690481));
#133775=CARTESIAN_POINT('Ctrl Pts',(21.0809575576242,-0.275195535103139,
-6.06961849079366));
#133776=CARTESIAN_POINT('Ctrl Pts',(21.0490555499635,-0.252764166351627,
-6.07166667355661));
#133777=CARTESIAN_POINT('Ctrl Pts',(21.0357684422469,-0.243100822828799,
-6.0725161757459));
#133778=CARTESIAN_POINT('Ctrl Pts',(21.0063495257877,-0.22097833516864,
-6.07439024599287));
#133779=CARTESIAN_POINT('Ctrl Pts',(20.990305966843,-0.208408766142356,
-6.07540837189322));
#133780=CARTESIAN_POINT('Ctrl Pts',(20.9168587552396,-0.148479743675298,
-6.08007417882351));
#133781=CARTESIAN_POINT('Ctrl Pts',(20.8626762669674,-0.0973218886797023,
-6.08353352830336));
#133782=CARTESIAN_POINT('Ctrl Pts',(20.7497573544803,0.0259043337482767,
-6.09128365314722));
#133783=CARTESIAN_POINT('Ctrl Pts',(20.6934103137738,0.0997633753528193,
-6.09556198197975));
#133784=CARTESIAN_POINT('Ctrl Pts',(20.6246422260201,0.209049987884131,
-6.10183457832132));
#133785=CARTESIAN_POINT('Ctrl Pts',(20.6063461910823,0.240546676970981,
-6.10363440488854));
#133786=CARTESIAN_POINT('Ctrl Pts',(20.576012610059,0.297299312273243,-6.10688156409804));
#133787=CARTESIAN_POINT('Ctrl Pts',(20.5635152670006,0.322290943916612,
-6.10831273841653));
#133788=CARTESIAN_POINT('Ctrl Pts',(20.5371537861922,0.378792418623317,
-6.11155694980618));
#133789=CARTESIAN_POINT('Ctrl Pts',(20.523652016707,0.410454007411718,-6.11338078139074));
#133790=CARTESIAN_POINT('Ctrl Pts',(20.4855010749848,0.508919708531068,
-6.11907447167697));
#133791=CARTESIAN_POINT('Ctrl Pts',(20.4644086054296,0.576994687016685,
-6.12304523881323));
#133792=CARTESIAN_POINT('Ctrl Pts',(20.426371671626,0.738499367635295,-6.13244484822318));
#133793=CARTESIAN_POINT('Ctrl Pts',(20.4131917664023,0.832527525450142,
-6.13790678576824));
#133794=CARTESIAN_POINT('Ctrl Pts',(20.4074799514418,0.953407776264625,
-6.14455885747248));
#133795=CARTESIAN_POINT('Ctrl Pts',(20.4069102795322,0.979672727419416,
-6.14598107986032));
#133796=CARTESIAN_POINT('Ctrl Pts',(20.407074337124,1.0222834328177,-6.14823787442868));
#133797=CARTESIAN_POINT('Ctrl Pts',(20.4073968871114,1.0386246937928,-6.14909100723485));
#133798=CARTESIAN_POINT('Ctrl Pts',(20.4087087238537,1.07543140343511,-6.1509823018051));
#133799=CARTESIAN_POINT('Ctrl Pts',(20.4098460050509,1.09588765886885,-6.15201339257036));
#133800=CARTESIAN_POINT('Ctrl Pts',(20.4160801089225,1.1783513212385,-6.15610974492835));
#133801=CARTESIAN_POINT('Ctrl Pts',(20.4245177640344,1.24005114339434,-6.15903835603049));
#133802=CARTESIAN_POINT('Ctrl Pts',(20.4591147545198,1.41395044292493,-6.16728631434038));
#133803=CARTESIAN_POINT('Ctrl Pts',(20.4941261403144,1.52395053529094,-6.17252368462059));
#133804=CARTESIAN_POINT('Ctrl Pts',(20.5549909095745,1.66027988345722,-6.17980850959296));
#133805=CARTESIAN_POINT('Ctrl Pts',(20.569975055633,1.69105052649164,-6.18150656486357));
#133806=CARTESIAN_POINT('Ctrl Pts',(20.5990244616489,1.74598534889885,-6.18465173205501));
#133807=CARTESIAN_POINT('Ctrl Pts',(20.6127472285442,1.77031418507078,-6.18608696454662));
#133808=CARTESIAN_POINT('Ctrl Pts',(20.6456358647184,1.82509203036845,-6.18942227251122));
#133809=CARTESIAN_POINT('Ctrl Pts',(20.6652210329991,1.8552691916005,-6.19133632453058));
#133810=CARTESIAN_POINT('Ctrl Pts',(20.7399076036783,1.96198572939441,-6.19839177344126));
#133811=CARTESIAN_POINT('Ctrl Pts',(20.8009359090357,2.03411237170792,-6.20373317207936));
#133812=CARTESIAN_POINT('Ctrl Pts',(20.9211764269764,2.15234553094063,-6.2133402501196));
#133813=CARTESIAN_POINT('Ctrl Pts',(20.9778985205184,2.20058240741101,-6.21757715180105));
#133814=CARTESIAN_POINT('Ctrl Pts',(21.0559785456939,2.25780688078353,-6.22285164873405));
#133815=CARTESIAN_POINT('Ctrl Pts',(21.0743646949676,2.27067518339825,-6.22405636420658));
#133816=CARTESIAN_POINT('Ctrl Pts',(21.1064163536908,2.29208163553281,-6.22608456222704));
#133817=CARTESIAN_POINT('Ctrl Pts',(21.1199452962614,2.30081418536878,-6.22691880436355));
#133818=CARTESIAN_POINT('Ctrl Pts',(21.1533951002631,2.32167064583337,-6.22892986322777));
#133819=CARTESIAN_POINT('Ctrl Pts',(21.1734581438383,2.33355746512882,-6.23009342356617));
#133820=CARTESIAN_POINT('Ctrl Pts',(21.2193653160923,2.35936870536518,-6.23267777615744));
#133821=CARTESIAN_POINT('Ctrl Pts',(21.2453530360858,2.37301970664579,-6.23408677404265));
#133822=CARTESIAN_POINT('Ctrl Pts',(21.3401133532828,2.41939640591508,-6.23908539283991));
#133823=CARTESIAN_POINT('Ctrl Pts',(21.4108974256887,2.44776275967269,-6.24256715351212));
#133824=CARTESIAN_POINT('Ctrl Pts',(21.4885359458098,2.47238853170355,-6.24635610638211));
#133825=CARTESIAN_POINT('Ctrl Pts',(21.4935918018411,2.47396357410221,-6.24660268601106));
#133826=CARTESIAN_POINT('Ctrl Pts',(21.5622279170449,2.49495866560251,-6.24994881050477));
#133827=CARTESIAN_POINT('Ctrl Pts',(21.6269866199216,2.51027481141422,-6.25309455412155));
#133828=CARTESIAN_POINT('Ctrl Pts',(21.7244173001186,2.52676374822183,-6.25794806330741));
#133829=CARTESIAN_POINT('Ctrl Pts',(21.7564673785425,2.53115643878961,-6.2595628771343));
#133830=CARTESIAN_POINT('Ctrl Pts',(21.8168444990354,2.53750559320117,-6.26265054819264));
#133831=CARTESIAN_POINT('Ctrl Pts',(21.8451336436462,2.53969371943589,-6.26411584255606));
#133832=CARTESIAN_POINT('Ctrl Pts',(21.9131739847374,2.5430727347742,-6.26768994805713));
#133833=CARTESIAN_POINT('Ctrl Pts',(21.9529408887972,2.54350918749679,-6.26981984984527));
#133834=CARTESIAN_POINT('Ctrl Pts',(22.0415697650441,2.54105684256572,-6.27465787470543));
#133835=CARTESIAN_POINT('Ctrl Pts',(22.0903664911747,2.53738022209195,-6.27738386990655));
#133836=CARTESIAN_POINT('Ctrl Pts',(22.2265459946849,2.52058191394221,-6.28512499152032));
#133837=CARTESIAN_POINT('Ctrl Pts',(22.3130971043322,2.50226743725145,-6.29020900478887));
#133838=CARTESIAN_POINT('Ctrl Pts',(22.4309242280149,2.46655138514755,-6.29706996368971));
#133839=CARTESIAN_POINT('Ctrl Pts',(22.4638931476742,2.4553264943439,-6.29898122936458));
#133840=CARTESIAN_POINT('Ctrl Pts',(22.5128797035298,2.43677550142827,-6.3017808672692));
#133841=CARTESIAN_POINT('Ctrl Pts',(22.5291970295223,2.43027559174652,-6.30270649612236));
#133842=CARTESIAN_POINT('Ctrl Pts',(22.5620524528981,2.4165332895137,-6.30455107145079));
#133843=CARTESIAN_POINT('Ctrl Pts',(22.5785814608003,2.40927646966181,-6.30546913265023));
#133844=CARTESIAN_POINT('Ctrl Pts',(22.6297832884031,2.38571691547216,-6.30829280364629));
#133845=CARTESIAN_POINT('Ctrl Pts',(22.6639803134744,2.36841118237412,-6.31014945798633));
#133846=CARTESIAN_POINT('Ctrl Pts',(22.7645337602741,2.31272818320848,-6.31561738288569));
#133847=CARTESIAN_POINT('Ctrl Pts',(22.8287116292269,2.27066407013551,-6.31912334298961));
#133848=CARTESIAN_POINT('Ctrl Pts',(22.8895003442092,2.22400492798496,-6.32268395960923));
#133849=CARTESIAN_POINT('Origin',(-21.9500000210213,0.999999999999992,-4.89578827641128));
#133850=CARTESIAN_POINT('',(-21.0105083902185,2.22401163215526,-7.78024815277603));
#133851=CARTESIAN_POINT('',(-21.0105083757967,2.22401162108585,-7.82252260735286));
#133852=CARTESIAN_POINT('',(-21.0105083758276,2.22401162110953,-4.89578827641128));
#133853=CARTESIAN_POINT('',(-21.5514861791641,-0.490649428218508,-8.00000000000001));
#133854=CARTESIAN_POINT('Ctrl Pts',(-21.0105083757967,2.22401162108585,
-7.82252260735286));
#133855=CARTESIAN_POINT('Ctrl Pts',(-21.0101364665912,2.22372616171165,
-7.82254903034026));
#133856=CARTESIAN_POINT('Ctrl Pts',(-21.0097646849254,2.22344053087246,
-7.82257545653808));
#133857=CARTESIAN_POINT('Ctrl Pts',(-20.9415574485498,2.17098911014149,
-7.8274258697074));
#133858=CARTESIAN_POINT('Ctrl Pts',(-20.8781806357393,2.11327211895452,
-7.83235245582535));
#133859=CARTESIAN_POINT('Ctrl Pts',(-20.7931319397805,2.021788962789,-7.83935306760022));
#133860=CARTESIAN_POINT('Ctrl Pts',(-20.7674574930824,1.99196270521193,
-7.84152583818574));
#133861=CARTESIAN_POINT('Ctrl Pts',(-20.7316291236481,1.94696970088399,
-7.84461094125883));
#133862=CARTESIAN_POINT('Ctrl Pts',(-20.7205600831609,1.93255388876716,
-7.84557212336584));
#133863=CARTESIAN_POINT('Ctrl Pts',(-20.6999790583234,1.90474650013823,
-7.84736967305452));
#133864=CARTESIAN_POINT('Ctrl Pts',(-20.6904217720473,1.89139288667088,
-7.84820831404718));
#133865=CARTESIAN_POINT('Ctrl Pts',(-20.6638711720371,1.85301603447934,
-7.85055540520169));
#133866=CARTESIAN_POINT('Ctrl Pts',(-20.6473972055945,1.82764115965349,
-7.85203352878403));
#133867=CARTESIAN_POINT('Ctrl Pts',(-20.6088757422345,1.76430386038195,
-7.85558658163264));
#133868=CARTESIAN_POINT('Ctrl Pts',(-20.5876813430491,1.72585321197464,
-7.8576288300798));
#133869=CARTESIAN_POINT('Ctrl Pts',(-20.5153433346791,1.58025565853965,
-7.86512319148981));
#133870=CARTESIAN_POINT('Ctrl Pts',(-20.4749760545482,1.46823052444739,
-7.87046330075095));
#133871=CARTESIAN_POINT('Ctrl Pts',(-20.4400936045535,1.3196598991621,-7.87787308008542));
#133872=CARTESIAN_POINT('Ctrl Pts',(-20.4334312005787,1.28638896378547,
-7.87954958683943));
#133873=CARTESIAN_POINT('Ctrl Pts',(-20.4234590698477,1.2263760915183,-7.88261793112134));
#133874=CARTESIAN_POINT('Ctrl Pts',(-20.4197428587125,1.19971557253502,
-7.88399643310594));
#133875=CARTESIAN_POINT('Ctrl Pts',(-20.4129891727275,1.13984911668774,
-7.88713097929326));
#133876=CARTESIAN_POINT('Ctrl Pts',(-20.4103269711696,1.10661518845308,
-7.88889789704431));
#133877=CARTESIAN_POINT('Ctrl Pts',(-20.4050970260198,0.996680750127306,
-7.89483355749922));
#133878=CARTESIAN_POINT('Ctrl Pts',(-20.4071730285304,0.919881221640968,
-7.89913247009676));
#133879=CARTESIAN_POINT('Ctrl Pts',(-20.4249337908562,0.745603808065916,
-7.90909211026956));
#133880=CARTESIAN_POINT('Ctrl Pts',(-20.4442706781516,0.648823289085554,
-7.91477605849206));
#133881=CARTESIAN_POINT('Ctrl Pts',(-20.478551910376,0.535133969891604,
-7.9212194892826));
#133882=CARTESIAN_POINT('Ctrl Pts',(-20.4847866649622,0.515841072379941,
-7.92230381076316));
#133883=CARTESIAN_POINT('Ctrl Pts',(-20.4966653771655,0.4814173590333,-7.9242148922779));
#133884=CARTESIAN_POINT('Ctrl Pts',(-20.5021692818573,0.466243780132118,
-7.92504824956178));
#133885=CARTESIAN_POINT('Ctrl Pts',(-20.5168580125421,0.427648969840413,
-7.92714911191537));
#133886=CARTESIAN_POINT('Ctrl Pts',(-20.5263791873653,0.404361209544981,
-7.92839926840572));
#133887=CARTESIAN_POINT('Ctrl Pts',(-20.549463745622,0.351618962859086,
-7.93121062067599));
#133888=CARTESIAN_POINT('Ctrl Pts',(-20.563394706907,0.322338055432545,
-7.93275679063243));
#133889=CARTESIAN_POINT('Ctrl Pts',(-20.6203510831758,0.211747237138487,
-7.93861007554522));
#133890=CARTESIAN_POINT('Ctrl Pts',(-20.6696914423677,0.133905544782897,
-7.94276892681729));
#133891=CARTESIAN_POINT('Ctrl Pts',(-20.7662759191897,0.00798323245494448,
-7.95016071945355));
#133892=CARTESIAN_POINT('Ctrl Pts',(-20.8102671522517,-0.0422610010400515,
-7.95332402361043));
#133893=CARTESIAN_POINT('Ctrl Pts',(-20.8817143842222,-0.113913629167302,
-7.9582974566318));
#133894=CARTESIAN_POINT('Ctrl Pts',(-20.9068697361912,-0.137504627672249,
-7.96002072079728));
#133895=CARTESIAN_POINT('Ctrl Pts',(-20.9565760612962,-0.18108350126588,
-7.96338515672788));
#133896=CARTESIAN_POINT('Ctrl Pts',(-20.9809934423874,-0.201197521638292,
-7.96502050629124));
#133897=CARTESIAN_POINT('Ctrl Pts',(-21.0454698315142,-0.251064557923271,
-7.96929935346712));
#133898=CARTESIAN_POINT('Ctrl Pts',(-21.0863831581526,-0.279649458108628,
-7.97197811452552));
#133899=CARTESIAN_POINT('Ctrl Pts',(-21.2322368052158,-0.371368263218477,
-7.98138249353394));
#133900=CARTESIAN_POINT('Ctrl Pts',(-21.3432485853337,-0.423968475974452,
-7.98832698880254));
#133901=CARTESIAN_POINT('Ctrl Pts',(-21.4765752288491,-0.468689818554702,
-7.99589803576898));
#133902=CARTESIAN_POINT('Ctrl Pts',(-21.4939471892734,-0.47417660831274,
-7.99686953981591));
#133903=CARTESIAN_POINT('Ctrl Pts',(-21.5247187777658,-0.483299523563084,
-7.99856015766123));
#133904=CARTESIAN_POINT('Ctrl Pts',(-21.5380778050746,-0.487064800894149,
-7.99928420157857));
#133905=CARTESIAN_POINT('Ctrl Pts',(-21.5514861791641,-0.490649428218531,
-7.99999999999997));
#133906=CARTESIAN_POINT('',(-22.3495836570369,-0.491450109733673,-7.99938619261749));
#133907=CARTESIAN_POINT('Origin',(-21.9500000210213,0.999999999999992,-8.00000000000001));
#133908=CARTESIAN_POINT('Ctrl Pts',(-22.3492583994676,-0.490450182743604,
-7.99877810051043));
#133909=CARTESIAN_POINT('Ctrl Pts',(-22.2384388820329,-0.520136261046303,
-7.99320323557973));
#133910=CARTESIAN_POINT('Ctrl Pts',(-22.1246459944166,-0.537372637890604,
-7.98804968162678));
#133911=CARTESIAN_POINT('Ctrl Pts',(-21.9664146949985,-0.543528710254337,
-7.98063115457279));
#133912=CARTESIAN_POINT('Ctrl Pts',(-21.9227930458819,-0.543376110631364,
-7.97856310091227));
#133913=CARTESIAN_POINT('Ctrl Pts',(-21.8421707043095,-0.539674874830167,
-7.9746501645128));
#133914=CARTESIAN_POINT('Ctrl Pts',(-21.8051788113476,-0.536636731148366,
-7.97281937567373));
#133915=CARTESIAN_POINT('Ctrl Pts',(-21.7401379958302,-0.528925477980793,
-7.96951906637576));
#133916=CARTESIAN_POINT('Ctrl Pts',(-21.7120409465171,-0.524805081106625,
-7.96806637484147));
#133917=CARTESIAN_POINT('Ctrl Pts',(-21.650086568324,-0.513965478821969,
-7.96479733085237));
#133918=CARTESIAN_POINT('Ctrl Pts',(-21.6163094102781,-0.506880848368754,
-7.96297085456803));
#133919=CARTESIAN_POINT('Ctrl Pts',(-21.5110114463801,-0.481081012433662,
-7.95713388664677));
#133920=CARTESIAN_POINT('Ctrl Pts',(-21.4405862735911,-0.458357903949134,
-7.95301400344654));
#133921=CARTESIAN_POINT('Ctrl Pts',(-21.3095237292062,-0.405414164595004,
-7.94502466825928));
#133922=CARTESIAN_POINT('Ctrl Pts',(-21.2487049862821,-0.376075685144217,
-7.94117463103428));
#133923=CARTESIAN_POINT('Ctrl Pts',(-21.1657927426782,-0.329150740126245,
-7.9358540260567));
#133924=CARTESIAN_POINT('Ctrl Pts',(-21.1419585008929,-0.314797236550457,
-7.93431615194845));
#133925=CARTESIAN_POINT('Ctrl Pts',(-21.0995576879271,-0.287673787591833,
-7.93158091869557));
#133926=CARTESIAN_POINT('Ctrl Pts',(-21.0808578105156,-0.275126605941027,
-7.9303748663119));
#133927=CARTESIAN_POINT('Ctrl Pts',(-21.04901952846,-0.252737905173928,
-7.92833078870972));
#133928=CARTESIAN_POINT('Ctrl Pts',(-21.0357526680659,-0.243088863336784,
-7.92748258443072));
#133929=CARTESIAN_POINT('Ctrl Pts',(-21.0063770126725,-0.220999055005691,
-7.92561126463514));
#133930=CARTESIAN_POINT('Ctrl Pts',(-20.9903562287209,-0.208448152004266,
-7.92459457615832));
#133931=CARTESIAN_POINT('Ctrl Pts',(-20.9160165047158,-0.147798369704182,
-7.91987207901798));
#133932=CARTESIAN_POINT('Ctrl Pts',(-20.861031231293,-0.0957699230770892,
-7.91636116260214));
#133933=CARTESIAN_POINT('Ctrl Pts',(-20.7482389106577,0.027869189716978,
-7.90860196020264));
#133934=CARTESIAN_POINT('Ctrl Pts',(-20.692570999941,0.101034389439105,
-7.90436462058109));
#133935=CARTESIAN_POINT('Ctrl Pts',(-20.6244066672067,0.209449570851663,
-7.89814236080197));
#133936=CARTESIAN_POINT('Ctrl Pts',(-20.6061700119408,0.240863394503106,
-7.89634727513816));
#133937=CARTESIAN_POINT('Ctrl Pts',(-20.5759137041703,0.29749449652976,
-7.89310706347015));
#133938=CARTESIAN_POINT('Ctrl Pts',(-20.5634384547691,0.322449937740252,
-7.89167795074537));
#133939=CARTESIAN_POINT('Ctrl Pts',(-20.5371092778647,0.378895001071782,
-7.88843696223817));
#133940=CARTESIAN_POINT('Ctrl Pts',(-20.5236184236341,0.41053670672039,
-7.88661426736097));
#133941=CARTESIAN_POINT('Ctrl Pts',(-20.4854206959021,0.509135814754278,
-7.88091285356935));
#133942=CARTESIAN_POINT('Ctrl Pts',(-20.4642933731975,0.577372119177006,
-7.87693256769951));
#133943=CARTESIAN_POINT('Ctrl Pts',(-20.4263143282665,0.738892566900184,
-7.86753224324677));
#133944=CARTESIAN_POINT('Ctrl Pts',(-20.4131762028146,0.832762284156119,
-7.8620800221764));
#133945=CARTESIAN_POINT('Ctrl Pts',(-20.4074791168623,0.953452867454163,
-7.85543859438069));
#133946=CARTESIAN_POINT('Ctrl Pts',(-20.4069105875293,0.979689338170266,
-7.85401794089713));
#133947=CARTESIAN_POINT('Ctrl Pts',(-20.407074122763,1.02224945059713,-7.85176381209117));
#133948=CARTESIAN_POINT('Ctrl Pts',(-20.4073957602307,1.0385686178664,-7.85091180793199));
#133949=CARTESIAN_POINT('Ctrl Pts',(-20.4087032216148,1.07530486524538,
-7.84902404313319));
#133950=CARTESIAN_POINT('Ctrl Pts',(-20.4098358161491,1.09571282519011,
-7.84799529516952));
#133951=CARTESIAN_POINT('Ctrl Pts',(-20.4155956852066,1.17205054070338,
-7.84420284070168));
#133952=CARTESIAN_POINT('Ctrl Pts',(-20.4228676212515,1.22774018619161,
-7.8415474830042));
#133953=CARTESIAN_POINT('Ctrl Pts',(-20.4484032470428,1.36464968149549,
-7.83504944595518));
#133954=CARTESIAN_POINT('Ctrl Pts',(-20.4702296781954,1.445019155653,-7.83125563776568));
#133955=CARTESIAN_POINT('Ctrl Pts',(-20.5164716674808,1.57330416441257,
-7.82481900236634));
#133956=CARTESIAN_POINT('Ctrl Pts',(-20.5370951030455,1.6223988119019,-7.82225979576069));
#133957=CARTESIAN_POINT('Ctrl Pts',(-20.5731772706048,1.69720781856102,
-7.81814274628359));
#133958=CARTESIAN_POINT('Ctrl Pts',(-20.5869186867565,1.72370488261534,
-7.81664000558087));
#133959=CARTESIAN_POINT('Ctrl Pts',(-20.6155331988979,1.77517155548965,
-7.81362360810701));
#133960=CARTESIAN_POINT('Ctrl Pts',(-20.6303604959109,1.80015249733067,
-7.81211193555699));
#133961=CARTESIAN_POINT('Ctrl Pts',(-20.6709788817185,1.86438333425773,
-7.80809366056266));
#133962=CARTESIAN_POINT('Ctrl Pts',(-20.6978708531977,1.90289844092202,
-7.80554979851484));
#133963=CARTESIAN_POINT('Ctrl Pts',(-20.7660407117086,1.99161801298054,
-7.7993678259325));
#133964=CARTESIAN_POINT('Ctrl Pts',(-20.8088152773384,2.04055869075717,
-7.79568820833976));
#133965=CARTESIAN_POINT('Ctrl Pts',(-20.9033924699419,2.13590186039225,
-7.78803967956329));
#133966=CARTESIAN_POINT('Ctrl Pts',(-20.9555001348351,2.18178997821006,
-7.78407748728989));
#133967=CARTESIAN_POINT('Ctrl Pts',(-21.0105083902185,2.22401163215526,
-7.78024815277603));
#133968=CARTESIAN_POINT('Origin',(-21.9500000210213,0.999999999999992,-4.89578827641128));
#133969=CARTESIAN_POINT('',(-21.0105083871506,2.22401162980051,-7.28231522554091));
#133970=CARTESIAN_POINT('',(-21.0105083124886,2.22401157249358,-7.32301699234766));
#133971=CARTESIAN_POINT('',(-21.0105083758276,2.22401162110953,-4.89578827641128));
#133972=CARTESIAN_POINT('',(-23.4929999234274,0.999451206005362,-7.64468148481327));
#133973=CARTESIAN_POINT('Ctrl Pts',(-21.0105083124886,2.22401157249359,
-7.32301699234766));
#133974=CARTESIAN_POINT('Ctrl Pts',(-20.9825174099087,2.20252711803328,
-7.32465074210701));
#133975=CARTESIAN_POINT('Ctrl Pts',(-20.9552590027711,2.18007909040033,
-7.32628511078963));
#133976=CARTESIAN_POINT('Ctrl Pts',(-20.8802334173451,2.11384142226394,
-7.33096327137465));
#133977=CARTESIAN_POINT('Ctrl Pts',(-20.8344335815339,2.06796717042893,
-7.33404150784907));
#133978=CARTESIAN_POINT('Ctrl Pts',(-20.7710173471336,1.99590392117325,
-7.33877508236544));
#133979=CARTESIAN_POINT('Ctrl Pts',(-20.7510988824047,1.9718336587144,-7.34034038852786));
#133980=CARTESIAN_POINT('Ctrl Pts',(-20.7143546234119,1.92458032026418,
-7.34339399104344));
#133981=CARTESIAN_POINT('Ctrl Pts',(-20.6974168159423,1.90150069016189,
-7.34487715139806));
#133982=CARTESIAN_POINT('Ctrl Pts',(-20.6569904945918,1.84307497164331,
-7.34861678929152));
#133983=CARTESIAN_POINT('Ctrl Pts',(-20.6343005404688,1.80720721579581,
-7.35090000409829));
#133984=CARTESIAN_POINT('Ctrl Pts',(-20.556610532312,1.67240022770003,-7.35943299964571));
#133985=CARTESIAN_POINT('Ctrl Pts',(-20.5110646580972,1.56843379141645,
-7.36595299644807));
#133986=CARTESIAN_POINT('Ctrl Pts',(-20.4671347665531,1.42792534268164,
-7.37426528765962));
#133987=CARTESIAN_POINT('Ctrl Pts',(-20.4580485041753,1.39508268472228,
-7.37617180250815));
#133988=CARTESIAN_POINT('Ctrl Pts',(-20.444003816196,1.33688302021406,-7.37945930259372));
#133989=CARTESIAN_POINT('Ctrl Pts',(-20.4385808188261,1.31165184878328,
-7.38085500811797));
#133990=CARTESIAN_POINT('Ctrl Pts',(-20.4307943588022,1.27041510178611,
-7.38307589604204));
#133991=CARTESIAN_POINT('Ctrl Pts',(-20.4280453875969,1.25448838415569,
-7.38391888361165));
#133992=CARTESIAN_POINT('Ctrl Pts',(-20.4223453296819,1.21805754009262,
-7.38581152273993));
#133993=CARTESIAN_POINT('Ctrl Pts',(-20.4195559395557,1.19753212131848,
-7.38685338534983));
#133994=CARTESIAN_POINT('Ctrl Pts',(-20.4104299899328,1.11848170660292,
-7.39079260141721));
#133995=CARTESIAN_POINT('Ctrl Pts',(-20.4070305032439,1.05966466419257,
-7.39357083336393));
#133996=CARTESIAN_POINT('Ctrl Pts',(-20.4069385286596,0.880834598077489,
-7.40190359308587));
#133997=CARTESIAN_POINT('Ctrl Pts',(-20.4208651202421,0.761285046035383,
-7.40735178265562));
#133998=CARTESIAN_POINT('Ctrl Pts',(-20.456251147579,0.611804087759982,
-7.41486317912615));
#133999=CARTESIAN_POINT('Ctrl Pts',(-20.4650733571445,0.579316786439152,
-7.41653669605546));
#134000=CARTESIAN_POINT('Ctrl Pts',(-20.4831985698121,0.52027889734565,
-7.41966729640507));
#134001=CARTESIAN_POINT('Ctrl Pts',(-20.4921788946539,0.49364412905756,
-7.42111389940446));
#134002=CARTESIAN_POINT('Ctrl Pts',(-20.5147072589758,0.432405270198859,
-7.42452558022747));
#134003=CARTESIAN_POINT('Ctrl Pts',(-20.5287875219883,0.398016755426616,
-7.42650669084278));
#134004=CARTESIAN_POINT('Ctrl Pts',(-20.5622016925475,0.324133344117312,
-7.4309089545039));
#134005=CARTESIAN_POINT('Ctrl Pts',(-20.5820101956731,0.284889258787158,
-7.43334252240344));
#134006=CARTESIAN_POINT('Ctrl Pts',(-20.6637999857438,0.138718718927442,
-7.44274379721125));
#134007=CARTESIAN_POINT('Ctrl Pts',(-20.7368651968496,0.0385327322597062,
-7.44994243427988));
#134008=CARTESIAN_POINT('Ctrl Pts',(-20.8356420516684,-0.0674786742026878,
-7.45781325123887));
#134009=CARTESIAN_POINT('Ctrl Pts',(-20.8505127447654,-0.0827890930495645,
-7.45895589166271));
#134010=CARTESIAN_POINT('Ctrl Pts',(-20.8772111809303,-0.109159602219511,
-7.46092680846376));
#134011=CARTESIAN_POINT('Ctrl Pts',(-20.88890283473,-0.120349814725715,
-7.46176344954001));
#134012=CARTESIAN_POINT('Ctrl Pts',(-20.9186285316735,-0.147917722788811,
-7.463827551843));
#134013=CARTESIAN_POINT('Ctrl Pts',(-20.9368778425727,-0.164055761895932,
-7.46503962438934));
#134014=CARTESIAN_POINT('Ctrl Pts',(-20.9794194152348,-0.199916990876399,
-7.46776144170377));
#134015=CARTESIAN_POINT('Ctrl Pts',(-21.0039449655319,-0.219347157900796,
-7.46925730064342));
#134016=CARTESIAN_POINT('Ctrl Pts',(-21.1004826953953,-0.291160989232186,
-7.4749373138021));
#134017=CARTESIAN_POINT('Ctrl Pts',(-21.1763866890077,-0.338020772946308,
-7.47898466000172));
#134018=CARTESIAN_POINT('Ctrl Pts',(-21.3098275538653,-0.40523052196344,
-7.48599160329124));
#134019=CARTESIAN_POINT('Ctrl Pts',(-21.3652891660476,-0.429197680117652,
-7.4888733748211));
#134020=CARTESIAN_POINT('Ctrl Pts',(-21.4509546007336,-0.460394340771098,
-7.49337696367223));
#134021=CARTESIAN_POINT('Ctrl Pts',(-21.4802080171293,-0.47006573856716,
-7.49492315699789));
#134022=CARTESIAN_POINT('Ctrl Pts',(-21.5373387453146,-0.487074128834837,
-7.49796824884198));
#134023=CARTESIAN_POINT('Ctrl Pts',(-21.56517082176,-0.494518364049688,
-7.49946308194927));
#134024=CARTESIAN_POINT('Ctrl Pts',(-21.6359399645652,-0.511339055157261,
-7.50329762925914));
#134025=CARTESIAN_POINT('Ctrl Pts',(-21.679097562047,-0.519668003638882,
-7.50566733676152));
#134026=CARTESIAN_POINT('Ctrl Pts',(-21.8309885556989,-0.542305271731283,
-7.51410992656871));
#134027=CARTESIAN_POINT('Ctrl Pts',(-21.9408365684424,-0.546861831239269,
-7.52042331398859));
#134028=CARTESIAN_POINT('Ctrl Pts',(-22.0958932938982,-0.53676888202514,
-7.52919847845896));
#134029=CARTESIAN_POINT('Ctrl Pts',(-22.1414098711509,-0.531765722993547,
-7.53175292081958));
#134030=CARTESIAN_POINT('Ctrl Pts',(-22.2069442455781,-0.521594851987155,
-7.53534307517313));
#134031=CARTESIAN_POINT('Ctrl Pts',(-22.2271853538923,-0.518038075534597,
-7.53643955310714));
#134032=CARTESIAN_POINT('Ctrl Pts',(-22.2634430446844,-0.51091741548571,
-7.53837419482939));
#134033=CARTESIAN_POINT('Ctrl Pts',(-22.279482987493,-0.507500896406463,
-7.53921887770395));
#134034=CARTESIAN_POINT('Ctrl Pts',(-22.3212785846377,-0.497899401140471,
-7.54139486311327));
#134035=CARTESIAN_POINT('Ctrl Pts',(-22.3469344129687,-0.491306011968331,
-7.54270631114527));
#134036=CARTESIAN_POINT('Ctrl Pts',(-22.4064675711735,-0.474360991844471,
-7.54571807414151));
#134037=CARTESIAN_POINT('Ctrl Pts',(-22.4401837662657,-0.463496861682668,
-7.54739969250235));
#134038=CARTESIAN_POINT('Ctrl Pts',(-22.5934123338542,-0.408232804815731,
-7.5550447355139));
#134039=CARTESIAN_POINT('Ctrl Pts',(-22.7075008109141,-0.350293314109797,
-7.56079061806701));
#134040=CARTESIAN_POINT('Ctrl Pts',(-22.8421048301696,-0.259451035805984,
-7.56870602408927));
#134041=CARTESIAN_POINT('Ctrl Pts',(-22.8703711059668,-0.238945014554024,
-7.57043691824677));
#134042=CARTESIAN_POINT('Ctrl Pts',(-22.920102126338,-0.200225593617103,
-7.5736245937489));
#134043=CARTESIAN_POINT('Ctrl Pts',(-22.9418105371418,-0.18234992364591,
-7.57506848978076));
#134044=CARTESIAN_POINT('Ctrl Pts',(-22.9900174503622,-0.140392028154088,
-7.57840233260295));
#134045=CARTESIAN_POINT('Ctrl Pts',(-23.0161897903214,-0.11596117382787,
-7.58030550933155));
#134046=CARTESIAN_POINT('Ctrl Pts',(-23.0707648472802,-0.061343877884279,
-7.58448345814335));
#134047=CARTESIAN_POINT('Ctrl Pts',(-23.0988486391809,-0.0308788126267512,
-7.58676806107228));
#134048=CARTESIAN_POINT('Ctrl Pts',(-23.1914998655966,0.0781224522796942,
-7.59476820294255));
#134049=CARTESIAN_POINT('Ctrl Pts',(-23.2495112925459,0.161877582365277,
-7.60064078391186));
#134050=CARTESIAN_POINT('Ctrl Pts',(-23.3171212636818,0.283590941131213,
-7.60842788628872));
#134051=CARTESIAN_POINT('Ctrl Pts',(-23.3341714951037,0.317114857107446,
-7.61049976047697));
#134052=CARTESIAN_POINT('Ctrl Pts',(-23.3575265775445,0.367512801829775,
-7.6134753723346));
#134053=CARTESIAN_POINT('Ctrl Pts',(-23.3647878991279,0.383926644308552,
-7.61442335329552));
#134054=CARTESIAN_POINT('Ctrl Pts',(-23.3785471106268,0.416555746178902,
-7.6162611971365));
#134055=CARTESIAN_POINT('Ctrl Pts',(-23.3850592199905,0.432761853411496,
-7.61715156911495));
#134056=CARTESIAN_POINT('Ctrl Pts',(-23.4036813872892,0.481480027026735,
-7.61977108682102));
#134057=CARTESIAN_POINT('Ctrl Pts',(-23.4149722010192,0.514295073396851,
-7.62146071096474));
#134058=CARTESIAN_POINT('Ctrl Pts',(-23.4567647225752,0.650527847038154,
-7.62827219534873));
#134059=CARTESIAN_POINT('Ctrl Pts',(-23.4774950477446,0.756623954743234,
-7.63312464040482));
#134060=CARTESIAN_POINT('Ctrl Pts',(-23.4909810007103,0.909055911904548,
-7.64031701852787));
#134061=CARTESIAN_POINT('Ctrl Pts',(-23.4929838445311,0.954243467532069,
-7.64247299936936));
#134062=CARTESIAN_POINT('Ctrl Pts',(-23.4929999234274,0.999451206005372,
-7.64468148481327));
#134063=CARTESIAN_POINT('Ctrl Pts',(-23.4929999238988,0.999452532970484,
-7.6446815496381));
#134064=CARTESIAN_POINT('Ctrl Pts',(-23.4930085114816,1.02365607183503,
-7.64586393984481));
#134065=CARTESIAN_POINT('Ctrl Pts',(-23.4924476138905,1.0478558850477,-7.64706073081155));
#134066=CARTESIAN_POINT('Ctrl Pts',(-23.4901694298798,1.09660371989079,
-7.64950686770363));
#134067=CARTESIAN_POINT('Ctrl Pts',(-23.4884337229621,1.12114349549346,
-7.65075638292366));
#134068=CARTESIAN_POINT('Ctrl Pts',(-23.4832437590197,1.17588730286728,
-7.6535890139563));
#134069=CARTESIAN_POINT('Ctrl Pts',(-23.4794820947881,1.20605126467252,
-7.65518079881767));
#134070=CARTESIAN_POINT('Ctrl Pts',(-23.4665063553662,1.28985996614385,
-7.65969496515285));
#134071=CARTESIAN_POINT('Ctrl Pts',(-23.4553420473108,1.34315417741164,
-7.66267255350303));
#134072=CARTESIAN_POINT('Ctrl Pts',(-23.4157813897991,1.49224118326177,
-7.67128030487612));
#134073=CARTESIAN_POINT('Ctrl Pts',(-23.3808725778652,1.58601920182374,
-7.67704365154786));
#134074=CARTESIAN_POINT('Ctrl Pts',(-23.32425325355,1.70224247422789,-7.68430571723315));
#134075=CARTESIAN_POINT('Ctrl Pts',(-23.310598428907,1.7283464552991,-7.68594353260486));
#134076=CARTESIAN_POINT('Ctrl Pts',(-23.284792819778,1.77441749754843,-7.68882747927395));
#134077=CARTESIAN_POINT('Ctrl Pts',(-23.2729198099333,1.79452980962327,
-7.69008406577255));
#134078=CARTESIAN_POINT('Ctrl Pts',(-23.2520823567405,1.82806442713746,
-7.69216539256959));
#134079=CARTESIAN_POINT('Ctrl Pts',(-23.2433564881602,1.84162830276682,
-7.69300271423055));
#134080=CARTESIAN_POINT('Ctrl Pts',(-23.2219454670272,1.87379082615475,
-7.69497760974999));
#134081=CARTESIAN_POINT('Ctrl Pts',(-23.2090633715712,1.89225287977395,
-7.69610371153933));
#134082=CARTESIAN_POINT('Ctrl Pts',(-23.151252659042,1.97135804848215,-7.70092488448967));
#134083=CARTESIAN_POINT('Ctrl Pts',(-23.1023102094883,2.02894476856537,
-7.70442786783079));
#134084=CARTESIAN_POINT('Ctrl Pts',(-23.001492262045,2.13131074214869,-7.71108294872847));
#134085=CARTESIAN_POINT('Ctrl Pts',(-22.9504701430702,2.17667288738263,
-7.71422942256887));
#134086=CARTESIAN_POINT('Ctrl Pts',(-22.8584396223527,2.24816808717301,
-7.71976799293735));
#134087=CARTESIAN_POINT('Ctrl Pts',(-22.8188924839979,2.27601390244584,
-7.72210897050593));
#134088=CARTESIAN_POINT('Ctrl Pts',(-22.753246906146,2.31776757601064,-7.72598093632391));
#134089=CARTESIAN_POINT('Ctrl Pts',(-22.7279417435769,2.33286288751146,
-7.72747011811387));
#134090=CARTESIAN_POINT('Ctrl Pts',(-22.6759548820214,2.36188969038298,
-7.73053054398033));
#134091=CARTESIAN_POINT('Ctrl Pts',(-22.649266790528,2.37578334592831,-7.73210219678114));
#134092=CARTESIAN_POINT('Ctrl Pts',(-22.574168254494,2.41212937179847,-7.73653122830441));
#134093=CARTESIAN_POINT('Ctrl Pts',(-22.5249765339493,2.43286305957033,
-7.73944094679471));
#134094=CARTESIAN_POINT('Ctrl Pts',(-22.3835381759353,2.48401977293374,
-7.74780833457134));
#134095=CARTESIAN_POINT('Ctrl Pts',(-22.289353304043,2.50834599267184,-7.7533942681113));
#134096=CARTESIAN_POINT('Ctrl Pts',(-22.1615663346598,2.52876930529932,
-7.76068186047944));
#134097=CARTESIAN_POINT('Ctrl Pts',(-22.129461962326,2.53286968825049,-7.76248705373911));
#134098=CARTESIAN_POINT('Ctrl Pts',(-22.0724061986856,2.53833958368692,
-7.76562597878474));
#134099=CARTESIAN_POINT('Ctrl Pts',(-22.0475057349244,2.54011840849329,
-7.76697264145341));
#134100=CARTESIAN_POINT('Ctrl Pts',(-22.006140838668,2.54206607692399,-7.76915980717778));
#134101=CARTESIAN_POINT('Ctrl Pts',(-21.9896987243607,2.54257695040143,
-7.77001561273912));
#134102=CARTESIAN_POINT('Ctrl Pts',(-21.9514280502855,2.54315366996898,
-7.77197565979465));
#134103=CARTESIAN_POINT('Ctrl Pts',(-21.9296009542589,2.54301952489229,
-7.7730705668631));
#134104=CARTESIAN_POINT('Ctrl Pts',(-21.8075920309032,2.53968007434948,
-7.77909694454067));
#134105=CARTESIAN_POINT('Ctrl Pts',(-21.7078978891598,2.52718199321523,
-7.78367936087284));
#134106=CARTESIAN_POINT('Ctrl Pts',(-21.5584628593292,2.49343615451053,
-7.79082067555691));
#134107=CARTESIAN_POINT('Ctrl Pts',(-21.5074480946691,2.47912147234658,
-7.79330682532593));
#134108=CARTESIAN_POINT('Ctrl Pts',(-21.4177380503691,2.44889150373347,
-7.79786184300392));
#134109=CARTESIAN_POINT('Ctrl Pts',(-21.3787630166346,2.43397257380083,
-7.79990510100624));
#134110=CARTESIAN_POINT('Ctrl Pts',(-21.3139820648928,2.4061151292695,-7.80344067170145));
#134111=CARTESIAN_POINT('Ctrl Pts',(-21.2878470936279,2.39399855237854,
-7.80490687943469));
#134112=CARTESIAN_POINT('Ctrl Pts',(-21.2332948943076,2.36682698487295,
-7.8080597344432));
#134113=CARTESIAN_POINT('Ctrl Pts',(-21.204978631849,2.35160096991859,-7.80975147477486));
#134114=CARTESIAN_POINT('Ctrl Pts',(-21.119245398269,2.30198811074357,-7.8150518172889));
#134115=CARTESIAN_POINT('Ctrl Pts',(-21.0635782815461,2.26474549338369,
-7.81875215631224));
#134116=CARTESIAN_POINT('Ctrl Pts',(-21.0105083757967,2.22401162108585,
-7.82252260735286));
#134117=CARTESIAN_POINT('',(-23.4929996000016,1.00121063888742,-7.60402754881385));
#134118=CARTESIAN_POINT('Ctrl Pts',(-21.0105083902185,2.22401163215526,
-7.78024815277603));
#134119=CARTESIAN_POINT('Ctrl Pts',(-21.0197419184587,2.23109883809076,
-7.7796053716493));
#134120=CARTESIAN_POINT('Ctrl Pts',(-21.0290571784149,2.23808274160231,
-7.77896644365765));
#134121=CARTESIAN_POINT('Ctrl Pts',(-21.0564551693885,2.25814325226005,
-7.77711683465143));
#134122=CARTESIAN_POINT('Ctrl Pts',(-21.0747425636672,2.27093325031787,
-7.77591920883034));
#134123=CARTESIAN_POINT('Ctrl Pts',(-21.1066760886153,2.29225087703121,
-7.77389918387178));
#134124=CARTESIAN_POINT('Ctrl Pts',(-21.1201883770866,2.30096896730836,
-7.77306624663121));
#134125=CARTESIAN_POINT('Ctrl Pts',(-21.1536653251659,2.32183432985019,
-7.77105410660961));
#134126=CARTESIAN_POINT('Ctrl Pts',(-21.1737736744045,2.33374199468929,
-7.76988830108668));
#134127=CARTESIAN_POINT('Ctrl Pts',(-21.2198207051163,2.35961557186169,
-7.76729699303873));
#134128=CARTESIAN_POINT('Ctrl Pts',(-21.245904612514,2.37330482217105,-7.76588339996987));
#134129=CARTESIAN_POINT('Ctrl Pts',(-21.3413995460949,2.41998555348903,
-7.76084830321388));
#134130=CARTESIAN_POINT('Ctrl Pts',(-21.4128598593125,2.44852845345996,
-7.75733619977407));
#134131=CARTESIAN_POINT('Ctrl Pts',(-21.5537504719334,2.49293636181643,
-7.75046189238699));
#134132=CARTESIAN_POINT('Ctrl Pts',(-21.6227336739363,2.50955898666401,
-7.74711726701255));
#134133=CARTESIAN_POINT('Ctrl Pts',(-21.7244611107527,2.52676935584913,
-7.74204961207007));
#134134=CARTESIAN_POINT('Ctrl Pts',(-21.7564710493216,2.53115604148476,
-7.74043680514408));
#134135=CARTESIAN_POINT('Ctrl Pts',(-21.8167641829495,2.53749782510377,
-7.73735346131916));
#134136=CARTESIAN_POINT('Ctrl Pts',(-21.8450095454325,2.53968445416299,
-7.73589048002731));
#134137=CARTESIAN_POINT('Ctrl Pts',(-21.9129133037364,2.54306410630991,
-7.73232374112381));
#134138=CARTESIAN_POINT('Ctrl Pts',(-21.9525873905057,2.54350743791063,
-7.73019902524178));
#134139=CARTESIAN_POINT('Ctrl Pts',(-22.0409683647097,2.54108751699568,
-7.72537519877531));
#134140=CARTESIAN_POINT('Ctrl Pts',(-22.0896108143746,2.53744407769253,
-7.72265837686186));
#134141=CARTESIAN_POINT('Ctrl Pts',(-22.2237099944816,2.52098301537759,
-7.71503710853011));
#134142=CARTESIAN_POINT('Ctrl Pts',(-22.3083873242692,2.50328470266827,
-7.71006781788095));
#134143=CARTESIAN_POINT('Ctrl Pts',(-22.4259304090191,2.46821574170422,
-7.70321968796503));
#134144=CARTESIAN_POINT('Ctrl Pts',(-22.4603470330766,2.45661026094603,
-7.70122256125562));
#134145=CARTESIAN_POINT('Ctrl Pts',(-22.5109493811257,2.43753278314046,
-7.69832874573481));
#134146=CARTESIAN_POINT('Ctrl Pts',(-22.5274659299164,2.4309779405036,-7.69739117791553));
#134147=CARTESIAN_POINT('Ctrl Pts',(-22.5602659327625,2.41730033281319,
-7.69554850763487));
#134148=CARTESIAN_POINT('Ctrl Pts',(-22.5765469386756,2.41017861599385,
-7.69464356527523));
#134149=CARTESIAN_POINT('Ctrl Pts',(-22.6258229610287,2.38760211544239,
-7.6919242610315));
#134150=CARTESIAN_POINT('Ctrl Pts',(-22.6583982163992,2.37125803393056,
-7.69015368986645));
#134151=CARTESIAN_POINT('Ctrl Pts',(-22.742773382217,2.32511409832406,-7.68556609088079));
#134152=CARTESIAN_POINT('Ctrl Pts',(-22.7934741572237,2.29343298809316,
-7.68280645716952));
#134153=CARTESIAN_POINT('Ctrl Pts',(-22.9129322814421,2.20876961904608,
-7.67602684285459));
#134154=CARTESIAN_POINT('Ctrl Pts',(-22.9793004999558,2.15278002644172,
-7.67200483924843));
#134155=CARTESIAN_POINT('Ctrl Pts',(-23.0653973436928,2.06675456468141,
-7.66607621203001));
#134156=CARTESIAN_POINT('Ctrl Pts',(-23.0893295966423,2.04115531288518,
-7.66434025154041));
#134157=CARTESIAN_POINT('Ctrl Pts',(-23.1308013119013,1.99365127050742,
-7.6611524413116));
#134158=CARTESIAN_POINT('Ctrl Pts',(-23.148654227675,1.97204038054973,-7.65971387821901));
#134159=CARTESIAN_POINT('Ctrl Pts',(-23.1877033287463,1.92205900344857,
-7.65640690763637));
#134160=CARTESIAN_POINT('Ctrl Pts',(-23.2085308171283,1.89342165939779,
-7.65452588400141));
#134161=CARTESIAN_POINT('Ctrl Pts',(-23.2511851465789,1.830318241846,-7.65040758639692));
#134162=CARTESIAN_POINT('Ctrl Pts',(-23.2726672903487,1.79565197934347,
-7.64816103474137));
#134163=CARTESIAN_POINT('Ctrl Pts',(-23.3406178280417,1.67562656014211,
-7.6404546928881));
#134164=CARTESIAN_POINT('Ctrl Pts',(-23.3803893676498,1.58674873226413,
-7.63485102634545));
#134165=CARTESIAN_POINT('Ctrl Pts',(-23.4244437981223,1.45660101062369,
-7.62713234020692));
#134166=CARTESIAN_POINT('Ctrl Pts',(-23.4358526985855,1.41798463828813,
-7.62490189634416));
#134167=CARTESIAN_POINT('Ctrl Pts',(-23.4504195209111,1.36049064100476,
-7.62170827403076));
#134168=CARTESIAN_POINT('Ctrl Pts',(-23.4547575886915,1.34193114230808,
-7.62069656021869));
#134169=CARTESIAN_POINT('Ctrl Pts',(-23.4622680333557,1.30688147646575,
-7.6188279000062));
#134170=CARTESIAN_POINT('Ctrl Pts',(-23.4655170783054,1.29041150155825,
-7.61796762642306));
#134171=CARTESIAN_POINT('Ctrl Pts',(-23.4738006666381,1.24448599846408,
-7.61561124648096));
#134172=CARTESIAN_POINT('Ctrl Pts',(-23.4782495619118,1.21493103208098,
-7.61414265623193));
#134173=CARTESIAN_POINT('Ctrl Pts',(-23.4892237504235,1.12419200102315,
-7.6097314109794));
#134174=CARTESIAN_POINT('Ctrl Pts',(-23.4929512956989,1.06273095523487,
-7.60687664523302));
#134175=CARTESIAN_POINT('Ctrl Pts',(-23.4929995464514,1.00121017463365,
-7.6040274338919));
#134176=CARTESIAN_POINT('Ctrl Pts',(-23.4929995460838,1.00121064316225,
-7.60402745559086));
#134177=CARTESIAN_POINT('Ctrl Pts',(-23.4930596419354,0.924616752090264,
-7.60048016335937));
#134178=CARTESIAN_POINT('Ctrl Pts',(-23.4874164958633,0.848124290790459,
-7.59694687164609));
#134179=CARTESIAN_POINT('Ctrl Pts',(-23.4697312634755,0.729556736793429,
-7.59120813810576));
#134180=CARTESIAN_POINT('Ctrl Pts',(-23.4615473628301,0.687035361430817,
-7.58909752211753));
#134181=CARTESIAN_POINT('Ctrl Pts',(-23.4449882882033,0.617009942846924,
-7.58550120388002));
#134182=CARTESIAN_POINT('Ctrl Pts',(-23.4376128968803,0.589294386240042,
-7.5840458793293));
#134183=CARTESIAN_POINT('Ctrl Pts',(-23.4207027905572,0.532201560820202,
-7.58097429083855));
#134184=CARTESIAN_POINT('Ctrl Pts',(-23.4110498168629,0.502872916424515,
-7.57935491829063));
#134185=CARTESIAN_POINT('Ctrl Pts',(-23.3795675010402,0.416079660239683,
-7.57443241543105));
#134186=CARTESIAN_POINT('Ctrl Pts',(-23.3551797296148,0.359613451613856,
-7.57105294541982));
#134187=CARTESIAN_POINT('Ctrl Pts',(-23.2879466423569,0.226404038537122,
-7.56268307598321));
#134188=CARTESIAN_POINT('Ctrl Pts',(-23.2417901228115,0.151572394266637,
-7.55763195629812));
#134189=CARTESIAN_POINT('Ctrl Pts',(-23.1710100165528,0.0560985072348075,
-7.55094334657079));
#134190=CARTESIAN_POINT('Ctrl Pts',(-23.1517446042031,0.0316893280978903,
-7.54921065594732));
#134191=CARTESIAN_POINT('Ctrl Pts',(-23.1161658143576,-0.0106899147818895,
-7.5461828076401));
#134192=CARTESIAN_POINT('Ctrl Pts',(-23.1001412057038,-0.0288887877254895,
-7.54487575978468));
#134193=CARTESIAN_POINT('Ctrl Pts',(-23.0727342685971,-0.0585734818121564,
-7.54274289611917));
#134194=CARTESIAN_POINT('Ctrl Pts',(-23.0615892832405,-0.0702707033213201,
-7.54190266586779));
#134195=CARTESIAN_POINT('Ctrl Pts',(-23.0352876493887,-0.0970213781877094,
-7.53998232383929));
#134196=CARTESIAN_POINT('Ctrl Pts',(-23.0199987346164,-0.111938837198471,
-7.53891124202531));
#134197=CARTESIAN_POINT('Ctrl Pts',(-22.9387089639375,-0.188023740955705,
-7.53341694542624));
#134198=CARTESIAN_POINT('Ctrl Pts',(-22.8677548878983,-0.243653730995503,
-7.52928309846972));
#134199=CARTESIAN_POINT('Ctrl Pts',(-22.7416118789101,-0.325845829355833,
-7.5223109031778));
#134200=CARTESIAN_POINT('Ctrl Pts',(-22.6889715804988,-0.355889789636206,
-7.5194987778821));
#134201=CARTESIAN_POINT('Ctrl Pts',(-22.5942224235777,-0.402806846620529,
-7.51445243134997));
#134202=CARTESIAN_POINT('Ctrl Pts',(-22.5528827945077,-0.421063509037571,
-7.51225599094274));
#134203=CARTESIAN_POINT('Ctrl Pts',(-22.483851918244,-0.447994515079917,
-7.50855925863481));
#134204=CARTESIAN_POINT('Ctrl Pts',(-22.4566108628926,-0.457748703528487,
-7.50709354417815));
#134205=CARTESIAN_POINT('Ctrl Pts',(-22.4001741632374,-0.476183945786,-7.50403567366152));
#134206=CARTESIAN_POINT('Ctrl Pts',(-22.3709635723084,-0.484777869885602,
-7.50244158152876));
#134207=CARTESIAN_POINT('Ctrl Pts',(-22.2860445492342,-0.507054171364554,
-7.49776978629059));
#134208=CARTESIAN_POINT('Ctrl Pts',(-22.2298065628716,-0.518501072663407,
-7.49462817013797));
#134209=CARTESIAN_POINT('Ctrl Pts',(-22.0816744032439,-0.54014336215404,
-7.48626170914276));
#134210=CARTESIAN_POINT('Ctrl Pts',(-21.9892694060592,-0.545262569073013,
-7.48094383685638));
#134211=CARTESIAN_POINT('Ctrl Pts',(-21.8652805946514,-0.540998683831635,
-7.47395724803011));
#134212=CARTESIAN_POINT('Ctrl Pts',(-21.833632184854,-0.538932429006236,
-7.47218857410449));
#134213=CARTESIAN_POINT('Ctrl Pts',(-21.7776066803395,-0.533536265839936,
-7.46910652516652));
#134214=CARTESIAN_POINT('Ctrl Pts',(-21.753203110952,-0.530595976630233,
-7.46778070139841));
#134215=CARTESIAN_POINT('Ctrl Pts',(-21.7128621329344,-0.524754583934963,
-7.46562774297288));
#134216=CARTESIAN_POINT('Ctrl Pts',(-21.6968827208267,-0.52218350221434,
-7.46478553566933));
#134217=CARTESIAN_POINT('Ctrl Pts',(-21.6601181541629,-0.515673070150711,
-7.46287333248927));
#134218=CARTESIAN_POINT('Ctrl Pts',(-21.6393685425915,-0.511556985091568,
-7.46181190417512));
#134219=CARTESIAN_POINT('Ctrl Pts',(-21.4977492012223,-0.48042446424839,
-7.4546513588263));
#134220=CARTESIAN_POINT('Ctrl Pts',(-21.3804193312323,-0.439364994380878,
-7.44910895372614));
#134221=CARTESIAN_POINT('Ctrl Pts',(-21.2133162502117,-0.357214475686276,
-7.44039005712894));
#134222=CARTESIAN_POINT('Ctrl Pts',(-21.159100921515,-0.326352839384203,
-7.43742060166912));
#134223=CARTESIAN_POINT('Ctrl Pts',(-21.0809655232895,-0.27537726297433,
-7.43281600339389));
#134224=CARTESIAN_POINT('Ctrl Pts',(-21.0555442391294,-0.257679137889282,
-7.43126282256385));
#134225=CARTESIAN_POINT('Ctrl Pts',(-21.0079164800827,-0.222346313620481,
-7.42823552736711));
#134226=CARTESIAN_POINT('Ctrl Pts',(-20.9856296930827,-0.204840921398022,
-7.42676652770496));
#134227=CARTESIAN_POINT('Ctrl Pts',(-20.9309961724158,-0.159441068286679,
-7.42302628650033));
#134228=CARTESIAN_POINT('Ctrl Pts',(-20.8993032888504,-0.130799881715213,
-7.42072719012891));
#134229=CARTESIAN_POINT('Ctrl Pts',(-20.7935830929418,-0.0269737837130934,
-7.41259657298036));
#134230=CARTESIAN_POINT('Ctrl Pts',(-20.7261072175214,0.0544535774880694,
-7.40654040341755));
#134231=CARTESIAN_POINT('Ctrl Pts',(-20.6464690772227,0.173511678049652,
-7.39842668985596));
#134232=CARTESIAN_POINT('Ctrl Pts',(-20.6266264646943,0.205671018122708,
-7.39630314709043));
#134233=CARTESIAN_POINT('Ctrl Pts',(-20.5943527970144,0.26255001077216,
-7.39269859444294));
#134234=CARTESIAN_POINT('Ctrl Pts',(-20.5813688297038,0.286935688463927,
-7.39119904248992));
#134235=CARTESIAN_POINT('Ctrl Pts',(-20.5616918804516,0.326411656098937,
-7.38885854109423));
#134236=CARTESIAN_POINT('Ctrl Pts',(-20.5545744222045,0.341282889580845,
-7.38799620917483));
#134237=CARTESIAN_POINT('Ctrl Pts',(-20.5394054038096,0.374326981356683,
-7.38612554047329));
#134238=CARTESIAN_POINT('Ctrl Pts',(-20.531464135058,0.392546370859086,
-7.38512285810854));
#134239=CARTESIAN_POINT('Ctrl Pts',(-20.5040987168699,0.458795644155141,
-7.38156277947558));
#134240=CARTESIAN_POINT('Ctrl Pts',(-20.4867431580902,0.507645615271635,
-7.37909756278097));
#134241=CARTESIAN_POINT('Ctrl Pts',(-20.4413405371832,0.659232453935692,
-7.37168556082397));
#134242=CARTESIAN_POINT('Ctrl Pts',(-20.4214344297855,0.764068975997816,
-7.3668630803487));
#134243=CARTESIAN_POINT('Ctrl Pts',(-20.4088304832659,0.91327570661631,
-7.3596948681011));
#134244=CARTESIAN_POINT('Ctrl Pts',(-20.4070037615243,0.956562532668586,
-7.35758308081218));
#134245=CARTESIAN_POINT('Ctrl Pts',(-20.4069975768245,1.02827379355278,
-7.35399898070112));
#134246=CARTESIAN_POINT('Ctrl Pts',(-20.4077795851932,1.05667405076351,
-7.35255750368066));
#134247=CARTESIAN_POINT('Ctrl Pts',(-20.4110421353416,1.11578425703944,
-7.34950458738404));
#134248=CARTESIAN_POINT('Ctrl Pts',(-20.4136593613833,1.1464737999966,-7.34788972301113));
#134249=CARTESIAN_POINT('Ctrl Pts',(-20.4241509379542,1.23729766619312,
-7.34301693987845));
#134250=CARTESIAN_POINT('Ctrl Pts',(-20.4346527686506,1.29706423016573,
-7.3396852899364));
#134251=CARTESIAN_POINT('Ctrl Pts',(-20.4751389248404,1.4677806731414,-7.32985087727042));
#134252=CARTESIAN_POINT('Ctrl Pts',(-20.5140225278048,1.57619581321561,
-7.32318230675));
#134253=CARTESIAN_POINT('Ctrl Pts',(-20.5764537348811,1.70352544961722,
-7.31537569807187));
#134254=CARTESIAN_POINT('Ctrl Pts',(-20.5889702902008,1.72744462915774,
-7.31391214165409));
#134255=CARTESIAN_POINT('Ctrl Pts',(-20.6100952404935,1.76535836747691,
-7.31161110467496));
#134256=CARTESIAN_POINT('Ctrl Pts',(-20.6183104045863,1.77956468469998,
-7.31075356003251));
#134257=CARTESIAN_POINT('Ctrl Pts',(-20.6371163776265,1.81092022924765,
-7.3088739979586));
#134258=CARTESIAN_POINT('Ctrl Pts',(-20.6478192327962,1.82799779439238,
-7.30785827798668));
#134259=CARTESIAN_POINT('Ctrl Pts',(-20.6923015762068,1.89597721645553,
-7.30382789631088));
#134260=CARTESIAN_POINT('Ctrl Pts',(-20.7287577906987,1.94506566056608,
-7.300945846947));
#134261=CARTESIAN_POINT('Ctrl Pts',(-20.840188010109,2.0778527740842,-7.29287114832312));
#134262=CARTESIAN_POINT('Ctrl Pts',(-20.921495780058,2.15568989360413,-7.28776554622509));
#134263=CARTESIAN_POINT('Ctrl Pts',(-21.0105083871506,2.22401162980051,
-7.28231522554091));
#134264=CARTESIAN_POINT('Origin',(-21.9500000210213,0.999999999999992,-4.89578827641128));
#134265=CARTESIAN_POINT('',(-21.010508379234,2.22401162372414,-6.7805154429392));
#134266=CARTESIAN_POINT('',(-21.0105469284169,2.2239496744092,-6.82271756118853));
#134267=CARTESIAN_POINT('',(-21.0105083758276,2.22401162110953,-4.89578827641128));
#134268=CARTESIAN_POINT('',(-23.4934928036937,1.00049669217445,-7.14664973949428));
#134269=CARTESIAN_POINT('Ctrl Pts',(-21.0105469284169,2.2239496744092,-6.82271756118853));
#134270=CARTESIAN_POINT('Ctrl Pts',(-20.9646994282928,2.18892255442207,
-6.82591631418018));
#134271=CARTESIAN_POINT('Ctrl Pts',(-20.9208499519301,2.15135842051501,
-6.82913507944199));
#134272=CARTESIAN_POINT('Ctrl Pts',(-20.8792997883414,2.11149720384009,
-6.83231398513469));
#134273=CARTESIAN_POINT('Ctrl Pts',(-20.8402565375944,2.07404099805647,
-6.83530109279786));
#134274=CARTESIAN_POINT('Ctrl Pts',(-20.8032432753279,2.03455597882077,
-6.838252529876));
#134275=CARTESIAN_POINT('Ctrl Pts',(-20.7684942010589,1.99327442215102,
-6.84110588764712));
#134276=CARTESIAN_POINT('Ctrl Pts',(-20.7662034820682,1.99055307063837,
-6.8412939859194));
#134277=CARTESIAN_POINT('Ctrl Pts',(-20.7639225844739,1.98782390653865,
-6.84148165797097));
#134278=CARTESIAN_POINT('Ctrl Pts',(-20.7616515677829,1.98508699390259,
-6.84166888592334));
#134279=CARTESIAN_POINT('Ctrl Pts',(-20.7545421303374,1.97651906516054,
-6.84225500465191));
#134280=CARTESIAN_POINT('Ctrl Pts',(-20.7475296520023,1.96787539299453,
-6.8428367407542));
#134281=CARTESIAN_POINT('Ctrl Pts',(-20.7406160611608,1.95915820811847,
-6.84341351093467));
#134282=CARTESIAN_POINT('Ctrl Pts',(-20.740605526905,1.95914492572187,-6.84341438976085));
#134283=CARTESIAN_POINT('Ctrl Pts',(-20.740594992867,1.95913164314035,-6.84341526857625));
#134284=CARTESIAN_POINT('Ctrl Pts',(-20.7405844590468,1.9591183603739,-6.84341614738087));
#134285=CARTESIAN_POINT('Ctrl Pts',(-20.7081586236352,1.91823055425673,
-6.84612133631287));
#134286=CARTESIAN_POINT('Ctrl Pts',(-20.6777965480067,1.87558611519414,
-6.84872437076239));
#134287=CARTESIAN_POINT('Ctrl Pts',(-20.6496700737443,1.83143437663984,
-6.85127674573291));
#134288=CARTESIAN_POINT('Ctrl Pts',(-20.6468302132197,1.82697648482437,
-6.8515344527194));
#134289=CARTESIAN_POINT('Ctrl Pts',(-20.6440131428578,1.82250327075007,
-6.8517916432608));
#134290=CARTESIAN_POINT('Ctrl Pts',(-20.6412190384027,1.81801502047479,
-6.85204837036131));
#134291=CARTESIAN_POINT('Ctrl Pts',(-20.6107934927671,1.7691415922377,-6.85484392157923));
#134292=CARTESIAN_POINT('Ctrl Pts',(-20.5830908180337,1.71847954347281,
-6.8575852240484));
#134293=CARTESIAN_POINT('Ctrl Pts',(-20.5582897697873,1.6663800599524,-6.8603324033392));
#134294=CARTESIAN_POINT('Ctrl Pts',(-20.5335117049533,1.61432885761366,
-6.86307703678782));
#134295=CARTESIAN_POINT('Ctrl Pts',(-20.5116295026666,1.56084318426877,
-6.86582797361469));
#134296=CARTESIAN_POINT('Ctrl Pts',(-20.4927783481858,1.5062830339907,-6.86862837225068));
#134297=CARTESIAN_POINT('Ctrl Pts',(-20.4739375418887,1.45175283405081,
-6.87142723363127));
#134298=CARTESIAN_POINT('Ctrl Pts',(-20.4581242020584,1.39614948283325,
-6.87427573809505));
#134299=CARTESIAN_POINT('Ctrl Pts',(-20.4454350789399,1.33983891146091,
-6.87719520358442));
#134300=CARTESIAN_POINT('Ctrl Pts',(-20.4327481282639,1.2835379807448,-6.88011416924645));
#134301=CARTESIAN_POINT('Ctrl Pts',(-20.4231842050893,1.22653013640785,
-6.88310416118364));
#134302=CARTESIAN_POINT('Ctrl Pts',(-20.4168045934839,1.16918611131505,
-6.88616231760585));
#134303=CARTESIAN_POINT('Ctrl Pts',(-20.4104194018568,1.11179192942249,
-6.8892231488898));
#134304=CARTESIAN_POINT('Ctrl Pts',(-20.4072241165769,1.05406098363771,
-6.89235222984401));
#134305=CARTESIAN_POINT('Ctrl Pts',(-20.4072454428099,0.996369467827194,
-6.89552205244813));
#134306=CARTESIAN_POINT('Ctrl Pts',(-20.4072667787057,0.938651812469348,
-6.89869331127257));
#134307=CARTESIAN_POINT('Ctrl Pts',(-20.410507835263,0.880973587345166,
-6.90190515928954));
#134308=CARTESIAN_POINT('Ctrl Pts',(-20.4169590402013,0.823716245000039,
-6.90510703379557));
#134309=CARTESIAN_POINT('Ctrl Pts',(-20.4234214586073,0.766359378089729,
-6.90831447379162));
#134310=CARTESIAN_POINT('Ctrl Pts',(-20.433105639191,0.709424852376949,
-6.91151149706294));
#134311=CARTESIAN_POINT('Ctrl Pts',(-20.4459607908488,0.653301304988339,
-6.91462858291627));
#134312=CARTESIAN_POINT('Ctrl Pts',(-20.4543194584833,0.616808691631712,
-6.91665537227897));
#134313=CARTESIAN_POINT('Ctrl Pts',(-20.4640179374223,0.580659075490424,
-6.91864797005291));
#134314=CARTESIAN_POINT('Ctrl Pts',(-20.4750312470688,0.544960268935724,
-6.92058466143602));
#134315=CARTESIAN_POINT('Ctrl Pts',(-20.4750362446744,0.544944069577026,
-6.92058554026535));
#134316=CARTESIAN_POINT('Ctrl Pts',(-20.4750412425556,0.544927870293381,
-6.9205864190839));
#134317=CARTESIAN_POINT('Ctrl Pts',(-20.4750462407125,0.544911671084798,
-6.92058729789167));
#134318=CARTESIAN_POINT('Ctrl Pts',(-20.4904318029095,0.495046503635593,
-6.92329248539754));
#134319=CARTESIAN_POINT('Ctrl Pts',(-20.5084332001617,0.445890056417994,
-6.92589551891448));
#134320=CARTESIAN_POINT('Ctrl Pts',(-20.5289419697622,0.397725053238161,
-6.92844789334448));
#134321=CARTESIAN_POINT('Ctrl Pts',(-20.5310126811773,0.392861971549898,
-6.92870559924156));
#134322=CARTESIAN_POINT('Ctrl Pts',(-20.5331089172014,0.388009021327957,
-6.92896278870169));
#134323=CARTESIAN_POINT('Ctrl Pts',(-20.5352305412919,0.383166509278513,
-6.92921951472834));
#134324=CARTESIAN_POINT('Ctrl Pts',(-20.5583334033085,0.330435260516698,
-6.93201506460749));
#134325=CARTESIAN_POINT('Ctrl Pts',(-20.58445120499,0.278938245314851,-6.93475636620834));
#134326=CARTESIAN_POINT('Ctrl Pts',(-20.6133953906851,0.229021486521721,
-6.93750354492877));
#134327=CARTESIAN_POINT('Ctrl Pts',(-20.6423127544647,0.179150984448229,
-6.94024817790147));
#134328=CARTESIAN_POINT('Ctrl Pts',(-20.674050798609,0.130857661063998,
-6.94299911455059));
#134329=CARTESIAN_POINT('Ctrl Pts',(-20.7083890639754,0.0844565855523038,
-6.94579951316334));
#134330=CARTESIAN_POINT('Ctrl Pts',(-20.742708480812,0.0380809799369405,
-6.94859837461641));
#134331=CARTESIAN_POINT('Ctrl Pts',(-20.7796250004785,-0.0064045817375827,
-6.95144687931098));
#134332=CARTESIAN_POINT('Ctrl Pts',(-20.8188915324266,-0.0487133722867088,
-6.95436634506362));
#134333=CARTESIAN_POINT('Ctrl Pts',(-20.8581513430867,-0.0910149208016234,
-6.95728531108864));
#134334=CARTESIAN_POINT('Ctrl Pts',(-20.8997602408799,-0.13114050550213,
-6.96027530342673));
#134335=CARTESIAN_POINT('Ctrl Pts',(-20.9434471190817,-0.168829934658833,
-6.96333346016748));
#134336=CARTESIAN_POINT('Ctrl Pts',(-20.9871722109337,-0.206552331395789,
-6.96639429192958));
#134337=CARTESIAN_POINT('Ctrl Pts',(-21.0329789281761,-0.241834287798403,
-6.96952337328719));
#134338=CARTESIAN_POINT('Ctrl Pts',(-21.0805721059298,-0.274441042978287,
-6.97269319608993));
#134339=CARTESIAN_POINT('Ctrl Pts',(-21.1281868491517,-0.307062572963616,
-6.97586445520593));
#134340=CARTESIAN_POINT('Ctrl Pts',(-21.1775898109862,-0.337006337150968,
-6.97907630331255));
#134341=CARTESIAN_POINT('Ctrl Pts',(-21.2284609747694,-0.364064520778986,
-6.98227817755357));
#134342=CARTESIAN_POINT('Ctrl Pts',(-21.2794205649908,-0.391169738102013,
-6.98548561742969));
#134343=CARTESIAN_POINT('Ctrl Pts',(-21.331853722017,-0.415378971384698,
-6.98868264022486));
#134344=CARTESIAN_POINT('Ctrl Pts',(-21.3854111946562,-0.436514338276396,
-6.99179972505387));
#134345=CARTESIAN_POINT('Ctrl Pts',(-21.4202352931566,-0.450256960215189,
-6.99382651354427));
#134346=CARTESIAN_POINT('Ctrl Pts',(-21.4555341619196,-0.462700608224986,
-6.9958191102204));
#134347=CARTESIAN_POINT('Ctrl Pts',(-21.491204756158,-0.473804917728884,
-6.99775580022609));
#134348=CARTESIAN_POINT('Ctrl Pts',(-21.4912209426116,-0.473809956596179,
-6.99775667904921));
#134349=CARTESIAN_POINT('Ctrl Pts',(-21.4912371291592,-0.47381499519367,
-6.99775755786155));
#134350=CARTESIAN_POINT('Ctrl Pts',(-21.4912533158008,-0.473820033521343,
-6.99775843666311));
#134351=CARTESIAN_POINT('Ctrl Pts',(-21.5410800807606,-0.489329338961987,
-7.00046362034064));
#134352=CARTESIAN_POINT('Ctrl Pts',(-21.5918015719565,-0.502280458528975,
-7.00306664967207));
#134353=CARTESIAN_POINT('Ctrl Pts',(-21.6431232786224,-0.512602967705018,
-7.00561901926318));
#134354=CARTESIAN_POINT('Ctrl Pts',(-21.6483051918672,-0.513645223516332,
-7.00587673005749));
#134355=CARTESIAN_POINT('Ctrl Pts',(-21.6534931835026,-0.514660697509918,
-7.0061339243866));
#134356=CARTESIAN_POINT('Ctrl Pts',(-21.6586869233386,-0.515649328854675,
-7.00639065525699));
#134357=CARTESIAN_POINT('Ctrl Pts',(-21.7152416978683,-0.526414562493791,
-7.00918620469696));
#134358=CARTESIAN_POINT('Ctrl Pts',(-21.7724834763618,-0.533995261557184,
-7.01192750496353));
#134359=CARTESIAN_POINT('Ctrl Pts',(-21.8300202479235,-0.53835126258365,
-7.01467468168719));
#134360=CARTESIAN_POINT('Ctrl Pts',(-21.8875036999948,-0.542703226891542,
-7.01741931259434));
#134361=CARTESIAN_POINT('Ctrl Pts',(-21.9452814580753,-0.543836937871541,
-7.02017024652085));
#134362=CARTESIAN_POINT('Ctrl Pts',(-22.0029689990605,-0.541756048795133,
-7.0229706421471));
#134363=CARTESIAN_POINT('Ctrl Pts',(-22.0606248733005,-0.539676301992831,
-7.02576950053649));
#134364=CARTESIAN_POINT('Ctrl Pts',(-22.1181905847057,-0.534385773536387,
-7.02861800190396));
#134365=CARTESIAN_POINT('Ctrl Pts',(-22.1752899253371,-0.525926108334006,
-7.03153746456503));
#134366=CARTESIAN_POINT('Ctrl Pts',(-22.2323794904752,-0.51746789143909,
-7.03445642740968));
#134367=CARTESIAN_POINT('Ctrl Pts',(-22.2890028275311,-0.505841757544152,
-7.03744641680038));
#134368=CARTESIAN_POINT('Ctrl Pts',(-22.3447920326749,-0.491124164652751,
-7.04050457139828));
#134369=CARTESIAN_POINT('Ctrl Pts',(-22.4006300344293,-0.476393698865109,
-7.04356540084301));
#134370=CARTESIAN_POINT('Ctrl Pts',(-22.4556324317036,-0.458566345186209,
-7.0466944806829));
#134371=CARTESIAN_POINT('Ctrl Pts',(-22.509438690026,-0.437752784647632,
-7.0498643033953));
#134372=CARTESIAN_POINT('Ctrl Pts',(-22.563269327466,-0.416929793677423,
-7.05303556232504));
#134373=CARTESIAN_POINT('Ctrl Pts',(-22.6159027050888,-0.393117695772129,
-7.05624741167359));
#134374=CARTESIAN_POINT('Ctrl Pts',(-22.6669864586967,-0.366462906402016,
-7.05944928924691));
#134375=CARTESIAN_POINT('Ctrl Pts',(-22.7181590051619,-0.339761786158799,
-7.06265673226596));
#134376=CARTESIAN_POINT('Ctrl Pts',(-22.7677763813216,-0.310207666983498,
-7.06585376030648));
#134377=CARTESIAN_POINT('Ctrl Pts',(-22.8154943778053,-0.277988002117594,
-7.06897085315136));
#134378=CARTESIAN_POINT('Ctrl Pts',(-22.8465210788424,-0.257038465612008,
-7.07099761694971));
#134379=CARTESIAN_POINT('Ctrl Pts',(-22.8767449536752,-0.234962827962764,
-7.07299019111136));
#134380=CARTESIAN_POINT('Ctrl Pts',(-22.9060744440312,-0.211823246532039,
-7.07492686191659));
#134381=CARTESIAN_POINT('Ctrl Pts',(-22.9060877521632,-0.21181274704497,
-7.07492774067277));
#134382=CARTESIAN_POINT('Ctrl Pts',(-22.9061010601267,-0.211802247327223,
-7.0749286194182));
#134383=CARTESIAN_POINT('Ctrl Pts',(-22.9061143679217,-0.211791747378802,
-7.07492949815289));
#134384=CARTESIAN_POINT('Ctrl Pts',(-22.9468357822309,-0.179662251027165,
-7.07761839737488));
#134385=CARTESIAN_POINT('Ctrl Pts',(-22.9859801592963,-0.145368599613194,
-7.08020673534755));
#134386=CARTESIAN_POINT('Ctrl Pts',(-23.0233229641384,-0.10911017788726,
-7.08274491630824));
#134387=CARTESIAN_POINT('Ctrl Pts',(-23.0275410591066,-0.105014570530441,
-7.0830316191519));
#134388=CARTESIAN_POINT('Ctrl Pts',(-23.0317361566911,-0.100893948133087,
-7.083317682039));
#134389=CARTESIAN_POINT('Ctrl Pts',(-23.0359079259895,-0.0967486390692106,
-7.08360317761281));
#134390=CARTESIAN_POINT('Ctrl Pts',(-23.0763795485599,-0.0565337154069281,
-7.08637285836026));
#134391=CARTESIAN_POINT('Ctrl Pts',(-23.1146571956832,-0.0139898798970523,
-7.08908982186985));
#134392=CARTESIAN_POINT('Ctrl Pts',(-23.150488725235,0.0305884411469265,
-7.09181244443254));
#134393=CARTESIAN_POINT('Ctrl Pts',(-23.1862876935111,0.0751262524214138,
-7.09453259285961));
#134394=CARTESIAN_POINT('Ctrl Pts',(-23.2196452613176,0.121694460344611,
-7.09725881554214));
#134395=CARTESIAN_POINT('Ctrl Pts',(-23.2503495102397,0.169979309385704,
-7.10003316983043));
#134396=CARTESIAN_POINT('Ctrl Pts',(-23.2810380611888,0.218239472128002,
-7.10280610569161));
#134397=CARTESIAN_POINT('Ctrl Pts',(-23.3090761954244,0.268214298768575,
-7.10562735425302));
#134398=CARTESIAN_POINT('Ctrl Pts',(-23.3342883246752,0.319574916103118,
-7.10851790109925));
#134399=CARTESIAN_POINT('Ctrl Pts',(-23.3602550446221,0.372472739740242,
-7.11149496105729));
#134400=CARTESIAN_POINT('Ctrl Pts',(-23.3832239786204,0.426840488413619,
-7.11454575062313));
#134401=CARTESIAN_POINT('Ctrl Pts',(-23.4030409202316,0.482304364683225,
-7.11766728314441));
#134402=CARTESIAN_POINT('Ctrl Pts',(-23.4222963531123,0.536196684081849,
-7.12070036772061));
#134403=CARTESIAN_POINT('Ctrl Pts',(-23.4385760267113,0.591123798865315,
-7.12380008299715));
#134404=CARTESIAN_POINT('Ctrl Pts',(-23.4517724941886,0.646730648522823,
-7.12693955632812));
#134405=CARTESIAN_POINT('Ctrl Pts',(-23.4655461960298,0.704769829752706,
-7.13021635518913));
#134406=CARTESIAN_POINT('Ctrl Pts',(-23.4759605798014,0.763549655735676,
-7.13353642047766));
#134407=CARTESIAN_POINT('Ctrl Pts',(-23.4829341020971,0.822652425744619,
-7.13684359595235));
#134408=CARTESIAN_POINT('Ctrl Pts',(-23.4894646191262,0.878000588358255,
-7.13994067728945));
#134409=CARTESIAN_POINT('Ctrl Pts',(-23.4929774206621,0.933632566162483,
-7.14302600958895));
#134410=CARTESIAN_POINT('Ctrl Pts',(-23.4934429988996,0.989191194661555,
-7.14603647098282));
#134411=CARTESIAN_POINT('Ctrl Pts',(-23.4934745819443,0.992960079256549,
-7.14624068915519));
#134412=CARTESIAN_POINT('Ctrl Pts',(-23.4934921520323,0.996728643780493,
-7.14644456279066));
#134413=CARTESIAN_POINT('Ctrl Pts',(-23.4934957039329,1.00049678448525,
-7.14664807218481));
#134414=CARTESIAN_POINT('Ctrl Pts',(-23.4929999460485,1.00048100516412,
-7.1469330768822));
#134415=CARTESIAN_POINT('Ctrl Pts',(-23.492995606971,1.01440018264177,-7.14769520777935));
#134416=CARTESIAN_POINT('Ctrl Pts',(-23.4928029234977,1.02831911176174,
-7.14845097177061));
#134417=CARTESIAN_POINT('Ctrl Pts',(-23.4920747206752,1.05491373269753,
-7.14988057379478));
#134418=CARTESIAN_POINT('Ctrl Pts',(-23.4915711760172,1.06758912955807,
-7.15055567525103));
#134419=CARTESIAN_POINT('Ctrl Pts',(-23.4901195877529,1.09545912419696,
-7.15202419674145));
#134420=CARTESIAN_POINT('Ctrl Pts',(-23.4891029406518,1.11064793043558,
-7.15281367016478));
#134421=CARTESIAN_POINT('Ctrl Pts',(-23.4860264450462,1.14825076246317,
-7.15474174833385));
#134422=CARTESIAN_POINT('Ctrl Pts',(-23.4837007584413,1.17063882517362,
-7.15586742123826));
#134423=CARTESIAN_POINT('Ctrl Pts',(-23.4718381460451,1.2647487847365,-7.16053380107808));
#134424=CARTESIAN_POINT('Ctrl Pts',(-23.4577523504494,1.33580899914792,
-7.16389923987488));
#134425=CARTESIAN_POINT('Ctrl Pts',(-23.4136240420131,1.49777028144667,
-7.17167745885749));
#134426=CARTESIAN_POINT('Ctrl Pts',(-23.3800166044622,1.58738566658417,
-7.17607379939565));
#134427=CARTESIAN_POINT('Ctrl Pts',(-23.3225703197009,1.70583732246154,
-7.18246826192759));
#134428=CARTESIAN_POINT('Ctrl Pts',(-23.3056601762985,1.73779458812649,
-7.18425462770703));
#134429=CARTESIAN_POINT('Ctrl Pts',(-23.273650854959,1.79346428721037,-7.18749456285743));
#134430=CARTESIAN_POINT('Ctrl Pts',(-23.2589964753055,1.8174137632315,-7.18893267095306));
#134431=CARTESIAN_POINT('Ctrl Pts',(-23.2249186609308,1.86983830929628,
-7.19218663482361));
#134432=CARTESIAN_POINT('Ctrl Pts',(-23.2051784341818,1.89808860119427,
-7.19401318830177));
#134433=CARTESIAN_POINT('Ctrl Pts',(-23.1404516046374,1.98441242923143,
-7.1998321920315));
#134434=CARTESIAN_POINT('Ctrl Pts',(-23.0922582773881,2.03994570306167,
-7.20393429709599));
#134435=CARTESIAN_POINT('Ctrl Pts',(-22.9748421830628,2.15719689916491,
-7.21334160530327));
#134436=CARTESIAN_POINT('Ctrl Pts',(-22.9036391416837,2.21654403609204,
-7.21866748139473));
#134437=CARTESIAN_POINT('Ctrl Pts',(-22.8064356547726,2.28375458395037,
-7.22515481445023));
#134438=CARTESIAN_POINT('Ctrl Pts',(-22.784961263876,2.29782421345522,-7.22654288378816));
#134439=CARTESIAN_POINT('Ctrl Pts',(-22.7493022659349,2.31993568488509,
-7.22876294875351));
#134440=CARTESIAN_POINT('Ctrl Pts',(-22.7353244335586,2.32829963880074,
-7.22961224423531));
#134441=CARTESIAN_POINT('Ctrl Pts',(-22.7031155255575,2.34688630745489,
-7.23152007551862));
#134442=CARTESIAN_POINT('Ctrl Pts',(-22.6848047304287,2.35696271424021,
-7.23257068044111));
#134443=CARTESIAN_POINT('Ctrl Pts',(-22.5692719180702,2.41751559109791,
-7.23902368287473));
#134444=CARTESIAN_POINT('Ctrl Pts',(-22.4671012880312,2.45789545795415,
-7.24398258813654));
#134445=CARTESIAN_POINT('Ctrl Pts',(-22.3121948561576,2.50076041021326,
-7.25145546034124));
#134446=CARTESIAN_POINT('Ctrl Pts',(-22.2622361565879,2.51194416002773,
-7.25385577103448));
#134447=CARTESIAN_POINT('Ctrl Pts',(-22.1715308460596,2.52756148926621,
-7.25828116903142));
#134448=CARTESIAN_POINT('Ctrl Pts',(-22.1309882027902,2.53289365621636,
-7.26028259981875));
#134449=CARTESIAN_POINT('Ctrl Pts',(-22.0619594124097,2.53919558030227,
-7.26375649074289));
#134450=CARTESIAN_POINT('Ctrl Pts',(-22.0335705239765,2.54099765733307,
-7.26520384315705));
#134451=CARTESIAN_POINT('Ctrl Pts',(-21.9734078333471,2.54314933590617,
-7.26831712319099));
#134452=CARTESIAN_POINT('Ctrl Pts',(-21.9416406956213,2.54330416067235,
-7.26998812350956));
#134453=CARTESIAN_POINT('Ctrl Pts',(-21.8468753336334,2.54084009038898,
-7.2750585036591));
#134454=CARTESIAN_POINT('Ctrl Pts',(-21.7840232013831,2.53534143395902,
-7.27853717554386));
#134455=CARTESIAN_POINT('Ctrl Pts',(-21.6243468563648,2.51145177189216,
-7.28761690548862));
#134456=CARTESIAN_POINT('Ctrl Pts',(-21.5286253330284,2.48760858816982,
-7.29330251109865));
#134457=CARTESIAN_POINT('Ctrl Pts',(-21.4045065326495,2.44374147697707,
-7.3006251062374));
#134458=CARTESIAN_POINT('Ctrl Pts',(-21.3735484677153,2.43166213524614,
-7.30244526827081));
#134459=CARTESIAN_POINT('Ctrl Pts',(-21.3270981830507,2.41178665936046,
-7.30514250636572));
#134460=CARTESIAN_POINT('Ctrl Pts',(-21.3113081209796,2.40471385140882,
-7.30605323168097));
#134461=CARTESIAN_POINT('Ctrl Pts',(-21.2790674065393,2.38961623386901,
-7.30789520428164));
#134462=CARTESIAN_POINT('Ctrl Pts',(-21.2626341129214,2.38156144162985,
-7.30882479588518));
#134463=CARTESIAN_POINT('Ctrl Pts',(-21.2105634331301,2.35487978438863,
-7.31175213004992));
#134464=CARTESIAN_POINT('Ctrl Pts',(-21.175507583218,2.33515076760792,-7.31369539834519));
#134465=CARTESIAN_POINT('Ctrl Pts',(-21.0961406510116,2.2863048176587,-7.31811707110993));
#134466=CARTESIAN_POINT('Ctrl Pts',(-21.0525001934093,2.25624249647932,
-7.32056604511031));
#134467=CARTESIAN_POINT('Ctrl Pts',(-21.0105083124886,2.22401157249359,
-7.32301699234766));
#134468=CARTESIAN_POINT('',(-23.4929995837554,0.998856457160122,-7.10475651497821));
#134469=CARTESIAN_POINT('Ctrl Pts',(-21.0105083871506,2.22401162980051,
-7.28231522554091));
#134470=CARTESIAN_POINT('Ctrl Pts',(-21.0154433030097,2.22779943054572,
-7.2820130562768));
#134471=CARTESIAN_POINT('Ctrl Pts',(-21.0204019059921,2.23155798536614,
-7.28170992437689));
#134472=CARTESIAN_POINT('Ctrl Pts',(-21.0524692318098,2.25556047488597,
-7.27975230871523));
#134473=CARTESIAN_POINT('Ctrl Pts',(-21.0802126029924,2.27493657437935,
-7.27807089094534));
#134474=CARTESIAN_POINT('Ctrl Pts',(-21.1320938352773,2.3086886945479,-7.27493466288154));
#134475=CARTESIAN_POINT('Ctrl Pts',(-21.1560305371592,2.32334763317577,
-7.27349072591619));
#134476=CARTESIAN_POINT('Ctrl Pts',(-21.2122677539476,2.35571236830967,
-7.27009975274404));
#134477=CARTESIAN_POINT('Ctrl Pts',(-21.2448281257554,2.37293016328562,
-7.26813730194881));
#134478=CARTESIAN_POINT('Ctrl Pts',(-21.3169976092341,2.40784818654129,
-7.26378785011317));
#134479=CARTESIAN_POINT('Ctrl Pts',(-21.3567999017545,2.42507606764693,
-7.26138903369756));
#134480=CARTESIAN_POINT('Ctrl Pts',(-21.5080480798264,2.48310656762016,
-7.25230379096701));
#134481=CARTESIAN_POINT('Ctrl Pts',(-21.6233510767689,2.51268840343621,
-7.24540369428604));
#134482=CARTESIAN_POINT('Ctrl Pts',(-21.7651606672024,2.53208449585394,
-7.23756759266639));
#134483=CARTESIAN_POINT('Ctrl Pts',(-21.7894961107612,2.53482478079956,
-7.23624690026639));
#134484=CARTESIAN_POINT('Ctrl Pts',(-21.8299994154273,2.53841167427614,
-7.23409950048903));
#134485=CARTESIAN_POINT('Ctrl Pts',(-21.8461326030543,2.53958508900774,
-7.23325789768662));
#134486=CARTESIAN_POINT('Ctrl Pts',(-21.8838441270495,2.54173239551484,
-7.23132362071633));
#134487=CARTESIAN_POINT('Ctrl Pts',(-21.9054294949286,2.54250735399395,
-7.23024045598921));
#134488=CARTESIAN_POINT('Ctrl Pts',(-21.9533154410427,2.54322044730049,
-7.22787733247796));
#134489=CARTESIAN_POINT('Ctrl Pts',(-21.9796126886395,2.54293990217794,
-7.22660616669071));
#134490=CARTESIAN_POINT('Ctrl Pts',(-22.0657856888371,2.53981647523319,
-7.22249340032146));
#134491=CARTESIAN_POINT('Ctrl Pts',(-22.1255053989186,2.53415758684263,
-7.21972515361034));
#134492=CARTESIAN_POINT('Ctrl Pts',(-22.2701556811391,2.5118918462487,-7.21294916558321));
#134493=CARTESIAN_POINT('Ctrl Pts',(-22.3543061852121,2.49159373334547,
-7.20893914798103));
#134494=CARTESIAN_POINT('Ctrl Pts',(-22.4695614278901,2.45331776208942,
-7.20302379902626));
#134495=CARTESIAN_POINT('Ctrl Pts',(-22.5024250381675,2.44114640207076,
-7.20128788444688));
#134496=CARTESIAN_POINT('Ctrl Pts',(-22.5607741855221,2.41724700131708,
-7.19810053903254));
#134497=CARTESIAN_POINT('Ctrl Pts',(-22.586408546388,2.40592254562723,-7.19666241153334));
#134498=CARTESIAN_POINT('Ctrl Pts',(-22.6436823226993,2.37873337814514,
-7.19335702924423));
#134499=CARTESIAN_POINT('Ctrl Pts',(-22.6751120434059,2.36246583866492,
-7.19147718478864));
#134500=CARTESIAN_POINT('Ctrl Pts',(-22.7414704559497,2.32517297960324,
-7.18736173738413));
#134501=CARTESIAN_POINT('Ctrl Pts',(-22.7761810526608,2.30381495724719,
-7.1851168749434));
#134502=CARTESIAN_POINT('Ctrl Pts',(-22.8905757391552,2.22702222184579,
-7.17741931534524));
#134503=CARTESIAN_POINT('Ctrl Pts',(-22.9658603965422,2.16545808079784,
-7.17182311867539));
#134504=CARTESIAN_POINT('Ctrl Pts',(-23.0635118593128,2.06890764052073,
-7.16410894451162));
#134505=CARTESIAN_POINT('Ctrl Pts',(-23.0910426054437,2.0394683168284,-7.16187627565383));
#134506=CARTESIAN_POINT('Ctrl Pts',(-23.1298573577239,1.99455976175702,
-7.15868013171908));
#134507=CARTESIAN_POINT('Ctrl Pts',(-23.1420560093701,1.97990562862154,
-7.15766803758976));
#134508=CARTESIAN_POINT('Ctrl Pts',(-23.1644838315487,1.95192442584678,
-7.15579861238001));
#134509=CARTESIAN_POINT('Ctrl Pts',(-23.174772511727,1.93864977178774,-7.15493795306817));
#134510=CARTESIAN_POINT('Ctrl Pts',(-23.2027698489291,1.90128277031755,
-7.15258029688543));
#134511=CARTESIAN_POINT('Ctrl Pts',(-23.2199988473526,1.8768386692303,-7.15111083575362));
#134512=CARTESIAN_POINT('Ctrl Pts',(-23.2601041473455,1.81627372022938,
-7.1476050035486));
#134513=CARTESIAN_POINT('Ctrl Pts',(-23.2822110673174,1.77967277852856,
-7.14559741607967));
#134514=CARTESIAN_POINT('Ctrl Pts',(-23.3587185524053,1.64022641179758,
-7.13819206927601));
#134515=CARTESIAN_POINT('Ctrl Pts',(-23.4029541298363,1.53226049804071,
-7.13289979707267));
#134516=CARTESIAN_POINT('Ctrl Pts',(-23.4439575791163,1.38743996206328,
-7.125551731529));
#134517=CARTESIAN_POINT('Ctrl Pts',(-23.4521782242363,1.35423064126585,
-7.1238535211426));
#134518=CARTESIAN_POINT('Ctrl Pts',(-23.4650622428798,1.29361002239718,
-7.12071564115976));
#134519=CARTESIAN_POINT('Ctrl Pts',(-23.4701013710537,1.26629333959326,
-7.11928801698951));
#134520=CARTESIAN_POINT('Ctrl Pts',(-23.478593183246,1.21209796685664,-7.11642423113787));
#134521=CARTESIAN_POINT('Ctrl Pts',(-23.4820804942635,1.18523474495591,
-7.11498966588192));
#134522=CARTESIAN_POINT('Ctrl Pts',(-23.4903223452944,1.10531999917952,
-7.11067568228148));
#134523=CARTESIAN_POINT('Ctrl Pts',(-23.4930390689691,1.05210288801396,
-7.10774127659502));
#134524=CARTESIAN_POINT('Ctrl Pts',(-23.4929995970599,0.998856170999325,
-7.10475651985954));
#134525=CARTESIAN_POINT('Ctrl Pts',(-23.4929995972711,0.998856455981027,
-7.10475653583426));
#134526=CARTESIAN_POINT('Ctrl Pts',(-23.4929235684559,0.896269736323447,
-7.09900601444055));
#134527=CARTESIAN_POINT('Ctrl Pts',(-23.4826173632919,0.793951174046108,
-7.09307389240344));
#134528=CARTESIAN_POINT('Ctrl Pts',(-23.4554216638391,0.659808150190311,
-7.08544914418858));
#134529=CARTESIAN_POINT('Ctrl Pts',(-23.447489592033,0.626435965649716,
-7.08356747181471));
#134530=CARTESIAN_POINT('Ctrl Pts',(-23.4338545668414,0.576527510145044,
-7.08080277447794));
#134531=CARTESIAN_POINT('Ctrl Pts',(-23.4289723050001,0.5597792430666,-7.07988358165846));
#134532=CARTESIAN_POINT('Ctrl Pts',(-23.4184651421447,0.525885426277317,
-7.07804590384003));
#134533=CARTESIAN_POINT('Ctrl Pts',(-23.4128214830959,0.508748672184849,
-7.07712845262034));
#134534=CARTESIAN_POINT('Ctrl Pts',(-23.3942266054438,0.4554509610844,-7.07430080697578));
#134535=CARTESIAN_POINT('Ctrl Pts',(-23.3802245111786,0.419670474931517,
-7.07243990595309));
#134536=CARTESIAN_POINT('Ctrl Pts',(-23.3247344473096,0.29212168199213,
-7.06582440446269));
#134537=CARTESIAN_POINT('Ctrl Pts',(-23.2756269513529,0.203946453300423,
-7.06127103180419));
#134538=CARTESIAN_POINT('Ctrl Pts',(-23.1947847243802,0.0872780304448506,
-7.0545992842203));
#134539=CARTESIAN_POINT('Ctrl Pts',(-23.1699431365536,0.0543315104024122,
-7.052635529525));
#134540=CARTESIAN_POINT('Ctrl Pts',(-23.1212172601452,-0.00517217496151634,
-7.0488955805939));
#134541=CARTESIAN_POINT('Ctrl Pts',(-23.0976733738544,-0.031972173152881,
-7.04713122248206));
#134542=CARTESIAN_POINT('Ctrl Pts',(-23.0540091024304,-0.0783312500188815,
-7.04391566112988));
#134543=CARTESIAN_POINT('Ctrl Pts',(-23.0342437025603,-0.0982030088020824,
-7.04247901301624));
#134544=CARTESIAN_POINT('Ctrl Pts',(-22.9887646089028,-0.141501763314325,
-7.03920886218204));
#134545=CARTESIAN_POINT('Ctrl Pts',(-22.9627783967539,-0.164619191730893,
-7.03736396896967));
#134546=CARTESIAN_POINT('Ctrl Pts',(-22.8759567370481,-0.236751334806526,
-7.03127076068956));
#134547=CARTESIAN_POINT('Ctrl Pts',(-22.8121812656029,-0.282026159689912,
-7.02689484245253));
#134548=CARTESIAN_POINT('Ctrl Pts',(-22.6885981218585,-0.356353052293743,
-7.01870584870337));
#134549=CARTESIAN_POINT('Ctrl Pts',(-22.6298048411199,-0.386753904916288,
-7.0149198752483));
#134550=CARTESIAN_POINT('Ctrl Pts',(-22.5440146711127,-0.424343430091305,
-7.00967619214999));
#134551=CARTESIAN_POINT('Ctrl Pts',(-22.5184945792665,-0.434720068827819,
-7.00815027324963));
#134552=CARTESIAN_POINT('Ctrl Pts',(-22.4718291636836,-0.452253724291736,
-7.00543646442907));
#134553=CARTESIAN_POINT('Ctrl Pts',(-22.4507802083443,-0.459645791147558,
-7.00423981184371));
#134554=CARTESIAN_POINT('Ctrl Pts',(-22.4142449426568,-0.471592971785797,
-7.00221832953674));
#134555=CARTESIAN_POINT('Ctrl Pts',(-22.3988356394484,-0.476365755844768,
-7.00138309921836));
#134556=CARTESIAN_POINT('Ctrl Pts',(-22.3607207743651,-0.487519248761599,
-6.99935827975823));
#134557=CARTESIAN_POINT('Ctrl Pts',(-22.3379391289771,-0.493622579457318,
-6.99818245163965));
#134558=CARTESIAN_POINT('Ctrl Pts',(-22.2089740258507,-0.525022989092951,
-6.99167488196766));
#134559=CARTESIAN_POINT('Ctrl Pts',(-22.1004735716382,-0.539520866665173,
-6.98674407773248));
#134560=CARTESIAN_POINT('Ctrl Pts',(-21.9429128893289,-0.543744164116973,
-6.97939961816967));
#134561=CARTESIAN_POINT('Ctrl Pts',(-21.8944492667416,-0.542760529498119,
-6.97711872041165));
#134562=CARTESIAN_POINT('Ctrl Pts',(-21.8066980210038,-0.536839038377313,
-6.97287877274052));
#134563=CARTESIAN_POINT('Ctrl Pts',(-21.767400942394,-0.532666620530167,
-6.97093984339362));
#134564=CARTESIAN_POINT('Ctrl Pts',(-21.7003350912236,-0.522929891555131,
-6.96753784741619));
#134565=CARTESIAN_POINT('Ctrl Pts',(-21.6724793484114,-0.518100846150755,
-6.96609707798743));
#134566=CARTESIAN_POINT('Ctrl Pts',(-21.6131465058929,-0.506127377859396,
-6.96296223021407));
#134567=CARTESIAN_POINT('Ctrl Pts',(-21.5817296271079,-0.498755046429045,
-6.96126188238585));
#134568=CARTESIAN_POINT('Ctrl Pts',(-21.4826261628817,-0.472195084465676,
-6.9557639991729));
#134569=CARTESIAN_POINT('Ctrl Pts',(-21.4160151938523,-0.449363720947438,
-6.95186191620282));
#134570=CARTESIAN_POINT('Ctrl Pts',(-21.2800805401054,-0.39212482982534,
-6.94353064191551));
#134571=CARTESIAN_POINT('Ctrl Pts',(-21.2113095914403,-0.356886132052856,
-6.93909812875738));
#134572=CARTESIAN_POINT('Ctrl Pts',(-21.1100450799699,-0.295008716368494,
-6.93243413491605));
#134573=CARTESIAN_POINT('Ctrl Pts',(-21.0755116954913,-0.271944376227107,
-6.93013619706407));
#134574=CARTESIAN_POINT('Ctrl Pts',(-21.0270350840932,-0.236658793809985,
-6.92691624399505));
#134575=CARTESIAN_POINT('Ctrl Pts',(-21.0123168573177,-0.225536450728647,
-6.92593950089538));
#134576=CARTESIAN_POINT('Ctrl Pts',(-20.9843119570395,-0.203573606993106,
-6.92408833559616));
#134577=CARTESIAN_POINT('Ctrl Pts',(-20.9709999790984,-0.192770641257813,
-6.9232121190002));
#134578=CARTESIAN_POINT('Ctrl Pts',(-20.9331534224597,-0.160996785684957,
-6.92072351297379));
#134579=CARTESIAN_POINT('Ctrl Pts',(-20.909092004255,-0.139474124473975,
-6.91914429441138));
#134580=CARTESIAN_POINT('Ctrl Pts',(-20.8077072639397,-0.0428929965425517,
-6.91241776664495));
#134581=CARTESIAN_POINT('Ctrl Pts',(-20.7376880684383,0.0393955660242851,
-6.90756134962266));
#134582=CARTESIAN_POINT('Ctrl Pts',(-20.6530010058874,0.163089637464466,
-6.90052454657455));
#134583=CARTESIAN_POINT('Ctrl Pts',(-20.6306265776347,0.198826577730289,
-6.898521096522));
#134584=CARTESIAN_POINT('Ctrl Pts',(-20.5918250272167,0.266844205188268,
-6.89471787182838));
#134585=CARTESIAN_POINT('Ctrl Pts',(-20.5750169378145,0.298873752970388,
-6.89293087809891));
#134586=CARTESIAN_POINT('Ctrl Pts',(-20.547316080813,0.356495366945819,
-6.88970547296704));
#134587=CARTESIAN_POINT('Ctrl Pts',(-20.5359606161303,0.38184719788406,
-6.88828301164002));
#134588=CARTESIAN_POINT('Ctrl Pts',(-20.5121629580809,0.43906928953469,
-6.88505922553819));
#134589=CARTESIAN_POINT('Ctrl Pts',(-20.5000842471488,0.471074015530362,
-6.88324720963607));
#134590=CARTESIAN_POINT('Ctrl Pts',(-20.4518269416484,0.61305446837943,
-6.8751647374586));
#134591=CARTESIAN_POINT('Ctrl Pts',(-20.4270307385083,0.726490167276728,
-6.86855659908311));
#134592=CARTESIAN_POINT('Ctrl Pts',(-20.4107297270828,0.884453665080072,
-6.85953431059122));
#134593=CARTESIAN_POINT('Ctrl Pts',(-20.4081041812435,0.927463828955015,
-6.85710049262177));
#134594=CARTESIAN_POINT('Ctrl Pts',(-20.4067076773825,1.00056636344053,
-6.85305303151891));
#134595=CARTESIAN_POINT('Ctrl Pts',(-20.4070112176528,1.03061597687359,
-6.85141498321165));
#134596=CARTESIAN_POINT('Ctrl Pts',(-20.4088527960233,1.0774398547753,-6.84892117341234));
#134597=CARTESIAN_POINT('Ctrl Pts',(-20.4097881696222,1.0942297131862,-6.84803886342712));
#134598=CARTESIAN_POINT('Ctrl Pts',(-20.4123662245766,1.12997337732766,
-6.84618996558625));
#134599=CARTESIAN_POINT('Ctrl Pts',(-20.4140852520832,1.1489182898307,-6.84522698511415));
#134600=CARTESIAN_POINT('Ctrl Pts',(-20.42050610887,1.20760122916372,-6.84228409368999));
#134601=CARTESIAN_POINT('Ctrl Pts',(-20.4264036946116,1.24719329182546,
-6.84035554010008));
#134602=CARTESIAN_POINT('Ctrl Pts',(-20.4519070219309,1.38215124775166,
-6.83385124108246));
#134603=CARTESIAN_POINT('Ctrl Pts',(-20.4789884718184,1.4758659320459,-6.82944225733426));
#134604=CARTESIAN_POINT('Ctrl Pts',(-20.5296893367747,1.60434242310546,
-6.82294545066961));
#134605=CARTESIAN_POINT('Ctrl Pts',(-20.5461572741502,1.6416677470014,-6.82100222148694));
#134606=CARTESIAN_POINT('Ctrl Pts',(-20.5796471676462,1.71009542190057,
-6.81729507665812));
#134607=CARTESIAN_POINT('Ctrl Pts',(-20.5962996928161,1.74134853143709,
-6.81554251962331));
#134608=CARTESIAN_POINT('Ctrl Pts',(-20.6280302337796,1.79625997677209,
-6.81233885406098));
#134609=CARTESIAN_POINT('Ctrl Pts',(-20.642706422861,1.82013254419814,-6.81090178551949));
#134610=CARTESIAN_POINT('Ctrl Pts',(-20.6771650920889,1.87290664683747,
-6.80761800174241));
#134611=CARTESIAN_POINT('Ctrl Pts',(-20.6972974748007,1.90156023183691,
-6.8057594227486));
#134612=CARTESIAN_POINT('Ctrl Pts',(-20.7687254420368,1.99620402690321,
-6.79935474250027));
#134613=CARTESIAN_POINT('Ctrl Pts',(-20.8243953407901,2.05869903584125,
-6.79465794669617));
#134614=CARTESIAN_POINT('Ctrl Pts',(-20.9247799203756,2.15447800779839,
-6.78676889289815));
#134615=CARTESIAN_POINT('Ctrl Pts',(-20.9667284900612,2.19040831542292,
-6.78361570988936));
#134616=CARTESIAN_POINT('Ctrl Pts',(-21.010508379234,2.22401162372414,-6.7805154429392));
#134617=CARTESIAN_POINT('Origin',(-21.9500000210213,0.999999999999992,-4.89578827641128));
#134618=CARTESIAN_POINT('',(-21.0105083954618,2.22401163617983,-6.28210099484077));
#134619=CARTESIAN_POINT('',(-21.0104995485061,2.22400480179726,-6.32268395191223));
#134620=CARTESIAN_POINT('',(-21.0105083758276,2.22401162110953,-4.89578827641128));
#134621=CARTESIAN_POINT('',(-23.4929994962299,0.998727401813637,-6.10421116902006));
#134622=CARTESIAN_POINT('Ctrl Pts',(-21.0105083954618,2.22401163617983,
-6.28210099484077));
#134623=CARTESIAN_POINT('Ctrl Pts',(-21.0399420576368,2.24660347951331,
-6.28033334307814));
#134624=CARTESIAN_POINT('Ctrl Pts',(-21.0701862087003,2.26813026764285,
-6.27853890030681));
#134625=CARTESIAN_POINT('Ctrl Pts',(-21.1272476034273,2.30571881745943,
-6.27516770049963));
#134626=CARTESIAN_POINT('Ctrl Pts',(-21.1538260232459,2.32209302687499,
-6.27360290129919));
#134627=CARTESIAN_POINT('Ctrl Pts',(-21.2058017969316,2.35197793063193,
-6.27054312625838));
#134628=CARTESIAN_POINT('Ctrl Pts',(-21.2311163498558,2.36560662365534,
-6.26905302826995));
#134629=CARTESIAN_POINT('Ctrl Pts',(-21.2951697405236,2.39781659414886,
-6.26527786714295));
#134630=CARTESIAN_POINT('Ctrl Pts',(-21.3343301025341,2.41550133710155,
-6.26296519001372));
#134631=CARTESIAN_POINT('Ctrl Pts',(-21.4710988065573,2.4705158514446,-6.25487663302854));
#134632=CARTESIAN_POINT('Ctrl Pts',(-21.5717263105529,2.49955619443129,
-6.24888457579755));
#134633=CARTESIAN_POINT('Ctrl Pts',(-21.7277180933228,2.52786285000555,
-6.23991047362025));
#134634=CARTESIAN_POINT('Ctrl Pts',(-21.7814083644928,2.53471553886673,
-6.2368815771936));
#134635=CARTESIAN_POINT('Ctrl Pts',(-21.8553177804522,2.54022244172986,
-6.23287967914589));
#134636=CARTESIAN_POINT('Ctrl Pts',(-21.8753128488886,2.5413214450698,-6.23181386516449));
#134637=CARTESIAN_POINT('Ctrl Pts',(-21.9121701837277,2.54262828845049,
-6.2298869175179));
#134638=CARTESIAN_POINT('Ctrl Pts',(-21.9290242886329,2.54294950002155,
-6.22902091033235));
#134639=CARTESIAN_POINT('Ctrl Pts',(-21.974782136117,2.54307165911276,-6.22670446443604));
#134640=CARTESIAN_POINT('Ctrl Pts',(-22.0036816037231,2.54233678673989,
-6.22527853767758));
#134641=CARTESIAN_POINT('Ctrl Pts',(-22.0729403217914,2.53862638826864,
-6.22191620035668));
#134642=CARTESIAN_POINT('Ctrl Pts',(-22.113236826147,2.53487442235251,-6.22000460833268));
#134643=CARTESIAN_POINT('Ctrl Pts',(-22.2764385706084,2.51317803463437,
-6.21229706939189));
#134644=CARTESIAN_POINT('Ctrl Pts',(-22.3971028428975,2.48201488658762,
-6.20663628045763));
#134645=CARTESIAN_POINT('Ctrl Pts',(-22.5425760708672,2.42503691862949,
-6.19894016248278));
#134646=CARTESIAN_POINT('Ctrl Pts',(-22.5720513687978,2.41241939267394,
-6.19733559635578));
#134647=CARTESIAN_POINT('Ctrl Pts',(-22.6271966893725,2.38675215540171,
-6.19423532974995));
#134648=CARTESIAN_POINT('Ctrl Pts',(-22.6529362929851,2.37388403002961,
-6.19274595625672));
#134649=CARTESIAN_POINT('Ctrl Pts',(-22.7150309651085,2.34063885617738,
-6.18904239299203));
#134650=CARTESIAN_POINT('Ctrl Pts',(-22.7509478063943,2.31949502682848,
-6.18680367436301));
#134651=CARTESIAN_POINT('Ctrl Pts',(-22.8300682175276,2.26849612803417,
-6.18164975339245));
#134652=CARTESIAN_POINT('Ctrl Pts',(-22.8726917097609,2.23783759138832,
-6.17871252205881));
#134653=CARTESIAN_POINT('Ctrl Pts',(-22.9970391372201,2.13839958269721,
-6.16969915852561));
#134654=CARTESIAN_POINT('Ctrl Pts',(-23.0732672897155,2.06325741091267,
-6.16352545379134));
#134655=CARTESIAN_POINT('Ctrl Pts',(-23.1547083221331,1.96435639115255,
-6.15656940289705));
#134656=CARTESIAN_POINT('Ctrl Pts',(-23.1679444396728,1.94758473008388,
-6.15542626544825));
#134657=CARTESIAN_POINT('Ctrl Pts',(-23.1902798871168,1.91804164419559,
-6.15348251238319));
#134658=CARTESIAN_POINT('Ctrl Pts',(-23.1995400452213,1.90539736460431,
-6.1526723881803));
#134659=CARTESIAN_POINT('Ctrl Pts',(-23.2217834688439,1.87403355879309,
-6.15071616183161));
#134660=CARTESIAN_POINT('Ctrl Pts',(-23.2345475457967,1.85516405463928,
-6.14958334449216));
#134661=CARTESIAN_POINT('Ctrl Pts',(-23.2624514573597,1.81187754770932,
-6.14706663325803));
#134662=CARTESIAN_POINT('Ctrl Pts',(-23.2773367856322,1.78730628113049,
-6.14569480397432));
#134663=CARTESIAN_POINT('Ctrl Pts',(-23.3278520552486,1.69841118107881,
-6.14088067068674));
#134664=CARTESIAN_POINT('Ctrl Pts',(-23.3595621120084,1.63197301865059,
-6.13754841931213));
#134665=CARTESIAN_POINT('Ctrl Pts',(-23.4156185653712,1.48908618307238,
-6.13049356446041));
#134666=CARTESIAN_POINT('Ctrl Pts',(-23.438989578096,1.4124944097765,-6.1267702769421));
#134667=CARTESIAN_POINT('Ctrl Pts',(-23.4631992388391,1.30345455377153,
-6.12131064098858));
#134668=CARTESIAN_POINT('Ctrl Pts',(-23.469121040962,1.2722640034517,-6.1197324987456));
#134669=CARTESIAN_POINT('Ctrl Pts',(-23.4782868704816,1.21427896280653,
-6.11675767833993));
#134670=CARTESIAN_POINT('Ctrl Pts',(-23.4817980370255,1.18753902847286,
-6.11536997386869));
#134671=CARTESIAN_POINT('Ctrl Pts',(-23.4872188284534,1.1357801535101,-6.11264969886424));
#134672=CARTESIAN_POINT('Ctrl Pts',(-23.4892224601812,1.11077950719954,
-6.1113204876626));
#134673=CARTESIAN_POINT('Ctrl Pts',(-23.492229676773,1.05674573773822,-6.10841408928787));
#134674=CARTESIAN_POINT('Ctrl Pts',(-23.4930244222693,1.0277112516658,-6.10683148327199));
#134675=CARTESIAN_POINT('Ctrl Pts',(-23.4929994504673,0.998673075206048,
-6.10522924338513));
#134676=CARTESIAN_POINT('',(-22.3485138628786,-0.490649428218508,-6.00000000000001));
#134677=CARTESIAN_POINT('Ctrl Pts',(-22.3485138628786,-0.490649428218505,
-6.00000000000001));
#134678=CARTESIAN_POINT('Ctrl Pts',(-22.4054645488374,-0.475424093389119,
-6.00304027996498));
#134679=CARTESIAN_POINT('Ctrl Pts',(-22.4615861511829,-0.456918922190118,
-6.00608055992995));
#134680=CARTESIAN_POINT('Ctrl Pts',(-22.5164905695608,-0.435248221882018,
-6.00912083989493));
#134681=CARTESIAN_POINT('Ctrl Pts',(-22.5713672765413,-0.413588459225288,
-6.01215958536762));
#134682=CARTESIAN_POINT('Ctrl Pts',(-22.6250275672966,-0.388766515308164,
-6.01519833084031));
#134683=CARTESIAN_POINT('Ctrl Pts',(-22.6771008615109,-0.360945762240122,
-6.01823707631301));
#134684=CARTESIAN_POINT('Ctrl Pts',(-22.7291610802877,-0.333131994874129,
-6.02127505876644));
#134685=CARTESIAN_POINT('Ctrl Pts',(-22.7796346657544,-0.302321142806013,
-6.02431304121987));
#134686=CARTESIAN_POINT('Ctrl Pts',(-22.8281749607985,-0.268722891394062,
-6.0273510236733));
#134687=CARTESIAN_POINT('Ctrl Pts',(-22.8767176954887,-0.235122951326502,
-6.0303891588164));
#134688=CARTESIAN_POINT('Ctrl Pts',(-22.9233265478032,-0.198735610807954,
-6.03342729395951));
#134689=CARTESIAN_POINT('Ctrl Pts',(-22.9676847033286,-0.159813298508449,
-6.03646542910262));
#134690=CARTESIAN_POINT('Ctrl Pts',(-23.0120584570753,-0.120877299462252,
-6.03950463258375));
#134691=CARTESIAN_POINT('Ctrl Pts',(-23.0541795776982,-0.0794048791799065,
-6.04254383606487));
#134692=CARTESIAN_POINT('Ctrl Pts',(-23.093766475409,-0.0356868724751493,
-6.045583039546));
#134693=CARTESIAN_POINT('Ctrl Pts',(-23.1334091763913,0.00809276087724915,
-6.04862652720969));
#134694=CARTESIAN_POINT('Ctrl Pts',(-23.1705101975796,0.0541239379441578,
-6.05167001487339));
#134695=CARTESIAN_POINT('Ctrl Pts',(-23.204827386285,0.102081694481424,
-6.05471350253708));
#134696=CARTESIAN_POINT('Ctrl Pts',(-23.2391709747928,0.150076344346653,
-6.05775933151939));
#134697=CARTESIAN_POINT('Ctrl Pts',(-23.2707262037194,0.200000116083609,
-6.06080516050171));
#134698=CARTESIAN_POINT('Ctrl Pts',(-23.2992951510333,0.25150039938155,
-6.06385098948403));
#134699=CARTESIAN_POINT('Ctrl Pts',(-23.3279184112935,0.303098590806417,
-6.06690260894732));
#134700=CARTESIAN_POINT('Ctrl Pts',(-23.353543839082,0.356278842196677,
-6.06995422841061));
#134701=CARTESIAN_POINT('Ctrl Pts',(-23.3760205576544,0.41066611407408,
-6.07300584787389));
#134702=CARTESIAN_POINT('Ctrl Pts',(-23.3862470624495,0.435411349676536,
-6.07439428012985));
#134703=CARTESIAN_POINT('Ctrl Pts',(-23.3958224323161,0.46040621178625,
-6.07578271238581));
#134704=CARTESIAN_POINT('Ctrl Pts',(-23.4047358843596,0.485614378197155,
-6.07717114464177));
#134705=CARTESIAN_POINT('Ctrl Pts',(-23.4262377242088,0.546423810324719,
-6.0805204472311));
#134706=CARTESIAN_POINT('Ctrl Pts',(-23.4439525213542,0.608667248297671,
-6.08386974982044));
#134707=CARTESIAN_POINT('Ctrl Pts',(-23.4577111099897,0.671889847457075,
-6.08721905240977));
#134708=CARTESIAN_POINT('Ctrl Pts',(-23.4713655900064,0.734634053254386,
-6.09054301146455));
#134709=CARTESIAN_POINT('Ctrl Pts',(-23.481123374027,0.798342409543584,
-6.09386697051933));
#134710=CARTESIAN_POINT('Ctrl Pts',(-23.4868657659852,0.862549347195262,
-6.09719092957411));
#134711=CARTESIAN_POINT('Ctrl Pts',(-23.4909084317617,0.907751275475867,
-6.09953100938943));
#134712=CARTESIAN_POINT('Ctrl Pts',(-23.4929619471197,0.953199867774789,
-6.10187108920474));
#134713=CARTESIAN_POINT('Ctrl Pts',(-23.4929994962299,0.998727401813637,
-6.10421116902006));
#134714=CARTESIAN_POINT('',(-21.5504160121885,-0.491448856702306,-6.00061430725121));
#134715=CARTESIAN_POINT('Origin',(-21.9500000210213,0.999999999999992,-6.00000000000001));
#134716=CARTESIAN_POINT('Ctrl Pts',(-21.5507399893082,-0.490449739869315,
-6.00122170731199));
#134717=CARTESIAN_POINT('Ctrl Pts',(-21.6610500159688,-0.519999468092027,
-6.00677097255486));
#134718=CARTESIAN_POINT('Ctrl Pts',(-21.7743077902558,-0.537214133001513,
-6.01190259476999));
#134719=CARTESIAN_POINT('Ctrl Pts',(-21.9322474019439,-0.543520758127318,
-6.01930552493555));
#134720=CARTESIAN_POINT('Ctrl Pts',(-21.9761115034942,-0.543401889099155,
-6.02138429714415));
#134721=CARTESIAN_POINT('Ctrl Pts',(-22.0571228967315,-0.539727697711485,
-6.02531493526066));
#134722=CARTESIAN_POINT('Ctrl Pts',(-22.0942610855388,-0.536692936399459,
-6.02715245989659));
#134723=CARTESIAN_POINT('Ctrl Pts',(-22.1594942207025,-0.528976779336596,
-6.0304619058166));
#134724=CARTESIAN_POINT('Ctrl Pts',(-22.1876379153144,-0.524856029833001,
-6.03191676485581));
#134725=CARTESIAN_POINT('Ctrl Pts',(-22.2496355964202,-0.514020403450957,
-6.03518764553848));
#134726=CARTESIAN_POINT('Ctrl Pts',(-22.2834099463349,-0.50694288099423,
-6.03701370772975));
#134727=CARTESIAN_POINT('Ctrl Pts',(-22.3882782086187,-0.481269335601699,
-6.04282601778578));
#134728=CARTESIAN_POINT('Ctrl Pts',(-22.4582939949709,-0.458726186211478,
-6.04691998350428));
#134729=CARTESIAN_POINT('Ctrl Pts',(-22.5893559603307,-0.405942603454932,
-6.05490457723179));
#134730=CARTESIAN_POINT('Ctrl Pts',(-22.6505403979752,-0.376478824792641,
-6.05877689367356));
#134731=CARTESIAN_POINT('Ctrl Pts',(-22.7338709781122,-0.329350822765226,
-6.06412398750824));
#134732=CARTESIAN_POINT('Ctrl Pts',(-22.7577783682896,-0.314960667081059,
-6.06566654975089));
#134733=CARTESIAN_POINT('Ctrl Pts',(-22.8002959396778,-0.287771390292826,
-6.06840930513845));
#134734=CARTESIAN_POINT('Ctrl Pts',(-22.8190404855472,-0.275196876042019,
-6.06961825102237));
#134735=CARTESIAN_POINT('Ctrl Pts',(-22.8509429893663,-0.252765218852784,
-6.07166646327611));
#134736=CARTESIAN_POINT('Ctrl Pts',(-22.8642302338089,-0.243101798573084,
-6.07251597341895));
#134737=CARTESIAN_POINT('Ctrl Pts',(-22.8936494233844,-0.220979149973743,
-6.07439005923984));
#134738=CARTESIAN_POINT('Ctrl Pts',(-22.9096931179497,-0.208409495667832,
-6.07540819278686));
#134739=CARTESIAN_POINT('Ctrl Pts',(-22.9831314129292,-0.148487828845703,
-6.08007342936211));
#134740=CARTESIAN_POINT('Ctrl Pts',(-23.0373059617777,-0.0973387028306494,
-6.08353226615008));
#134741=CARTESIAN_POINT('Ctrl Pts',(-23.1502278023002,0.0258849230818559,
-6.09128240976901));
#134742=CARTESIAN_POINT('Ctrl Pts',(-23.2065829199942,0.0997527170754831,
-6.09556125321762));
#134743=CARTESIAN_POINT('Ctrl Pts',(-23.2753571201417,0.2090489116262,-6.10183440883477));
#134744=CARTESIAN_POINT('Ctrl Pts',(-23.293652973816,0.240545219623791,
-6.10363421644827));
#134745=CARTESIAN_POINT('Ctrl Pts',(-23.3239863983212,0.297297376375765,
-6.10688135315738));
#134746=CARTESIAN_POINT('Ctrl Pts',(-23.336483743355,0.322288922384821,
-6.10831252467071));
#134747=CARTESIAN_POINT('Ctrl Pts',(-23.3628453486188,0.378790441542916,
-6.11155674323206));
#134748=CARTESIAN_POINT('Ctrl Pts',(-23.3763472268142,0.410452167354132,
-6.11338058526193));
#134749=CARTESIAN_POINT('Ctrl Pts',(-23.4145000719108,0.508922436110657,
-6.1190745475602));
#134750=CARTESIAN_POINT('Ctrl Pts',(-23.4355937249144,0.577002067434984,
-6.12304559436128));
#134751=CARTESIAN_POINT('Ctrl Pts',(-23.4736296145518,0.738508175634958,
-6.13244529422364));
#134752=CARTESIAN_POINT('Ctrl Pts',(-23.486808582738,0.832532780455595,
-6.13790701918962));
#134753=CARTESIAN_POINT('Ctrl Pts',(-23.4925200820875,0.953409077433793,
-6.14455887250051));
#134754=CARTESIAN_POINT('Ctrl Pts',(-23.493089727375,0.979673689909002,
-6.14598107634226));
#134755=CARTESIAN_POINT('Ctrl Pts',(-23.4929256542696,1.02228395308811,
-6.14823784741868));
#134756=CARTESIAN_POINT('Ctrl Pts',(-23.4926031013543,1.03862511078824,
-6.14909097477935));
#134757=CARTESIAN_POINT('Ctrl Pts',(-23.4912912630949,1.07543165259509,
-6.15098226069784));
#134758=CARTESIAN_POINT('Ctrl Pts',(-23.4901539825997,1.09588784344058,
-6.15201334818872));
#134759=CARTESIAN_POINT('Ctrl Pts',(-23.4839198812159,1.17835138725323,
-6.15610969450251));
#134760=CARTESIAN_POINT('Ctrl Pts',(-23.4754822318377,1.240051155664,-6.1590383024477));
#134761=CARTESIAN_POINT('Ctrl Pts',(-23.4408852249599,1.41395056175007,
-6.16728626316443));
#134762=CARTESIAN_POINT('Ctrl Pts',(-23.405873775418,1.5239508049406,-6.17252363801508));
#134763=CARTESIAN_POINT('Ctrl Pts',(-23.3450089343391,1.66028020901609,
-6.17980846545791));
#134764=CARTESIAN_POINT('Ctrl Pts',(-23.3300248175135,1.69105077579272,
-6.18150651637506));
#134765=CARTESIAN_POINT('Ctrl Pts',(-23.3009754905653,1.74598543158371,
-6.18465167366141));
#134766=CARTESIAN_POINT('Ctrl Pts',(-23.287252773586,1.77031417764042,-6.18608690057584));
#134767=CARTESIAN_POINT('Ctrl Pts',(-23.2543643062361,1.82509175063418,
-6.18942219110806));
#134768=CARTESIAN_POINT('Ctrl Pts',(-23.2347792649466,1.85526873488805,
-6.1913362310384));
#134769=CARTESIAN_POINT('Ctrl Pts',(-23.1600938155023,1.96198378283801,
-6.1983915769134));
#134770=CARTESIAN_POINT('Ctrl Pts',(-23.099066730903,2.03410928827497,-6.20373287736962));
#134771=CARTESIAN_POINT('Ctrl Pts',(-22.9788263056844,2.15234322845604,
-6.21333998477113));
#134772=CARTESIAN_POINT('Ctrl Pts',(-22.9221026636113,2.20058158039932,
-6.21757701323441));
#134773=CARTESIAN_POINT('Ctrl Pts',(-22.8440209512564,2.25780723714646,
-6.22285162256179));
#134774=CARTESIAN_POINT('Ctrl Pts',(-22.8256348519561,2.27067549443591,
-6.22405633446677));
#134775=CARTESIAN_POINT('Ctrl Pts',(-22.7935832655446,2.29208188377887,
-6.22608452755371));
#134776=CARTESIAN_POINT('Ctrl Pts',(-22.7800543441279,2.30081441448915,
-6.22691876824615));
#134777=CARTESIAN_POINT('Ctrl Pts',(-22.7466045939436,2.3216708294086,-6.22892982368272));
#134778=CARTESIAN_POINT('Ctrl Pts',(-22.7265415836033,2.333557623114,-6.2300933820803));
#134779=CARTESIAN_POINT('Ctrl Pts',(-22.680634511015,2.35936879660854,-6.23267772917099));
#134780=CARTESIAN_POINT('Ctrl Pts',(-22.6546468587024,2.3730197589747,-6.23408672358884));
#134781=CARTESIAN_POINT('Ctrl Pts',(-22.5598870564335,2.41939620322339,
-6.23908531612044));
#134782=CARTESIAN_POINT('Ctrl Pts',(-22.489103459848,2.44776240380153,-6.24256705516795));
#134783=CARTESIAN_POINT('Ctrl Pts',(-22.4114565320771,2.47239092282788,
-6.24635641860603));
#134784=CARTESIAN_POINT('Ctrl Pts',(-22.4063917444806,2.47396870242068,
-6.24660343356632));
#134785=CARTESIAN_POINT('Ctrl Pts',(-22.3377292321456,2.49497057530267,
-6.24995084027072));
#134786=CARTESIAN_POINT('Ctrl Pts',(-22.2729525430773,2.51028860883495,
-6.25309746792029));
#134787=CARTESIAN_POINT('Ctrl Pts',(-22.1755111153672,2.52677415703778,
-6.25795160199854));
#134788=CARTESIAN_POINT('Ctrl Pts',(-22.1434686229847,2.53116436088038,
-6.25956606450709));
#134789=CARTESIAN_POINT('Ctrl Pts',(-22.0830973930617,2.53751065570492,
-6.26265348577708));
#134790=CARTESIAN_POINT('Ctrl Pts',(-22.0548064789168,2.5396978275622,-6.26411889894446));
#134791=CARTESIAN_POINT('Ctrl Pts',(-21.9867470944211,2.54307506056329,
-6.26769407499894));
#134792=CARTESIAN_POINT('Ctrl Pts',(-21.9469629074188,2.54350944526434,
-6.2698249634293));
#134793=CARTESIAN_POINT('Ctrl Pts',(-21.8582828737924,2.54104916253855,
-6.2746659497019));
#134794=CARTESIAN_POINT('Ctrl Pts',(-21.8094524622411,2.53736476695281,
-6.27739396025025));
#134795=CARTESIAN_POINT('Ctrl Pts',(-21.6731460597477,2.52053146119447,
-6.28514267612558));
#134796=CARTESIAN_POINT('Ctrl Pts',(-21.5865046564124,2.50217678250399,
-6.29023233649642));
#134797=CARTESIAN_POINT('Ctrl Pts',(-21.4687029736605,2.46642646096579,
-6.29709151426721));
#134798=CARTESIAN_POINT('Ctrl Pts',(-21.4358412537486,2.45523003967735,
-6.29899642453891));
#134799=CARTESIAN_POINT('Ctrl Pts',(-21.3869755296177,2.43671857752933,
-6.30178902130684));
#134800=CARTESIAN_POINT('Ctrl Pts',(-21.3706740825828,2.43022318980088,
-6.30271370133179));
#134801=CARTESIAN_POINT('Ctrl Pts',(-21.337817154416,2.41647718771444,-6.30455827205078));
#134802=CARTESIAN_POINT('Ctrl Pts',(-21.3212712525374,2.40921101237725,
-6.30547722344926));
#134803=CARTESIAN_POINT('Ctrl Pts',(-21.2699277666166,2.38557900306318,
-6.30830857008338));
#134804=CARTESIAN_POINT('Ctrl Pts',(-21.2356102976186,2.36820142370269,
-6.3101716146859));
#134805=CARTESIAN_POINT('Ctrl Pts',(-21.1351312428264,2.3125085960954,-6.31563558238665));
#134806=CARTESIAN_POINT('Ctrl Pts',(-21.0711295876697,2.27054219549131,
-6.31913256746625));
#134807=CARTESIAN_POINT('Ctrl Pts',(-21.0104996389931,2.22400491509179,
-6.32268388509548));
#134808=CARTESIAN_POINT('Origin',(-21.9500000210213,0.999999999999992,-4.89578827641128));
#134809=CARTESIAN_POINT('Ctrl Pts',(-21.0104995251143,2.22400482768268,
-6.32268389176578));
#134810=CARTESIAN_POINT('Ctrl Pts',(-20.9562341136017,2.18235271988569,
-6.32586241547408));
#134811=CARTESIAN_POINT('Ctrl Pts',(-20.904801326001,2.13714005071609,-6.32907692812556));
#134812=CARTESIAN_POINT('Ctrl Pts',(-20.836886846209,2.0689265576077,-6.33377202520786));
#134813=CARTESIAN_POINT('Ctrl Pts',(-20.8177723087817,2.04865877321731,
-6.3351494024185));
#134814=CARTESIAN_POINT('Ctrl Pts',(-20.7803819362632,2.00679789242068,
-6.33796867069634));
#134815=CARTESIAN_POINT('Ctrl Pts',(-20.7621304569972,1.98519755889625,
-6.33941067971846));
#134816=CARTESIAN_POINT('Ctrl Pts',(-20.7241763881389,1.93769071429974,
-6.34256173010129));
#134817=CARTESIAN_POINT('Ctrl Pts',(-20.7046794530676,1.91163805099431,
-6.34427751992109));
#134818=CARTESIAN_POINT('Ctrl Pts',(-20.6422571075561,1.82248390314033,
-6.35011409126985));
#134819=CARTESIAN_POINT('Ctrl Pts',(-20.6031940448469,1.75682417900575,
-6.35436279536965));
#134820=CARTESIAN_POINT('Ctrl Pts',(-20.5269466097512,1.60391434667756,
-6.36404044954824));
#134821=CARTESIAN_POINT('Ctrl Pts',(-20.4926133630438,1.51557577547159,
-6.36949173509087));
#134822=CARTESIAN_POINT('Ctrl Pts',(-20.4593701503564,1.39944800184883,
-6.37613068745714));
#134823=CARTESIAN_POINT('Ctrl Pts',(-20.4527990439309,1.37406616908951,
-6.37754990006557));
#134824=CARTESIAN_POINT('Ctrl Pts',(-20.4431870672623,1.33261188094062,
-6.37980343335026));
#134825=CARTESIAN_POINT('Ctrl Pts',(-20.4397495176974,1.3166377024717,-6.38065619165817));
#134826=CARTESIAN_POINT('Ctrl Pts',(-20.4325568901538,1.2804261259711,-6.3825518739719));
#134827=CARTESIAN_POINT('Ctrl Pts',(-20.4289517763339,1.26016299182771,
-6.38358756660748));
#134828=CARTESIAN_POINT('Ctrl Pts',(-20.408399779469,1.12954571381993,-6.39013654082707));
#134829=CARTESIAN_POINT('Ctrl Pts',(-20.4030657857814,1.01769003896382,
-6.39518362391348));
#134830=CARTESIAN_POINT('Ctrl Pts',(-20.4129206373538,0.855827210789566,
-6.40272654629885));
#134831=CARTESIAN_POINT('Ctrl Pts',(-20.4184615460036,0.805607689584953,
-6.40509731095146));
#134832=CARTESIAN_POINT('Ctrl Pts',(-20.4328717565922,0.715721109269101,
-6.4094769056059));
#134833=CARTESIAN_POINT('Ctrl Pts',(-20.4408641619389,0.675960963588054,
-6.41146296055267));
#134834=CARTESIAN_POINT('Ctrl Pts',(-20.4571000342257,0.608969604186957,
-6.41491880669847));
#134835=CARTESIAN_POINT('Ctrl Pts',(-20.4645476519412,0.581566887249796,
-6.41636416598429));
#134836=CARTESIAN_POINT('Ctrl Pts',(-20.4819485838035,0.523881088261651,
-6.419481160704));
#134837=CARTESIAN_POINT('Ctrl Pts',(-20.4920926772242,0.493669843337177,
-6.42115813565528));
#134838=CARTESIAN_POINT('Ctrl Pts',(-20.5257524393385,0.402845995000081,
-6.4263410428713));
#134839=CARTESIAN_POINT('Ctrl Pts',(-20.5521672900069,0.343390251564348,
-6.4299329195472));
#134840=CARTESIAN_POINT('Ctrl Pts',(-20.6203403434113,0.212836742300793,
-6.43822622212054));
#134841=CARTESIAN_POINT('Ctrl Pts',(-20.6642042133427,0.143058002541596,
-6.44295830203225));
#134842=CARTESIAN_POINT('Ctrl Pts',(-20.7315494102603,0.0528222783889909,
-6.44928846053436));
#134843=CARTESIAN_POINT('Ctrl Pts',(-20.7503890387456,0.0290720038810077,
-6.45097557899787));
#134844=CARTESIAN_POINT('Ctrl Pts',(-20.7852712951851,-0.0123359045356564,
-6.45393509006294));
#134845=CARTESIAN_POINT('Ctrl Pts',(-20.8010469073053,-0.030205730246653,
-6.4552186523618));
#134846=CARTESIAN_POINT('Ctrl Pts',(-20.8282025812767,-0.0595662316240952,
-6.45732825101379));
#134847=CARTESIAN_POINT('Ctrl Pts',(-20.8393596816521,-0.0712554251554742,
-6.45816782161908));
#134848=CARTESIAN_POINT('Ctrl Pts',(-20.8662483195728,-0.0985545988870662,
-6.46012755899386));
#134849=CARTESIAN_POINT('Ctrl Pts',(-20.88213590301,-0.114004612038738,
-6.46123703413011));
#134850=CARTESIAN_POINT('Ctrl Pts',(-20.9598138514844,-0.186353685959237,
-6.46646524650204));
#134851=CARTESIAN_POINT('Ctrl Pts',(-21.0258530758953,-0.238490394082511,
-6.47033902180352));
#134852=CARTESIAN_POINT('Ctrl Pts',(-21.1484797236972,-0.320005204140976,
-6.47715631456662));
#134853=CARTESIAN_POINT('Ctrl Pts',(-21.2032481408839,-0.351743225870034,
-6.48008573476119));
#134854=CARTESIAN_POINT('Ctrl Pts',(-21.3012246596113,-0.400744078161206,
-6.48530548313974));
#134855=CARTESIAN_POINT('Ctrl Pts',(-21.3435506834406,-0.419581698746345,
-6.48755350984637));
#134856=CARTESIAN_POINT('Ctrl Pts',(-21.4137553273215,-0.447113623230408,
-6.49131200715453));
#134857=CARTESIAN_POINT('Ctrl Pts',(-21.441146992811,-0.45697105924249,
-6.49278530721232));
#134858=CARTESIAN_POINT('Ctrl Pts',(-21.4975619518885,-0.475488111564677,
-6.49584095296535));
#134859=CARTESIAN_POINT('Ctrl Pts',(-21.5265940810974,-0.484079721875075,
-6.49742464029722));
#134860=CARTESIAN_POINT('Ctrl Pts',(-21.6096220131408,-0.506015952451806,
-6.50199026825619));
#134861=CARTESIAN_POINT('Ctrl Pts',(-21.6641091384797,-0.517302451331485,
-6.50503113072352));
#134862=CARTESIAN_POINT('Ctrl Pts',(-21.812480326198,-0.539759817998222,
-6.51340318009745));
#134863=CARTESIAN_POINT('Ctrl Pts',(-21.9069774850213,-0.545289479571833,
-6.5188429419793));
#134864=CARTESIAN_POINT('Ctrl Pts',(-22.033347344027,-0.541079278017493,
-6.52596573887694));
#134865=CARTESIAN_POINT('Ctrl Pts',(-22.0652763800405,-0.539020354314514,
-6.52775069597113));
#134866=CARTESIAN_POINT('Ctrl Pts',(-22.1217359591999,-0.533612498204303,
-6.53085747415398));
#134867=CARTESIAN_POINT('Ctrl Pts',(-22.1462934541628,-0.530663105383828,
-6.5321919993967));
#134868=CARTESIAN_POINT('Ctrl Pts',(-22.1868194492482,-0.524804415545166,
-6.53435520691601));
#134869=CARTESIAN_POINT('Ctrl Pts',(-22.2028307423267,-0.52223146657294,
-6.53519924511303));
#134870=CARTESIAN_POINT('Ctrl Pts',(-22.2395951150924,-0.515727427956221,
-6.53711169458104));
#134871=CARTESIAN_POINT('Ctrl Pts',(-22.2603130945794,-0.511621921228222,
-6.53817165515519));
#134872=CARTESIAN_POINT('Ctrl Pts',(-22.3713839177443,-0.487231968747643,
-6.54378835514993));
#134873=CARTESIAN_POINT('Ctrl Pts',(-22.4598635700684,-0.459268836868039,
-6.5480350907299));
#134874=CARTESIAN_POINT('Ctrl Pts',(-22.6001469429997,-0.400603907158095,
-6.55507815490046));
#134875=CARTESIAN_POINT('Ctrl Pts',(-22.6536139325846,-0.374521509609291,
-6.55784135482481));
#134876=CARTESIAN_POINT('Ctrl Pts',(-22.7444188811032,-0.323535381443718,
-6.56281563063614));
#134877=CARTESIAN_POINT('Ctrl Pts',(-22.7824246651095,-0.299967705704365,
-6.56499076557906));
#134878=CARTESIAN_POINT('Ctrl Pts',(-22.8432256142893,-0.258503891876072,
-6.5686640702641));
#134879=CARTESIAN_POINT('Ctrl Pts',(-22.8666359666912,-0.241556447839582,
-6.57012876868565));
#134880=CARTESIAN_POINT('Ctrl Pts',(-22.9138325744578,-0.205326702411308,
-6.57319460310958));
#134881=CARTESIAN_POINT('Ctrl Pts',(-22.9375483131362,-0.185973798882371,
-6.57479801190376));
#134882=CARTESIAN_POINT('Ctrl Pts',(-23.004930141621,-0.127564667818754,
-6.57954616177047));
#134883=CARTESIAN_POINT('Ctrl Pts',(-23.0469641398496,-0.086714456729049,
-6.58275836341238));
#134884=CARTESIAN_POINT('Ctrl Pts',(-23.1569796139188,0.0331046437758653,
-6.59185970446722));
#134885=CARTESIAN_POINT('Ctrl Pts',(-23.2194426880718,0.116710483508204,
-6.59788077953576));
#134886=CARTESIAN_POINT('Ctrl Pts',(-23.2912070633835,0.236283472400158,
-6.60566010455058));
#134887=CARTESIAN_POINT('Ctrl Pts',(-23.308356659545,0.267219804178711,
-6.60760322519845));
#134888=CARTESIAN_POINT('Ctrl Pts',(-23.3324356887674,0.314411950420515,
-6.61043673716491));
#134889=CARTESIAN_POINT('Ctrl Pts',(-23.3401734202136,0.330240840590128,
-6.6113658409607));
#134890=CARTESIAN_POINT('Ctrl Pts',(-23.3552233444543,0.362413282298291,
-6.6132065810141));
#134891=CARTESIAN_POINT('Ctrl Pts',(-23.3625255688187,0.378758466336531,
-6.61411765569486));
#134892=CARTESIAN_POINT('Ctrl Pts',(-23.3841632059582,0.429547060338007,
-6.61688541096149));
#134893=CARTESIAN_POINT('Ctrl Pts',(-23.3975359418104,0.464387549600414,
-6.61869588756311));
#134894=CARTESIAN_POINT('Ctrl Pts',(-23.4298625914804,0.558697394457863,
-6.62344517255297));
#134895=CARTESIAN_POINT('Ctrl Pts',(-23.4464946628616,0.618889023904732,
-6.62632150302345));
#134896=CARTESIAN_POINT('Ctrl Pts',(-23.4766331346268,0.761018215989604,
-6.63304958114686));
#134897=CARTESIAN_POINT('Ctrl Pts',(-23.487265281678,0.843362629562132,
-6.63690547217981));
#134898=CARTESIAN_POINT('Ctrl Pts',(-23.4929082668566,0.961142564865192,
-6.64264947334773));
#134899=CARTESIAN_POINT('Ctrl Pts',(-23.4933926753148,0.996172631423811,
-6.64438499317861));
#134900=CARTESIAN_POINT('Ctrl Pts',(-23.4921176458459,1.05924199535909,
-6.64757409183285));
#134901=CARTESIAN_POINT('Ctrl Pts',(-23.4907853367835,1.08727465647435,
-6.64901444994649));
#134902=CARTESIAN_POINT('Ctrl Pts',(-23.4860372889687,1.15066291194352,
-6.65232896858211));
#134903=CARTESIAN_POINT('Ctrl Pts',(-23.4821637489637,1.18596734259516,
-6.6542159044333));
#134904=CARTESIAN_POINT('Ctrl Pts',(-23.4712090913378,1.26162638613013,
-6.65835012692968));
#134905=CARTESIAN_POINT('Ctrl Pts',(-23.463731816284,1.30189586599952,-6.66060684148032));
#134906=CARTESIAN_POINT('Ctrl Pts',(-23.4328736456791,1.43773153290873,
-6.66839145727455));
#134907=CARTESIAN_POINT('Ctrl Pts',(-23.4019655431347,1.53133589721564,
-6.67406668466317));
#134908=CARTESIAN_POINT('Ctrl Pts',(-23.3466214656947,1.65713401311009,
-6.68177779194508));
#134909=CARTESIAN_POINT('Ctrl Pts',(-23.3295278391368,1.69230047404541,
-6.68394064536241));
#134910=CARTESIAN_POINT('Ctrl Pts',(-23.3022236472745,1.74343573844717,
-6.68705933762911));
#134911=CARTESIAN_POINT('Ctrl Pts',(-23.2930257710599,1.7599258723455,-6.68806077676556));
#134912=CARTESIAN_POINT('Ctrl Pts',(-23.2750108856074,1.79087406184402,
-6.68992616830943));
#134913=CARTESIAN_POINT('Ctrl Pts',(-23.2662544151352,1.80536324413174,
-6.69079293623079));
#134914=CARTESIAN_POINT('Ctrl Pts',(-23.2409432436152,1.84572932969834,
-6.69319651652667));
#134915=CARTESIAN_POINT('Ctrl Pts',(-23.223850985873,1.871261403476,-6.69470390459601));
#134916=CARTESIAN_POINT('Ctrl Pts',(-23.1800957449363,1.93257890810397,
-6.69833351932767));
#134917=CARTESIAN_POINT('Ctrl Pts',(-23.1526208887644,1.96775115043998,
-6.70042416658543));
#134918=CARTESIAN_POINT('Ctrl Pts',(-23.0466673251364,2.09189542188605,
-6.70801287965762));
#134919=CARTESIAN_POINT('Ctrl Pts',(-22.9595373433578,2.17292280288611,
-6.71342011846344));
#134920=CARTESIAN_POINT('Ctrl Pts',(-22.8378521767939,2.26238657448279,
-6.72083474224028));
#134921=CARTESIAN_POINT('Ctrl Pts',(-22.8111180778296,2.28077196420455,
-6.72245361893247));
#134922=CARTESIAN_POINT('Ctrl Pts',(-22.7600259350867,2.31358557905283,
-6.72554074265786));
#134923=CARTESIAN_POINT('Ctrl Pts',(-22.7358116511044,2.32821271073992,
-6.72700110516213));
#134924=CARTESIAN_POINT('Ctrl Pts',(-22.6770094243654,2.36156242814138,
-6.73054636689619));
#134925=CARTESIAN_POINT('Ctrl Pts',(-22.6420821221952,2.37964377137921,
-6.7326515817394));
#134926=CARTESIAN_POINT('Ctrl Pts',(-22.5630159106784,2.41681678509703,
-6.73741613417258));
#134927=CARTESIAN_POINT('Ctrl Pts',(-22.5185986794014,2.43521892210959,
-6.74009239767715));
#134928=CARTESIAN_POINT('Ctrl Pts',(-22.3926152074019,2.48064685103347,
-6.7476444945669));
#134929=CARTESIAN_POINT('Ctrl Pts',(-22.3095438413971,2.50298080889107,
-6.75258775007764));
#134930=CARTESIAN_POINT('Ctrl Pts',(-22.1877083790675,2.52505201268467,
-6.75951568622415));
#134931=CARTESIAN_POINT('Ctrl Pts',(-22.1501307279146,2.53043685570049,
-6.76160781875572));
#134932=CARTESIAN_POINT('Ctrl Pts',(-22.0944990680934,2.53632441820255,
-6.76460540963081));
#134933=CARTESIAN_POINT('Ctrl Pts',(-22.0765749744832,2.53790491596644,
-6.76555602527367));
#134934=CARTESIAN_POINT('Ctrl Pts',(-22.041131350066,2.5404063387539,-6.76740053378691));
#134935=CARTESIAN_POINT('Ctrl Pts',(-22.0236157812493,2.54134271564379,
-6.76829494186236));
#134936=CARTESIAN_POINT('Ctrl Pts',(-21.9712829415989,2.5432462528985,-6.77092580964335));
#134937=CARTESIAN_POINT('Ctrl Pts',(-21.9364433604481,2.54333355593785,
-6.77262268627803));
#134938=CARTESIAN_POINT('Ctrl Pts',(-21.7931234648943,2.53883843510636,
-6.77948017284892));
#134939=CARTESIAN_POINT('Ctrl Pts',(-21.6852768798642,2.52399407466373,
-6.78437055207333));
#134940=CARTESIAN_POINT('Ctrl Pts',(-21.5254125865281,2.4844938621063,-6.79212364309885));
#134941=CARTESIAN_POINT('Ctrl Pts',(-21.471726072942,2.46807692340225,-6.79481389497106));
#134942=CARTESIAN_POINT('Ctrl Pts',(-21.3905822328316,2.43833943454232,
-6.79909201940464));
#134943=CARTESIAN_POINT('Ctrl Pts',(-21.3624244324847,2.42706810112698,
-6.80061711419488));
#134944=CARTESIAN_POINT('Ctrl Pts',(-21.3079700030568,2.40338551053759,
-6.80365574010498));
#134945=CARTESIAN_POINT('Ctrl Pts',(-21.2816558843548,2.39104615530282,
-6.80516647060912));
#134946=CARTESIAN_POINT('Ctrl Pts',(-21.2234565369133,2.36172232622214,
-6.80860841085151));
#134947=CARTESIAN_POINT('Ctrl Pts',(-21.1917884061643,2.34434668504245,
-6.81055170629451));
#134948=CARTESIAN_POINT('Ctrl Pts',(-21.108714593042,2.29489629144899,-6.81583981531629));
#134949=CARTESIAN_POINT('Ctrl Pts',(-21.0585416696014,2.26088010595229,
-6.81923971945315));
#134950=CARTESIAN_POINT('Ctrl Pts',(-21.010500834247,2.22400583252304,-6.82267576524316));
#134951=CARTESIAN_POINT('Ctrl Pts',(-21.010508379234,2.22401162372414,-6.7805154429392));
#134952=CARTESIAN_POINT('Ctrl Pts',(-21.0158319840829,2.22809776323681,
-6.78013845257946));
#134953=CARTESIAN_POINT('Ctrl Pts',(-21.0211826687174,2.23214949563438,
-6.779762270056));
#134954=CARTESIAN_POINT('Ctrl Pts',(-21.0479546426187,2.25214866918077,
-6.77789414648241));
#134955=CARTESIAN_POINT('Ctrl Pts',(-21.069761413228,2.2675733773478,-6.77641700861394));
#134956=CARTESIAN_POINT('Ctrl Pts',(-21.1101024866793,2.29456468137134,
-6.77377829641301));
#134957=CARTESIAN_POINT('Ctrl Pts',(-21.1285030699195,2.30631865728353,
-6.77260864865622));
#134958=CARTESIAN_POINT('Ctrl Pts',(-21.1609438262069,2.32608457938309,
-6.77061298461235));
#134959=CARTESIAN_POINT('Ctrl Pts',(-21.1748701643254,2.33427273249087,
-6.76977756093891));
#134960=CARTESIAN_POINT('Ctrl Pts',(-21.2099411322835,2.35415861960067,
-6.76772428237199));
#134961=CARTESIAN_POINT('Ctrl Pts',(-21.231236115858,2.36558093497895,-6.76652142220933));
#134962=CARTESIAN_POINT('Ctrl Pts',(-21.3591082537511,2.43034926128059,
-6.7595058326914));
#134963=CARTESIAN_POINT('Ctrl Pts',(-21.4713137061134,2.47170531252301,
-6.75416210594382));
#134964=CARTESIAN_POINT('Ctrl Pts',(-21.6293616921906,2.50994187462362,
-6.74654261423925));
#134965=CARTESIAN_POINT('Ctrl Pts',(-21.6719644205224,2.51836403026559,
-6.74448354629973));
#134966=CARTESIAN_POINT('Ctrl Pts',(-21.7512869548835,2.53059475126771,
-6.74059197164442));
#134967=CARTESIAN_POINT('Ctrl Pts',(-21.7878975289414,2.53490380989219,
-6.73877361598536));
#134968=CARTESIAN_POINT('Ctrl Pts',(-21.8525981064449,2.54017840620371,
-6.73550244069011));
#134969=CARTESIAN_POINT('Ctrl Pts',(-21.8806262774467,2.54169511006505,
-6.73406654873934));
#134970=CARTESIAN_POINT('Ctrl Pts',(-21.9424740070872,2.54335195946797,
-6.73085074675524));
#134971=CARTESIAN_POINT('Ctrl Pts',(-21.9762876254071,2.54314634694285,
-6.72906136890564));
#134972=CARTESIAN_POINT('Ctrl Pts',(-22.1286348797819,2.53721130201981,
-6.72085287407357));
#134973=CARTESIAN_POINT('Ctrl Pts',(-22.2462637612988,2.51893051234446,
-6.71407324563384));
#134974=CARTESIAN_POINT('Ctrl Pts',(-22.4011572741826,2.4761690198959,-6.70494802028667));
#134975=CARTESIAN_POINT('Ctrl Pts',(-22.4412254382283,2.46332351396336,
-6.70257354827352));
#134976=CARTESIAN_POINT('Ctrl Pts',(-22.508510626299,2.43867676985224,-6.69860984269868));
#134977=CARTESIAN_POINT('Ctrl Pts',(-22.5360042181797,2.42769892636964,
-6.69699735988813));
#134978=CARTESIAN_POINT('Ctrl Pts',(-22.5785388779167,2.4092794372668,-6.69453185836545));
#134979=CARTESIAN_POINT('Ctrl Pts',(-22.5938028425612,2.40237214751335,
-6.69365326401092));
#134980=CARTESIAN_POINT('Ctrl Pts',(-22.6262850837856,2.38703097935296,
-6.69180079736924));
#134981=CARTESIAN_POINT('Ctrl Pts',(-22.6434642433958,2.37852234693594,
-6.69083088443239));
#134982=CARTESIAN_POINT('Ctrl Pts',(-22.696841661751,2.35083469734678,-6.68783513167605));
#134983=CARTESIAN_POINT('Ctrl Pts',(-22.7324390925866,2.33053234822254,
-6.68586331655349));
#134984=CARTESIAN_POINT('Ctrl Pts',(-22.8388756668371,2.26407733948411,
-6.6799278788393));
#134985=CARTESIAN_POINT('Ctrl Pts',(-22.9067659995775,2.21350364864761,
-6.67607848618741));
#134986=CARTESIAN_POINT('Ctrl Pts',(-23.0190125075856,2.11458458275668,
-6.66908665964202));
#134987=CARTESIAN_POINT('Ctrl Pts',(-23.0650746359817,2.06850088429555,
-6.66599363517545));
#134988=CARTESIAN_POINT('Ctrl Pts',(-23.1287298590071,1.99620320124634,
-6.66124424824113));
#134989=CARTESIAN_POINT('Ctrl Pts',(-23.1486552774172,1.97213695556005,
-6.6596791010701));
#134990=CARTESIAN_POINT('Ctrl Pts',(-23.1853751846258,1.92493949450979,
-6.6566289499626));
#134991=CARTESIAN_POINT('Ctrl Pts',(-23.2022843990128,1.9019138338186,-6.65514918052333));
#134992=CARTESIAN_POINT('Ctrl Pts',(-23.2425644188,1.84374550446447,-6.6514258184822));
#134993=CARTESIAN_POINT('Ctrl Pts',(-23.2651501614679,1.80808965011639,
-6.64915593455419));
#134994=CARTESIAN_POINT('Ctrl Pts',(-23.3430156744391,1.67323548699643,
-6.64061895435643));
#134995=CARTESIAN_POINT('Ctrl Pts',(-23.3887578541548,1.56895524816671,
-6.63407810995863));
#134996=CARTESIAN_POINT('Ctrl Pts',(-23.4328202632318,1.42808318778802,
-6.62574372398752));
#134997=CARTESIAN_POINT('Ctrl Pts',(-23.4419161280397,1.39521843421883,
-6.62383579116251));
#134998=CARTESIAN_POINT('Ctrl Pts',(-23.4559719691841,1.33699181962598,
-6.6205465618877));
#134999=CARTESIAN_POINT('Ctrl Pts',(-23.4613977951412,1.31175616257833,
-6.61915051412952));
#135000=CARTESIAN_POINT('Ctrl Pts',(-23.4691843926443,1.27053356069065,
-6.61693023044573));
#135001=CARTESIAN_POINT('Ctrl Pts',(-23.4719314972308,1.25462564032951,
-6.61608815137605));
#135002=CARTESIAN_POINT('Ctrl Pts',(-23.4776218601947,1.21828113336301,
-6.61419977605289));
#135003=CARTESIAN_POINT('Ctrl Pts',(-23.4804055428535,1.19782354118241,
-6.61316116608744));
#135004=CARTESIAN_POINT('Ctrl Pts',(-23.4896298994907,1.11808486546197,
-6.60918679118317));
#135005=CARTESIAN_POINT('Ctrl Pts',(-23.4930433496661,1.05850239208585,
-6.60637398081075));
#135006=CARTESIAN_POINT('Ctrl Pts',(-23.4929123977605,0.879980588466109,
-6.59805811834505));
#135007=CARTESIAN_POINT('Ctrl Pts',(-23.4790861453881,0.761508781866254,
-6.59265560430452));
#135008=CARTESIAN_POINT('Ctrl Pts',(-23.4440436444851,0.612930062110029,
-6.58519421624484));
#135009=CARTESIAN_POINT('Ctrl Pts',(-23.4352147740766,0.58032581523435,
-6.58351569085597));
#135010=CARTESIAN_POINT('Ctrl Pts',(-23.4171075627419,0.521218975455224,
-6.58038309620043));
#135011=CARTESIAN_POINT('Ctrl Pts',(-23.4081619541454,0.494629386536749,
-6.57893981051724));
#135012=CARTESIAN_POINT('Ctrl Pts',(-23.3857994507276,0.433707849286491,
-6.57554803580583));
#135013=CARTESIAN_POINT('Ctrl Pts',(-23.3718676369664,0.399584314033827,
-6.57358404660376));
#135014=CARTESIAN_POINT('Ctrl Pts',(-23.3388913280474,0.32641670775893,
-6.56922966389112));
#135015=CARTESIAN_POINT('Ctrl Pts',(-23.3193928864519,0.28761225208465,
-6.56682737888396));
#135016=CARTESIAN_POINT('Ctrl Pts',(-23.2402869771439,0.145462469034467,
-6.55770283807279));
#135017=CARTESIAN_POINT('Ctrl Pts',(-23.1704028363531,0.0483220371332482,
-6.55076448196625));
#135018=CARTESIAN_POINT('Ctrl Pts',(-23.0737893992558,-0.0576044878973603,
-6.54292216097589));
#135019=CARTESIAN_POINT('Ctrl Pts',(-23.0571329308987,-0.0750286779057241,
-6.54162328574241));
#135020=CARTESIAN_POINT('Ctrl Pts',(-23.028646468382,-0.103463437826083,
-6.53949900737956));
#135021=CARTESIAN_POINT('Ctrl Pts',(-23.0170404137433,-0.114690349423836,
-6.53865948264827));
#135022=CARTESIAN_POINT('Ctrl Pts',(-22.989310460399,-0.140684296004001,
-6.53671437571113));
#135023=CARTESIAN_POINT('Ctrl Pts',(-22.9730454101688,-0.155294366914331,
-6.53561888994776));
#135024=CARTESIAN_POINT('Ctrl Pts',(-22.9361953473105,-0.18700614455315,
-6.53322219475524));
#135025=CARTESIAN_POINT('Ctrl Pts',(-22.9154647302448,-0.203928078952855,
-6.53193021308359));
#135026=CARTESIAN_POINT('Ctrl Pts',(-22.8451633437883,-0.258329209796937,
-6.52769522621964));
#135027=CARTESIAN_POINT('Ctrl Pts',(-22.7937690425955,-0.293353850330553,
-6.52483012745152));
#135028=CARTESIAN_POINT('Ctrl Pts',(-22.6688317874341,-0.367872169940582,
-6.51809418198171));
#135029=CARTESIAN_POINT('Ctrl Pts',(-22.5939250372128,-0.404689552146031,
-6.51421928011043));
#135030=CARTESIAN_POINT('Ctrl Pts',(-22.4838396276065,-0.448133563824942,
-6.50845448975972));
#135031=CARTESIAN_POINT('Ctrl Pts',(-22.4508360134639,-0.459876238515879,
-6.50671921363529));
#135032=CARTESIAN_POINT('Ctrl Pts',(-22.3907525256212,-0.478976595796365,
-6.5035321224017));
#135033=CARTESIAN_POINT('Ctrl Pts',(-22.3638169944941,-0.486738015358892,
-6.50209356883858));
#135034=CARTESIAN_POINT('Ctrl Pts',(-22.3024003776073,-0.502636772834646,
-6.49878590246613));
#135035=CARTESIAN_POINT('Ctrl Pts',(-22.2678212487443,-0.510328670147802,
-6.49690414862591));
#135036=CARTESIAN_POINT('Ctrl Pts',(-22.1929004767861,-0.524307426316777,
-6.49278341043077));
#135037=CARTESIAN_POINT('Ctrl Pts',(-22.1525123664644,-0.530196776520286,
-6.4905351174371));
#135038=CARTESIAN_POINT('Ctrl Pts',(-22.0150094238882,-0.544708068951087,
-6.48281006598786));
#135039=CARTESIAN_POINT('Ctrl Pts',(-21.9173332026759,-0.545729844303109,
-6.47718870666442));
#135040=CARTESIAN_POINT('Ctrl Pts',(-21.7805028360202,-0.534179947045099,
-6.46947870034317));
#135041=CARTESIAN_POINT('Ctrl Pts',(-21.7409314524311,-0.529290074618025,
-6.46727129671209));
#135042=CARTESIAN_POINT('Ctrl Pts',(-21.6828321060616,-0.519813011305401,
-6.46410260838279));
#135043=CARTESIAN_POINT('Ctrl Pts',(-21.6641298431269,-0.516406472774023,
-6.46309385846568));
#135044=CARTESIAN_POINT('Ctrl Pts',(-21.6289448336819,-0.509323542847642,
-6.46122336014601));
#135045=CARTESIAN_POINT('Ctrl Pts',(-21.6124509880453,-0.50572064195062,
-6.46035850839637));
#135046=CARTESIAN_POINT('Ctrl Pts',(-21.5665004722398,-0.494890250556752,
-6.45797549455699));
#135047=CARTESIAN_POINT('Ctrl Pts',(-21.537191549784,-0.487063594733397,
-6.45648575672324));
#135048=CARTESIAN_POINT('Ctrl Pts',(-21.4662484252342,-0.46585955517807,
-6.45291414954621));
#135049=CARTESIAN_POINT('Ctrl Pts',(-21.4249150449788,-0.451566714662723,
-6.45086240355508));
#135050=CARTESIAN_POINT('Ctrl Pts',(-21.2786382340742,-0.393917821786189,
-6.44354382177873));
#135051=CARTESIAN_POINT('Ctrl Pts',(-21.1779548297279,-0.34077544946403,
-6.43836818824263));
#135052=CARTESIAN_POINT('Ctrl Pts',(-21.0554792722513,-0.257724145329528,
-6.43114710654988));
#135053=CARTESIAN_POINT('Ctrl Pts',(-21.0276052634691,-0.237426803901148,
-6.42943627318962));
#135054=CARTESIAN_POINT('Ctrl Pts',(-20.9782974621631,-0.198929513972592,
-6.42626996190927));
#135055=CARTESIAN_POINT('Ctrl Pts',(-20.9566364666845,-0.1810446913926,
-6.42482654959232));
#135056=CARTESIAN_POINT('Ctrl Pts',(-20.9082215771356,-0.138795493085473,
-6.42147212821899));
#135057=CARTESIAN_POINT('Ctrl Pts',(-20.881813112811,-0.114061917786863,
-6.41954708107062));
#135058=CARTESIAN_POINT('Ctrl Pts',(-20.7888175167438,-0.0206155256541241,
-6.41240637985316));
#135059=CARTESIAN_POINT('Ctrl Pts',(-20.727794450089,0.053315868740702,
-6.40698564829393));
#135060=CARTESIAN_POINT('Ctrl Pts',(-20.6333894536693,0.192159711004867,
-6.3974279864016));
#135061=CARTESIAN_POINT('Ctrl Pts',(-20.5970086062709,0.254691521244603,
-6.39331852025902));
#135062=CARTESIAN_POINT('Ctrl Pts',(-20.5552227476554,0.339733896410683,
-6.38815766930478));
#135063=CARTESIAN_POINT('Ctrl Pts',(-20.5457452578314,0.360137804077088,
-6.38695033880945));
#135064=CARTESIAN_POINT('Ctrl Pts',(-20.5302659605582,0.395465004514892,
-6.38492122329409));
#135065=CARTESIAN_POINT('Ctrl Pts',(-20.5240457433938,0.410286677399196,
-6.38408853577244));
#135066=CARTESIAN_POINT('Ctrl Pts',(-20.509425406014,0.446709175401514,
-6.38208667830427));
#135067=CARTESIAN_POINT('Ctrl Pts',(-20.5012783785832,0.468406484994799,
-6.38093053177392));
#135068=CARTESIAN_POINT('Ctrl Pts',(-20.4839962705789,0.517785110231488,
-6.37836406239133));
#135069=CARTESIAN_POINT('Ctrl Pts',(-20.4751504511113,0.545558494229956,
-6.37696543244));
#135070=CARTESIAN_POINT('Ctrl Pts',(-20.446333687969,0.645767596038787,
-6.37202730282894));
#135071=CARTESIAN_POINT('Ctrl Pts',(-20.4308713361058,0.719390317600381,
-6.36859432163417));
#135072=CARTESIAN_POINT('Ctrl Pts',(-20.4109184264138,0.867394565708439,
-6.36165839645302));
#135073=CARTESIAN_POINT('Ctrl Pts',(-20.4063227858988,0.941555743434317,
-6.35816487654251));
#135074=CARTESIAN_POINT('Ctrl Pts',(-20.4074069935842,1.04773290587426,
-6.35294860163666));
#135075=CARTESIAN_POINT('Ctrl Pts',(-20.4087275525422,1.07969115724474,
-6.35135169440429));
#135076=CARTESIAN_POINT('Ctrl Pts',(-20.4130748840943,1.13964928531475,
-6.3482940066114));
#135077=CARTESIAN_POINT('Ctrl Pts',(-20.4158770275671,1.16765234748434,
-6.34684051975046));
#135078=CARTESIAN_POINT('Ctrl Pts',(-20.4244449069659,1.2347084391863,-6.34329366542665));
#135079=CARTESIAN_POINT('Ctrl Pts',(-20.4309463814792,1.27364602089609,
-6.34117932056259));
#135080=CARTESIAN_POINT('Ctrl Pts',(-20.4487420770081,1.35975358654683,
-6.33638099729633));
#135081=CARTESIAN_POINT('Ctrl Pts',(-20.4607816699277,1.40672626384451,
-6.33367939842577));
#135082=CARTESIAN_POINT('Ctrl Pts',(-20.5083340076015,1.56154109862775,
-6.32453935669608));
#135083=CARTESIAN_POINT('Ctrl Pts',(-20.553524172263,1.66602185052851,-6.31795301443009));
#135084=CARTESIAN_POINT('Ctrl Pts',(-20.6202965149974,1.78306409743752,
-6.31063225522325));
#135085=CARTESIAN_POINT('Ctrl Pts',(-20.6312101018548,1.80130769991334,
-6.30949396333953));
#135086=CARTESIAN_POINT('Ctrl Pts',(-20.6510730153479,1.83300566999782,
-6.30752892301034));
#135087=CARTESIAN_POINT('Ctrl Pts',(-20.659862053185,1.84655411008623,-6.30669390780339));
#135088=CARTESIAN_POINT('Ctrl Pts',(-20.6823976207191,1.88012662696967,
-6.30463470947974));
#135089=CARTESIAN_POINT('Ctrl Pts',(-20.6964068100095,1.89996827884071,
-6.3034258014671));
#135090=CARTESIAN_POINT('Ctrl Pts',(-20.7294275208484,1.94446844244388,
-6.30071397204598));
#135091=CARTESIAN_POINT('Ctrl Pts',(-20.7487287696739,1.96889907006515,
-6.29922472929941));
#135092=CARTESIAN_POINT('Ctrl Pts',(-20.8251818558492,2.05987013461749,
-6.29361229556627));
#135093=CARTESIAN_POINT('Ctrl Pts',(-20.8872293570132,2.12207838838893,
-6.28962278864746));
#135094=CARTESIAN_POINT('Ctrl Pts',(-20.9726354167221,2.19423119567501,
-6.28438479964871));
#135095=CARTESIAN_POINT('Ctrl Pts',(-20.9914011279391,2.20934582966756,
-6.28324849034829));
#135096=CARTESIAN_POINT('Ctrl Pts',(-21.0105083954618,2.22401163617983,
-6.28210099484077));
#135097=CARTESIAN_POINT('Origin',(21.9499999789786,0.999999999999992,-4.89578827641128));
#135098=CARTESIAN_POINT('Ctrl Pts',(22.889500458052,2.22400484060351,-6.32268396627741));
#135099=CARTESIAN_POINT('Ctrl Pts',(22.9437643008469,2.18235393808173,-6.32586239762496));
#135100=CARTESIAN_POINT('Ctrl Pts',(22.9951956853828,2.13714267871505,-6.32907681541136));
#135101=CARTESIAN_POINT('Ctrl Pts',(23.0631093143957,2.0689305661042,-6.33377182508186));
#135102=CARTESIAN_POINT('Ctrl Pts',(23.0822241961862,2.04866255736481,-6.33514921903181));
#135103=CARTESIAN_POINT('Ctrl Pts',(23.1196150714722,2.00680137313515,-6.33796850987336));
#135104=CARTESIAN_POINT('Ctrl Pts',(23.1378667184438,1.98520096915314,-6.33941052433828));
#135105=CARTESIAN_POINT('Ctrl Pts',(23.175820593364,1.93769463660604,-6.34256154195298));
#135106=CARTESIAN_POINT('Ctrl Pts',(23.1953172082192,1.9116425873736,-6.34427729204013));
#135107=CARTESIAN_POINT('Ctrl Pts',(23.2577255716203,1.82250918564089,-6.35011250822171));
#135108=CARTESIAN_POINT('Ctrl Pts',(23.2967779641055,1.75687153698208,-6.35435979606607));
#135109=CARTESIAN_POINT('Ctrl Pts',(23.3730325216872,1.60396707328758,-6.36403726486672));
#135110=CARTESIAN_POINT('Ctrl Pts',(23.4073766301252,1.5156082237948,-6.36948991197114));
#135111=CARTESIAN_POINT('Ctrl Pts',(23.44062749298,1.39945692921207,-6.37613025049715));
#135112=CARTESIAN_POINT('Ctrl Pts',(23.447199243024,1.37407316760549,-6.37754957858955));
#135113=CARTESIAN_POINT('Ctrl Pts',(23.4568118692577,1.33261671013395,-6.37980323811566));
#135114=CARTESIAN_POINT('Ctrl Pts',(23.4602495177829,1.31664231485889,-6.38065601132625));
#135115=CARTESIAN_POINT('Ctrl Pts',(23.4674421017827,1.2804315076925,-6.38255165984801));
#135116=CARTESIAN_POINT('Ctrl Pts',(23.4710471195632,1.26016936813628,-6.38358730609421));
#135117=CARTESIAN_POINT('Ctrl Pts',(23.4916006802992,1.12954626747083,-6.3901366029481));
#135118=CARTESIAN_POINT('Ctrl Pts',(23.496934793451,1.01768353663625,-6.39518397990132));
#135119=CARTESIAN_POINT('Ctrl Pts',(23.487078239273,0.855816002836622,-6.40272713885022));
#135120=CARTESIAN_POINT('Ctrl Pts',(23.4815372409517,0.805598702475043,
-6.40509780733745));
#135121=CARTESIAN_POINT('Ctrl Pts',(23.4671271473542,0.715715413179718,
-6.40947725420946));
#135122=CARTESIAN_POINT('Ctrl Pts',(23.4591348184108,0.675956349232925,
-6.41146326048851));
#135123=CARTESIAN_POINT('Ctrl Pts',(23.4428990601418,0.608966152625854,
-6.41491905342869));
#135124=CARTESIAN_POINT('Ctrl Pts',(23.4354514014897,0.581563532518983,
-6.41636441048629));
#135125=CARTESIAN_POINT('Ctrl Pts',(23.4180502203203,0.523877367121495,
-6.41948143109962));
#135126=CARTESIAN_POINT('Ctrl Pts',(23.4079058844485,0.49366567009403,-6.42115843521622));
#135127=CARTESIAN_POINT('Ctrl Pts',(23.374247668214,0.402846881396846,-6.42634106846));
#135128=CARTESIAN_POINT('Ctrl Pts',(23.3478353183392,0.34339637697697,-6.42993261983137));
#135129=CARTESIAN_POINT('Ctrl Pts',(23.2796645464399,0.21284467531784,-6.43822575523003));
#135130=CARTESIAN_POINT('Ctrl Pts',(23.2357993549451,0.143063056448227,
-6.44295801734837));
#135131=CARTESIAN_POINT('Ctrl Pts',(23.1684521806485,0.0528243095948877,
-6.44928838236166));
#135132=CARTESIAN_POINT('Ctrl Pts',(23.1496122899442,0.0290736305479866,
-6.45097552873429));
#135133=CARTESIAN_POINT('Ctrl Pts',(23.1147295976499,-0.0123348835206993,
-6.45393508227006));
#135134=CARTESIAN_POINT('Ctrl Pts',(23.0989538246302,-0.0302049200618226,
-6.45521865955291));
#135135=CARTESIAN_POINT('Ctrl Pts',(23.0717979693521,-0.0595656490477214,
-6.45732827442608));
#135136=CARTESIAN_POINT('Ctrl Pts',(23.0606408571012,-0.0712548669842761,
-6.45816784678587));
#135137=CARTESIAN_POINT('Ctrl Pts',(23.0337523306823,-0.0985539540488167,
-6.46012757782062));
#135138=CARTESIAN_POINT('Ctrl Pts',(23.0178648761823,-0.114003861819678,
-6.46123704524837));
#135139=CARTESIAN_POINT('Ctrl Pts',(22.9401855826268,-0.186354305817296,
-6.46646535512513));
#135140=CARTESIAN_POINT('Ctrl Pts',(22.8741446509117,-0.238492231703882,
-6.47033922117249));
#135141=CARTESIAN_POINT('Ctrl Pts',(22.751516819588,-0.320007256122885,
-6.47715656516353));
#135142=CARTESIAN_POINT('Ctrl Pts',(22.6967491804622,-0.351744659790034,
-6.48008594248547));
#135143=CARTESIAN_POINT('Ctrl Pts',(22.5987738286207,-0.400744765220158,
-6.48530562827809));
#135144=CARTESIAN_POINT('Ctrl Pts',(22.5564481505334,-0.419582183915144,
-6.48755363697606));
#135145=CARTESIAN_POINT('Ctrl Pts',(22.4862438984667,-0.44711390931647,
-6.49131211381761));
#135146=CARTESIAN_POINT('Ctrl Pts',(22.4588522655957,-0.456971317445483,
-6.49278541236058));
#135147=CARTESIAN_POINT('Ctrl Pts',(22.4024372406223,-0.475488361222527,
-6.49584106219699));
#135148=CARTESIAN_POINT('Ctrl Pts',(22.3734050104377,-0.484079983098811,
-6.49742475536692));
#135149=CARTESIAN_POINT('Ctrl Pts',(22.2903762349551,-0.506016376353173,
-6.50199043079261));
#135150=CARTESIAN_POINT('Ctrl Pts',(22.2358883509165,-0.517302952110055,
-6.50503133700028));
#135151=CARTESIAN_POINT('Ctrl Pts',(22.0875172306779,-0.539759982591068,
-6.51340338646219));
#135152=CARTESIAN_POINT('Ctrl Pts',(21.9930209423237,-0.545289469972139,
-6.51884309799928));
#135153=CARTESIAN_POINT('Ctrl Pts',(21.8666520621711,-0.541079243741303,
-6.52596583927362));
#135154=CARTESIAN_POINT('Ctrl Pts',(21.8347231308639,-0.539020315515715,
-6.52775079035233));
#135155=CARTESIAN_POINT('Ctrl Pts',(21.7782637085599,-0.533612460159687,
-6.53085755966035));
#135156=CARTESIAN_POINT('Ctrl Pts',(21.7537062659276,-0.530663068646278,
-6.53219208194916));
#135157=CARTESIAN_POINT('Ctrl Pts',(21.7131803188534,-0.524804379576196,
-6.53435528675913));
#135158=CARTESIAN_POINT('Ctrl Pts',(21.6971690217876,-0.522231427441526,
-6.53519932508586));
#135159=CARTESIAN_POINT('Ctrl Pts',(21.660404585231,-0.515727371555119,
-6.5371117777072));
#135160=CARTESIAN_POINT('Ctrl Pts',(21.6396865464047,-0.511621848385371,
-6.53817174118872));
#135161=CARTESIAN_POINT('Ctrl Pts',(21.5286161950409,-0.487231967237438,
-6.54378841661526));
#135162=CARTESIAN_POINT('Ctrl Pts',(21.4401370515953,-0.459269019950006,
-6.54803512904835));
#135163=CARTESIAN_POINT('Ctrl Pts',(21.299853908761,-0.400604312704793,
-6.5550781790296));
#135164=CARTESIAN_POINT('Ctrl Pts',(21.2463866893962,-0.374521838360011,
-6.55784138945292));
#135165=CARTESIAN_POINT('Ctrl Pts',(21.1555814175104,-0.323535564518975,
-6.56281568134926));
#135166=CARTESIAN_POINT('Ctrl Pts',(21.1175755322744,-0.29996783600625,
-6.56499082150684));
#135167=CARTESIAN_POINT('Ctrl Pts',(21.0567744575371,-0.258503943642658,
-6.56866413327037));
#135168=CARTESIAN_POINT('Ctrl Pts',(21.0333640765504,-0.241556480562992,
-6.57012883332864));
#135169=CARTESIAN_POINT('Ctrl Pts',(20.9861674288754,-0.205326705468321,
-6.57319467015804));
#135170=CARTESIAN_POINT('Ctrl Pts',(20.9624516782821,-0.185973792134488,
-6.5747980796891));
#135171=CARTESIAN_POINT('Ctrl Pts',(20.895069857232,-0.127564665502109,
-6.57954622892622));
#135172=CARTESIAN_POINT('Ctrl Pts',(20.8530358759571,-0.0867144713952817,
-6.58275842908974));
#135173=CARTESIAN_POINT('Ctrl Pts',(20.7430205123819,0.0331045016887321,
-6.59185976021977));
#135174=CARTESIAN_POINT('Ctrl Pts',(20.680557511281,0.116710214052071,-6.59788082635173));
#135175=CARTESIAN_POINT('Ctrl Pts',(20.6087931150197,0.236283153847814,
-6.60566015045069));
#135176=CARTESIAN_POINT('Ctrl Pts',(20.591643457666,0.267219581433107,-6.60760327755508));
#135177=CARTESIAN_POINT('Ctrl Pts',(20.5675643604903,0.314411850406251,
-6.61043679718368));
#135178=CARTESIAN_POINT('Ctrl Pts',(20.5598266162508,0.330240764197565,
-6.61136590244031));
#135179=CARTESIAN_POINT('Ctrl Pts',(20.5447766746547,0.362413239865487,
-6.61320664452485));
#135180=CARTESIAN_POINT('Ctrl Pts',(20.5374744452525,0.378758434017095,
-6.61411771979798));
#135181=CARTESIAN_POINT('Ctrl Pts',(20.5158367981773,0.429547049152643,
-6.61688547626871));
#135182=CARTESIAN_POINT('Ctrl Pts',(20.5024640578692,0.464387549626548,
-6.61869595346582));
#135183=CARTESIAN_POINT('Ctrl Pts',(20.4701373990076,0.558697423726744,
-6.62344523994509));
#135184=CARTESIAN_POINT('Ctrl Pts',(20.4535053242237,0.618889071572606,
-6.62632157129356));
#135185=CARTESIAN_POINT('Ctrl Pts',(20.4233668602429,0.761018257768411,
-6.63304964922663));
#135186=CARTESIAN_POINT('Ctrl Pts',(20.4127347180812,0.843362645664008,
-6.63690553919466));
#135187=CARTESIAN_POINT('Ctrl Pts',(20.407091732587,0.961142571795386,-6.64264953999652));
#135188=CARTESIAN_POINT('Ctrl Pts',(20.4066073242446,0.996172655188285,
-6.64438506069481));
#135189=CARTESIAN_POINT('Ctrl Pts',(20.4078823562372,1.05924206190599,-6.6475741616009));
#135190=CARTESIAN_POINT('Ctrl Pts',(20.4092146679806,1.08727474894511,-6.64901452110638));
#135191=CARTESIAN_POINT('Ctrl Pts',(20.4139627268901,1.15066308713468,-6.65232904425536));
#135192=CARTESIAN_POINT('Ctrl Pts',(20.4178362778303,1.18596757428787,-6.6542159832979));
#135193=CARTESIAN_POINT('Ctrl Pts',(20.4287909704093,1.26162675880698,-6.65835021399949));
#135194=CARTESIAN_POINT('Ctrl Pts',(20.4362682724006,1.30189632250002,-6.66060693363008));
#135195=CARTESIAN_POINT('Ctrl Pts',(20.4671266317164,1.43773259514078,-6.66839158565604));
#135196=CARTESIAN_POINT('Ctrl Pts',(20.4980349893845,1.53133745335054,-6.67406684576527));
#135197=CARTESIAN_POINT('Ctrl Pts',(20.5533792694773,1.6571355467828,-6.68177795249405));
#135198=CARTESIAN_POINT('Ctrl Pts',(20.5704727173108,1.69230155551479,-6.68394077780806));
#135199=CARTESIAN_POINT('Ctrl Pts',(20.5977766696573,1.74343631298846,-6.6870594387879));
#135200=CARTESIAN_POINT('Ctrl Pts',(20.6069745156197,1.75992637711794,-6.68806087354461));
#135201=CARTESIAN_POINT('Ctrl Pts',(20.6249894061157,1.7908745519929,-6.68992626393878));
#135202=CARTESIAN_POINT('Ctrl Pts',(20.6337459161862,1.80536378700923,-6.6907930348651));
#135203=CARTESIAN_POINT('Ctrl Pts',(20.6590573462398,1.84573024410616,-6.6931966369645));
#135204=CARTESIAN_POINT('Ctrl Pts',(20.6761498403642,1.8712626251278,-6.69470404293512));
#135205=CARTESIAN_POINT('Ctrl Pts',(20.7199058994271,1.93258111984863,-6.69833371665423));
#135206=CARTESIAN_POINT('Ctrl Pts',(20.7473813800819,1.96775401116228,-6.70042440363885));
#135207=CARTESIAN_POINT('Ctrl Pts',(20.8533343207297,2.09189681237628,-6.70801304148536));
#135208=CARTESIAN_POINT('Ctrl Pts',(20.9404625637073,2.17292247844536,-6.71342017695837));
#135209=CARTESIAN_POINT('Ctrl Pts',(21.0621458576958,2.26238519948046,-6.72083468934783));
#135210=CARTESIAN_POINT('Ctrl Pts',(21.0888801661886,2.2807707908411,-6.72245357899984));
#135211=CARTESIAN_POINT('Ctrl Pts',(21.139972488864,2.31358460660175,-6.72554071388244));
#135212=CARTESIAN_POINT('Ctrl Pts',(21.1641867323002,2.32821175374242,-6.72700107400664));
#135213=CARTESIAN_POINT('Ctrl Pts',(21.2229884635093,2.36156128605233,-6.73054630594845));
#135214=CARTESIAN_POINT('Ctrl Pts',(21.2579152940554,2.37964246114793,-6.7326514923484));
#135215=CARTESIAN_POINT('Ctrl Pts',(21.3369800858114,2.41681501954508,-6.73741595938099));
#135216=CARTESIAN_POINT('Ctrl Pts',(21.3813963494781,2.43521691975713,-6.74009216476792));
#135217=CARTESIAN_POINT('Ctrl Pts',(21.5073782212088,2.48064485645767,-6.74764416940453));
#135218=CARTESIAN_POINT('Ctrl Pts',(21.5904489791571,2.50297906165908,-6.75258739415442));
#135219=CARTESIAN_POINT('Ctrl Pts',(21.7122856226903,2.5250511234118,-6.75951541783196));
#135220=CARTESIAN_POINT('Ctrl Pts',(21.7498650751572,2.53043635240697,-6.76160765623574));
#135221=CARTESIAN_POINT('Ctrl Pts',(21.8054988143049,2.5363242221215,-6.76460536335205));
#135222=CARTESIAN_POINT('Ctrl Pts',(21.823423168918,2.53790476624975,-6.76555599408177));
#135223=CARTESIAN_POINT('Ctrl Pts',(21.8588668545299,2.54040623025768,-6.76740050787923));
#135224=CARTESIAN_POINT('Ctrl Pts',(21.8763822221601,2.54134261800288,-6.76829490683412));
#135225=CARTESIAN_POINT('Ctrl Pts',(21.9287134532859,2.54324617143663,-6.77092569723392));
#135226=CARTESIAN_POINT('Ctrl Pts',(21.9635516264176,2.54333356821809,-6.77262250926825));
#135227=CARTESIAN_POINT('Ctrl Pts',(22.1068607274314,2.53883938259562,-6.77947949458667));
#135228=CARTESIAN_POINT('Ctrl Pts',(22.2146981090058,2.52399774847878,-6.78436947284413));
#135229=CARTESIAN_POINT('Ctrl Pts',(22.3745615522837,2.48450154673247,-6.79212242091079));
#135230=CARTESIAN_POINT('Ctrl Pts',(22.4282556192527,2.4680831789754,-6.79481301565766));
#135231=CARTESIAN_POINT('Ctrl Pts',(22.5094076935878,2.43834337153749,-6.79909154459208));
#135232=CARTESIAN_POINT('Ctrl Pts',(22.5375664105778,2.42707189056893,-6.8006166790024));
#135233=CARTESIAN_POINT('Ctrl Pts',(22.5920213244423,2.40338946713281,-6.80365531411678));
#135234=CARTESIAN_POINT('Ctrl Pts',(22.6183350435291,2.39105050305001,-6.80516601174385));
#135235=CARTESIAN_POINT('Ctrl Pts',(22.6765353482745,2.36172669227281,-6.80860798388125));
#135236=CARTESIAN_POINT('Ctrl Pts',(22.708204780748,2.3443505645048,-6.81055134782412));
#135237=CARTESIAN_POINT('Ctrl Pts',(22.7912818291088,2.29489871651529,-6.81583963967357));
#135238=CARTESIAN_POINT('Ctrl Pts',(22.8414566079082,2.26088142700837,-6.81923966280967));
#135239=CARTESIAN_POINT('Ctrl Pts',(22.8894991487533,2.22400584557124,-6.82267583049642));
#135240=CARTESIAN_POINT('Ctrl Pts',(22.8894916066884,2.22401163452936,-6.78051560659813));
#135241=CARTESIAN_POINT('Ctrl Pts',(22.8840931829709,2.22815520125885,-6.78013331794407));
#135242=CARTESIAN_POINT('Ctrl Pts',(22.8786669161915,2.23226338446389,-6.77975186021311));
#135243=CARTESIAN_POINT('Ctrl Pts',(22.8518487668555,2.2522893892527,-6.77788090947732));
#135244=CARTESIAN_POINT('Ctrl Pts',(22.830073521286,2.2676871181595,-6.77640617520325));
#135245=CARTESIAN_POINT('Ctrl Pts',(22.7897835548849,2.29463821236672,-6.77377117239461));
#135246=CARTESIAN_POINT('Ctrl Pts',(22.7714018742259,2.30637803644346,-6.77260286395183));
#135247=CARTESIAN_POINT('Ctrl Pts',(22.7389786896359,2.3261307014459,-6.77060845819639));
#135248=CARTESIAN_POINT('Ctrl Pts',(22.7250504636334,2.33431885929378,-6.76977300307344));
#135249=CARTESIAN_POINT('Ctrl Pts',(22.6899501003446,2.35421860565912,-6.76771819252665));
#135250=CARTESIAN_POINT('Ctrl Pts',(22.6686269459659,2.36565354765244,-6.76651389728743));
#135251=CARTESIAN_POINT('Ctrl Pts',(22.5407643180451,2.43039771643578,-6.75949987971156));
#135252=CARTESIAN_POINT('Ctrl Pts',(22.4286034762515,2.47172818012277,-6.75415828547375));
#135253=CARTESIAN_POINT('Ctrl Pts',(22.2706083637621,2.5099480869076,-6.74654133461936));
#135254=CARTESIAN_POINT('Ctrl Pts',(22.2280104735494,2.51836848209117,-6.74448249074873));
#135255=CARTESIAN_POINT('Ctrl Pts',(22.1486955342246,2.53059695792077,-6.74059127163562));
#135256=CARTESIAN_POINT('Ctrl Pts',(22.1120876658938,2.53490530697078,-6.73877304185693));
#135257=CARTESIAN_POINT('Ctrl Pts',(22.0473899727701,2.54017915697149,-6.73550200032558));
#135258=CARTESIAN_POINT('Ctrl Pts',(22.0193619581218,2.54169563633919,-6.73406611077397));
#135259=CARTESIAN_POINT('Ctrl Pts',(21.9575124536453,2.5433520677348,-6.73085020387539));
#135260=CARTESIAN_POINT('Ctrl Pts',(21.9236969047742,2.54314612563261,-6.72906071477139));
#135261=CARTESIAN_POINT('Ctrl Pts',(21.7713623908797,2.53720985684749,-6.72085285723711));
#135262=CARTESIAN_POINT('Ctrl Pts',(21.6537480387357,2.51893167321256,-6.71407409434332));
#135263=CARTESIAN_POINT('Ctrl Pts',(21.498863030427,2.47617536862273,-6.70494939127576));
#135264=CARTESIAN_POINT('Ctrl Pts',(21.458789916911,2.46332881297855,-6.7025746245593));
#135265=CARTESIAN_POINT('Ctrl Pts',(21.3914977318376,2.43868006049563,-6.69861050217562));
#135266=CARTESIAN_POINT('Ctrl Pts',(21.3640020083109,2.42770152835382,-6.6969978915552));
#135267=CARTESIAN_POINT('Ctrl Pts',(21.3214649612704,2.40928115321159,-6.69453224843813));
#135268=CARTESIAN_POINT('Ctrl Pts',(21.306200696785,2.40237377604644,-6.69365363547436));
#135269=CARTESIAN_POINT('Ctrl Pts',(21.2737187776936,2.38703285237926,-6.69180118471747));
#135270=CARTESIAN_POINT('Ctrl Pts',(21.256540224098,2.37852458449533,-6.69083130454782));
#135271=CARTESIAN_POINT('Ctrl Pts',(21.2031676882277,2.35083971776745,-6.68783582185984));
#135272=CARTESIAN_POINT('Ctrl Pts',(21.1675743567698,2.33054010600596,-6.6858642297926));
#135273=CARTESIAN_POINT('Ctrl Pts',(21.0611400029486,2.26408844206428,-6.67992892815794));
#135274=CARTESIAN_POINT('Ctrl Pts',(20.9932480484945,2.21351481213039,-6.67607947826741));
#135275=CARTESIAN_POINT('Ctrl Pts',(20.8809964866106,2.1145934459105,-6.6690874217422));
#135276=CARTESIAN_POINT('Ctrl Pts',(20.8349311676575,2.068507187801,-6.66599421617396));
#135277=CARTESIAN_POINT('Ctrl Pts',(20.7712728118056,1.99620637292017,-6.66124461787238));
#135278=CARTESIAN_POINT('Ctrl Pts',(20.7513470972283,1.97213989531612,-6.6596794543379));
#135279=CARTESIAN_POINT('Ctrl Pts',(20.7146269435313,1.92494233273732,-6.65662929477761));
#135280=CARTESIAN_POINT('Ctrl Pts',(20.6977177555909,1.90191682112566,-6.65514953412702));
#135281=CARTESIAN_POINT('Ctrl Pts',(20.6574383238106,1.84374964845012,-6.65142624429221));
#135282=CARTESIAN_POINT('Ctrl Pts',(20.6348530691273,1.80809484780244,-6.64915642623132));
#135283=CARTESIAN_POINT('Ctrl Pts',(20.5569865088252,1.6732403373715,-6.64061941759587));
#135284=CARTESIAN_POINT('Ctrl Pts',(20.5112432376026,1.56895840254702,-6.63407846001082));
#135285=CARTESIAN_POINT('Ctrl Pts',(20.467180058202,1.42808431637099,-6.62574395041717));
#135286=CARTESIAN_POINT('Ctrl Pts',(20.4580841195376,1.39521938524899,-6.62383600647422));
#135287=CARTESIAN_POINT('Ctrl Pts',(20.4440281814812,1.33699250020193,-6.62054676086045));
#135288=CARTESIAN_POINT('Ctrl Pts',(20.438602324927,1.31175675253409,-6.61915070769246));
#135289=CARTESIAN_POINT('Ctrl Pts',(20.4308156970049,1.27053406387355,-6.6169304188676));
#135290=CARTESIAN_POINT('Ctrl Pts',(20.428068587813,1.25462614839134,-6.61608833984631));
#135291=CARTESIAN_POINT('Ctrl Pts',(20.4223782303219,1.21828175639506,-6.61419997008572));
#135292=CARTESIAN_POINT('Ctrl Pts',(20.4195945534745,1.19782427487334,-6.61316136543443));
#135293=CARTESIAN_POINT('Ctrl Pts',(20.4103699967504,1.11808425446866,-6.6091869222361));
#135294=CARTESIAN_POINT('Ctrl Pts',(20.4069565145037,1.05850030743707,-6.60637404577534));
#135295=CARTESIAN_POINT('Ctrl Pts',(20.4070878771545,0.879979125521468,
-6.59805821849222));
#135296=CARTESIAN_POINT('Ctrl Pts',(20.4209139176431,0.761509420213065,
-6.59265579470078));
#135297=CARTESIAN_POINT('Ctrl Pts',(20.4559557337416,0.612932441158596,
-6.58519450407706));
#135298=CARTESIAN_POINT('Ctrl Pts',(20.4647846174834,0.580327949192161,
-6.58351596820535));
#135299=CARTESIAN_POINT('Ctrl Pts',(20.4828917995404,0.521220934336388,
-6.5803833676819));
#135300=CARTESIAN_POINT('Ctrl Pts',(20.4918373460953,0.494631410075126,
-6.57894008721395));
#135301=CARTESIAN_POINT('Ctrl Pts',(20.5141995513575,0.433710413910999,
-6.57554834688385));
#135302=CARTESIAN_POINT('Ctrl Pts',(20.5281310980393,0.399587342221404,
-6.5735843877792));
#135303=CARTESIAN_POINT('Ctrl Pts',(20.5611066216066,0.326420996188346,
-6.56923008950995));
#135304=CARTESIAN_POINT('Ctrl Pts',(20.5806045083557,0.287617317350972,
-6.56682785975829));
#135305=CARTESIAN_POINT('Ctrl Pts',(20.6597049123616,0.1454759886516,-6.55770389375578));
#135306=CARTESIAN_POINT('Ctrl Pts',(20.7295823956875,0.0483421189603384,
-6.55076608976156));
#135307=CARTESIAN_POINT('Ctrl Pts',(20.8261911071129,-0.0575839008484547,
-6.54292385490149));
#135308=CARTESIAN_POINT('Ctrl Pts',(20.8428511354534,-0.0750123930301116,
-6.54162466241861));
#135309=CARTESIAN_POINT('Ctrl Pts',(20.8713413936361,-0.103451576259399,
-6.53950005581383));
#135310=CARTESIAN_POINT('Ctrl Pts',(20.882947502136,-0.114678785293956,
-6.53866050857244));
#135311=CARTESIAN_POINT('Ctrl Pts',(20.9106741103289,-0.140670152489015,
-6.53671559668221));
#135312=CARTESIAN_POINT('Ctrl Pts',(20.9269356295874,-0.15527749260217,
-6.53562031896456));
#135313=CARTESIAN_POINT('Ctrl Pts',(20.963775794222,-0.186981991820656,
-6.53322419177594));
#135314=CARTESIAN_POINT('Ctrl Pts',(20.9844999103353,-0.203899549018343,
-6.53193256269565));
#135315=CARTESIAN_POINT('Ctrl Pts',(21.054763183386,-0.258275061804536,
-6.52769968262103));
#135316=CARTESIAN_POINT('Ctrl Pts',(21.1061234807423,-0.293281901160238,
-6.5248362596312));
#135317=CARTESIAN_POINT('Ctrl Pts',(21.2310655043174,-0.367821419251677,
-6.51809965527141));
#135318=CARTESIAN_POINT('Ctrl Pts',(21.3060179359046,-0.404666552556696,
-6.51422243412655));
#135319=CARTESIAN_POINT('Ctrl Pts',(21.416153512383,-0.448131064296362,
-6.50845502411498));
#135320=CARTESIAN_POINT('Ctrl Pts',(21.4491582203328,-0.459874289426101,
-6.50671969329122));
#135321=CARTESIAN_POINT('Ctrl Pts',(21.5092427555379,-0.478975188539539,
-6.50353255105917));
#135322=CARTESIAN_POINT('Ctrl Pts',(21.5361782121453,-0.48673668019922,
-6.50209400370346));
#135323=CARTESIAN_POINT('Ctrl Pts',(21.5975933806693,-0.502635276219801,
-6.498786420574));
#135324=CARTESIAN_POINT('Ctrl Pts',(21.6321711152116,-0.510327030653523,
-6.49690474642806));
#135325=CARTESIAN_POINT('Ctrl Pts',(21.7070880248085,-0.524305528313742,
-6.49278423021513));
#135326=CARTESIAN_POINT('Ctrl Pts',(21.7474736554734,-0.530194861139748,
-6.49053608178524));
#135327=CARTESIAN_POINT('Ctrl Pts',(21.8849570246883,-0.544705579414959,
-6.48281215151114));
#135328=CARTESIAN_POINT('Ctrl Pts',(21.9826160321093,-0.545729839865223,
-6.47719181880399));
#135329=CARTESIAN_POINT('Ctrl Pts',(22.119445509224,-0.53418606024692,-6.46948177352854));
#135330=CARTESIAN_POINT('Ctrl Pts',(22.1590326063599,-0.529295396342859,
-6.46727346182807));
#135331=CARTESIAN_POINT('Ctrl Pts',(22.2171500931561,-0.51981617261752,
-6.46410375767297));
#135332=CARTESIAN_POINT('Ctrl Pts',(22.2358549284144,-0.516409375835991,
-6.46309486077475));
#135333=CARTESIAN_POINT('Ctrl Pts',(22.2710413790207,-0.509326462490085,
-6.46122427240631));
#135334=CARTESIAN_POINT('Ctrl Pts',(22.2875341176328,-0.505723967756331,
-6.46035947151717));
#135335=CARTESIAN_POINT('Ctrl Pts',(22.3334753671109,-0.494896276698613,
-6.45797691954056));
#135336=CARTESIAN_POINT('Ctrl Pts',(22.3627762470728,-0.487072361160386,
-6.45648757275791));
#135337=CARTESIAN_POINT('Ctrl Pts',(22.4336930571506,-0.465878281295291,
-6.45291725494369));
#135338=CARTESIAN_POINT('Ctrl Pts',(22.4750085545412,-0.451593759290283,
-6.45086637768186));
#135339=CARTESIAN_POINT('Ctrl Pts',(22.6213211387481,-0.393941787310652,
-6.44354608404348));
#135340=CARTESIAN_POINT('Ctrl Pts',(22.7220534181049,-0.340775273734657,
-6.43836812109678));
#135341=CARTESIAN_POINT('Ctrl Pts',(22.8445642454575,-0.257692989729819,
-6.43114461131943));
#135342=CARTESIAN_POINT('Ctrl Pts',(22.8724315858372,-0.237399128054494,
-6.42943411332381));
#135343=CARTESIAN_POINT('Ctrl Pts',(22.921732874008,-0.198904935814554,
-6.42626810994936));
#135344=CARTESIAN_POINT('Ctrl Pts',(22.9433937173593,-0.181019312596473,
-6.42482465495505));
#135345=CARTESIAN_POINT('Ctrl Pts',(22.9918147952299,-0.138762512766051,
-6.4214696779132));
#135346=CARTESIAN_POINT('Ctrl Pts',(23.0182291685037,-0.114021676901523,
-6.41954409982678));
#135347=CARTESIAN_POINT('Ctrl Pts',(23.1112963858827,-0.0204951197811365,
-6.41239742905592));
#135348=CARTESIAN_POINT('Ctrl Pts',(23.1723720004862,0.0535208882474469,
-6.40697078512297));
#135349=CARTESIAN_POINT('Ctrl Pts',(23.266729171269,0.192364277332073,-6.39741470329425));
#135350=CARTESIAN_POINT('Ctrl Pts',(23.3030397516549,0.254791455240788,
-6.39331263114128));
#135351=CARTESIAN_POINT('Ctrl Pts',(23.3447720161121,0.33972276701939,-6.38815846847536));
#135352=CARTESIAN_POINT('Ctrl Pts',(23.3542504995107,0.360128422700714,
-6.38695102416488));
#135353=CARTESIAN_POINT('Ctrl Pts',(23.3697307558064,0.395457295352428,
-6.38492179943724));
#135354=CARTESIAN_POINT('Ctrl Pts',(23.3759510206594,0.410278855129356,
-6.38408911225237));
#135355=CARTESIAN_POINT('Ctrl Pts',(23.3905706399993,0.446698980537339,
-6.38208737200271));
#135356=CARTESIAN_POINT('Ctrl Pts',(23.3987169996827,0.468393993728911,
-6.38093133740976));
#135357=CARTESIAN_POINT('Ctrl Pts',(23.4159974082986,0.517766152213794,
-6.37836517799455));
#135358=CARTESIAN_POINT('Ctrl Pts',(23.424842325753,0.545535327396278,-6.3769667417294));
#135359=CARTESIAN_POINT('Ctrl Pts',(23.4536527927569,0.645715557503674,
-6.3720299703545));
#135360=CARTESIAN_POINT('Ctrl Pts',(23.4691131058387,0.719312849991645,
-6.36859809863064));
#135361=CARTESIAN_POINT('Ctrl Pts',(23.4890770279367,0.867323398095032,
-6.36166190593236));
#135362=CARTESIAN_POINT('Ctrl Pts',(23.493677344455,0.941517396790919,-6.35816691881182));
#135363=CARTESIAN_POINT('Ctrl Pts',(23.492593171557,1.04772775196917,-6.35294902417737));
#135364=CARTESIAN_POINT('Ctrl Pts',(23.491272705243,1.07968628112634,-6.35135210632943));
#135365=CARTESIAN_POINT('Ctrl Pts',(23.4869255573007,1.13964435966628,-6.34829442666829));
#135366=CARTESIAN_POINT('Ctrl Pts',(23.4841235401043,1.16764709644041,-6.34684095963345));
#135367=CARTESIAN_POINT('Ctrl Pts',(23.4755561461554,1.23470133033093,-6.34329421128866));
#135368=CARTESIAN_POINT('Ctrl Pts',(23.4690551312463,1.27363739727861,-6.34117995530574));
#135369=CARTESIAN_POINT('Ctrl Pts',(23.4512609260417,1.35974065703618,-6.33638189067511));
#135370=CARTESIAN_POINT('Ctrl Pts',(23.4392225156365,1.40671058667802,-6.33368046478458));
#135371=CARTESIAN_POINT('Ctrl Pts',(23.3916706808293,1.56153063553269,-6.32454017074507));
#135372=CARTESIAN_POINT('Ctrl Pts',(23.3464779068928,1.66601881761278,-6.31795334965074));
#135373=CARTESIAN_POINT('Ctrl Pts',(23.2797017797471,1.78306697197067,-6.31063222170074));
#135374=CARTESIAN_POINT('Ctrl Pts',(23.2687885574923,1.8013098857123,-6.30949397324053));
#135375=CARTESIAN_POINT('Ctrl Pts',(23.248926102489,1.83300704257971,-6.30752898423778));
#135376=CARTESIAN_POINT('Ctrl Pts',(23.2401371351826,1.84655534405131,-6.30669397812446));
#135377=CARTESIAN_POINT('Ctrl Pts',(23.2176015009986,1.8801278980579,-6.30463477886682));
#135378=CARTESIAN_POINT('Ctrl Pts',(23.2035921619174,1.89996971688336,-6.30342586172547));
#135379=CARTESIAN_POINT('Ctrl Pts',(23.1705709844292,1.94447038942134,-6.30071400387885));
#135380=CARTESIAN_POINT('Ctrl Pts',(23.151269405167,1.96890134786215,-6.29922474256441));
#135381=CARTESIAN_POINT('Ctrl Pts',(23.0748138740875,2.05987491672823,-6.29361215898745));
#135382=CARTESIAN_POINT('Ctrl Pts',(23.0127639054047,2.12208500635517,-6.2896225304504));
#135383=CARTESIAN_POINT('Ctrl Pts',(22.9273581178032,2.19423640340638,-6.28438459941712));
#135384=CARTESIAN_POINT('Ctrl Pts',(22.9085955731876,2.20934836206942,-6.28324848751454));
#135385=CARTESIAN_POINT('Ctrl Pts',(22.8894915905204,2.22401164693913,-6.28210119346687));
#135386=CARTESIAN_POINT('Origin',(21.9499999789786,0.999999999999992,-6.00000000000001));
#135387=CARTESIAN_POINT('',(20.6853192846384,1.00091784636197,-6.44310594448828));
#135388=CARTESIAN_POINT('Ctrl Pts',(22.3906686064029,-0.185465307624328,
-6.28967669732482));
#135389=CARTESIAN_POINT('Ctrl Pts',(22.3471104093517,-0.201760426698602,
-6.29243744842554));
#135390=CARTESIAN_POINT('Ctrl Pts',(22.3026975844951,-0.215616979717695,
-6.29522313617549));
#135391=CARTESIAN_POINT('Ctrl Pts',(22.2577300141014,-0.226935083304443,
-6.29808537729643));
#135392=CARTESIAN_POINT('Ctrl Pts',(22.2546229511194,-0.227717114896844,
-6.29828314567384));
#135393=CARTESIAN_POINT('Ctrl Pts',(22.2515132255729,-0.228487042529604,
-6.2984812795329));
#135394=CARTESIAN_POINT('Ctrl Pts',(22.2484009299199,-0.229244839827862,
-6.29867979590079));
#135395=CARTESIAN_POINT('Ctrl Pts',(22.234150207789,-0.232714676865598,
-6.29958877175418));
#135396=CARTESIAN_POINT('Ctrl Pts',(22.2198461265754,-0.23593014822109,
-6.3005058046491));
#135397=CARTESIAN_POINT('Ctrl Pts',(22.2054985961248,-0.238888984456219,
-6.30143257033421));
#135398=CARTESIAN_POINT('Ctrl Pts',(22.20548208595,-0.238892389286325,-6.30143363679394));
#135399=CARTESIAN_POINT('Ctrl Pts',(22.2054655757175,-0.238895793776658,
-6.30143470326657));
#135400=CARTESIAN_POINT('Ctrl Pts',(22.2054490654275,-0.238899197927225,
-6.30143576975208));
#135401=CARTESIAN_POINT('Ctrl Pts',(22.1604907218272,-0.24816886980053,
-6.30433986302597));
#135402=CARTESIAN_POINT('Ctrl Pts',(22.1149403822828,-0.254945368919111,
-6.30734688179163));
#135403=CARTESIAN_POINT('Ctrl Pts',(22.0690965134344,-0.259196302886019,
-6.31039772755901));
#135404=CARTESIAN_POINT('Ctrl Pts',(22.0641721363121,-0.259652922331561,
-6.3107254380136));
#135405=CARTESIAN_POINT('Ctrl Pts',(22.0592444169884,-0.260080422701723,
-6.31105365415526));
#135406=CARTESIAN_POINT('Ctrl Pts',(22.0543137570268,-0.260478780285977,
-6.31138230273755));
#135407=CARTESIAN_POINT('Ctrl Pts',(22.0048946868554,-0.264471442842854,
-6.31467628518133));
#135408=CARTESIAN_POINT('Ctrl Pts',(21.9551747105688,-0.265534638531312,
-6.31801315904949));
#135409=CARTESIAN_POINT('Ctrl Pts',(21.905520136309,-0.263674160723438,
-6.3213342091162));
#135410=CARTESIAN_POINT('Ctrl Pts',(21.8559117159873,-0.261815412230112,
-6.32465217226612));
#135411=CARTESIAN_POINT('Ctrl Pts',(21.8063684946944,-0.257038727270444,
-6.32795404769888));
#135412=CARTESIAN_POINT('Ctrl Pts',(21.7572474127023,-0.249386952654866,
-6.33120269555329));
#135413=CARTESIAN_POINT('Ctrl Pts',(21.7081515065201,-0.241739099769335,
-6.33444967839266));
#135414=CARTESIAN_POINT('Ctrl Pts',(21.6594772769829,-0.231219180125691,
-6.3376433932741));
#135415=CARTESIAN_POINT('Ctrl Pts',(21.611573671104,-0.217904261974882,
-6.34077099162547));
#135416=CARTESIAN_POINT('Ctrl Pts',(21.5611704791935,-0.203894578100078,
-6.34406178648382));
#135417=CARTESIAN_POINT('Ctrl Pts',(21.5116205713624,-0.18679016275,-6.34727920537245));
#135418=CARTESIAN_POINT('Ctrl Pts',(21.4633212996666,-0.166721911367082,
-6.35043760878328));
#135419=CARTESIAN_POINT('Ctrl Pts',(21.4173767827947,-0.147632055932856,
-6.35344202921658));
#135420=CARTESIAN_POINT('Ctrl Pts',(21.3725640158992,-0.125860400443001,
-6.35639347018246));
#135421=CARTESIAN_POINT('Ctrl Pts',(21.3292155495703,-0.101557407831931,
-6.35932754013549));
#135422=CARTESIAN_POINT('Ctrl Pts',(21.2858407634226,-0.0772396592117836,
-6.36226339156306));
#135423=CARTESIAN_POINT('Ctrl Pts',(21.243932377574,-0.0503871474844555,
-6.36518226420441));
#135424=CARTESIAN_POINT('Ctrl Pts',(21.2038107755342,-0.0211918718241275,
-6.36813788253618));
#135425=CARTESIAN_POINT('Ctrl Pts',(21.1667726819221,0.00575962806526852,
-6.37086634956861));
#135426=CARTESIAN_POINT('Ctrl Pts',(21.1312570442013,0.0347080777191685,
-6.37362671885412));
#135427=CARTESIAN_POINT('Ctrl Pts',(21.0975026667503,0.0654651437902246,
-6.37646898484549));
#135428=CARTESIAN_POINT('Ctrl Pts',(21.0946320745128,0.0680808340140638,
-6.37671070124815));
#135429=CARTESIAN_POINT('Ctrl Pts',(21.0917741894305,0.0707096087900683,
-6.37695300996106));
#135430=CARTESIAN_POINT('Ctrl Pts',(21.0889291411323,0.0733513549243375,
-6.37719594173426));
#135431=CARTESIAN_POINT('Ctrl Pts',(21.0834768458455,0.0784140387480052,
-6.37766150000366));
#135432=CARTESIAN_POINT('Ctrl Pts',(21.0780717819019,0.083524250400563,
-6.37812935236638));
#135433=CARTESIAN_POINT('Ctrl Pts',(21.0727149191585,0.088681075410001,
-6.37859971721835));
#135434=CARTESIAN_POINT('Ctrl Pts',(21.0727027152255,0.0886928236197154,
-6.37860078879726));
#135435=CARTESIAN_POINT('Ctrl Pts',(21.0726905115426,0.0887045720713643,
-6.37860186038921));
#135436=CARTESIAN_POINT('Ctrl Pts',(21.0726783081099,0.088716320764919,
-6.3786029319942));
#135437=CARTESIAN_POINT('Ctrl Pts',(21.0400053868558,0.120171743909859,
-6.38147199895402));
#135438=CARTESIAN_POINT('Ctrl Pts',(21.0090029359217,0.15349050789987,-6.38444249757833));
#135439=CARTESIAN_POINT('Ctrl Pts',(20.9798665486039,0.188451002708149,
-6.387456984648));
#135440=CARTESIAN_POINT('Ctrl Pts',(20.9776674710995,0.191089656458805,
-6.38768450395676));
#135441=CARTESIAN_POINT('Ctrl Pts',(20.9754790263654,0.193737637925406,
-6.3879122738466));
#135442=CARTESIAN_POINT('Ctrl Pts',(20.9733012995092,0.196394839864987,
-6.38814026962001));
#135443=CARTESIAN_POINT('Ctrl Pts',(20.9423131839197,0.234205679463701,
-6.39138455131693));
#135444=CARTESIAN_POINT('Ctrl Pts',(20.913494205518,0.273888825683377,-6.3946739912619));
#135445=CARTESIAN_POINT('Ctrl Pts',(20.887045626256,0.315148386127671,-6.39795100572697));
#135446=CARTESIAN_POINT('Ctrl Pts',(20.8606219175173,0.356369148765442,
-6.40122493870083));
#135447=CARTESIAN_POINT('Ctrl Pts',(20.8365638887051,0.399163211076456,
-6.40448617352742));
#135448=CARTESIAN_POINT('Ctrl Pts',(20.815036381223,0.443220424278687,-6.40769730950366));
#135449=CARTESIAN_POINT('Ctrl Pts',(20.79350913539,0.487277102001824,-6.41090840645119));
#135450=CARTESIAN_POINT('Ctrl Pts',(20.7745122829039,0.532596833091644,
-6.41406930190269));
#135451=CARTESIAN_POINT('Ctrl Pts',(20.7581772244235,0.578855915145535,
-6.41716555815408));
#135452=CARTESIAN_POINT('Ctrl Pts',(20.7418437351398,0.625110553407703,
-6.42026151696944));
#135453=CARTESIAN_POINT('Ctrl Pts',(20.7281716171061,0.672304312036179,
-6.42329289035936));
#135454=CARTESIAN_POINT('Ctrl Pts',(20.7172586082588,0.720100864105695,
-6.42626864486285));
#135455=CARTESIAN_POINT('Ctrl Pts',(20.7063314001507,0.767959605779906,
-6.42924827121457));
#135456=CARTESIAN_POINT('Ctrl Pts',(20.6981707252607,0.816422655751023,
-6.43217231323709));
#135457=CARTESIAN_POINT('Ctrl Pts',(20.6928385219224,0.86514038307293,-6.43507160755436));
#135458=CARTESIAN_POINT('Ctrl Pts',(20.6878983206692,0.91027657955696,-6.43775775744604));
#135459=CARTESIAN_POINT('Ctrl Pts',(20.6853858878954,0.955631193610204,
-6.44042312323611));
#135460=CARTESIAN_POINT('Ctrl Pts',(20.6853192846385,1.00091784626045,-6.44310594448226));
#135461=CARTESIAN_POINT('Ctrl Pts',(20.6853192846374,1.00091784701293,-6.44310594452685));
#135462=CARTESIAN_POINT('Ctrl Pts',(20.6852476706139,1.04961157282125,-6.44599060379221));
#135463=CARTESIAN_POINT('Ctrl Pts',(20.6880029641633,1.09822147251094,-6.44889478139007));
#135464=CARTESIAN_POINT('Ctrl Pts',(20.693576975525,1.14645852421811,-6.45188204245391));
#135465=CARTESIAN_POINT('Ctrl Pts',(20.6959637507833,1.16711348777554,-6.45316117884858));
#135466=CARTESIAN_POINT('Ctrl Pts',(20.6988674365921,1.18770073386852,-6.45445554882266));
#135467=CARTESIAN_POINT('Ctrl Pts',(20.7022881168209,1.20820041042418,-6.45577014294436));
#135468=CARTESIAN_POINT('Ctrl Pts',(20.7022909071302,1.20821713237236,-6.455771215282));
#135469=CARTESIAN_POINT('Ctrl Pts',(20.7022936977835,1.20823385426237,-6.45577228763309));
#135470=CARTESIAN_POINT('Ctrl Pts',(20.7022964887809,1.20825057609418,-6.45577335999765));
#135471=CARTESIAN_POINT('Ctrl Pts',(20.7098513922171,1.25351461943438,-6.45867612545473));
#135472=CARTESIAN_POINT('Ctrl Pts',(20.719943901946,1.29843270002029,-6.46168198209947));
#135473=CARTESIAN_POINT('Ctrl Pts',(20.7324967565363,1.34271492383747,-6.46473183056348));
#135474=CARTESIAN_POINT('Ctrl Pts',(20.7338491123666,1.34748557764594,-6.46506039968074));
#135475=CARTESIAN_POINT('Ctrl Pts',(20.7352299875163,1.35224881741516,-6.46538947938398));
#135476=CARTESIAN_POINT('Ctrl Pts',(20.7366392583893,1.3570042568621,-6.46571899577594));
#135477=CARTESIAN_POINT('Ctrl Pts',(20.7507252931146,1.40453613058896,-6.46901259917654));
#135478=CARTESIAN_POINT('Ctrl Pts',(20.7676519490923,1.45129316637296,-6.47234927943961));
#135479=CARTESIAN_POINT('Ctrl Pts',(20.7872818407009,1.4969357915126,-6.47567026653761));
#135480=CARTESIAN_POINT('Ctrl Pts',(20.8068934362007,1.54253587528487,-6.47898815829804));
#135481=CARTESIAN_POINT('Ctrl Pts',(20.8292029756259,1.58702381075725,-6.48229009245401));
#135482=CARTESIAN_POINT('Ctrl Pts',(20.8540418840448,1.63008212614013,-6.48553887032211));
#135483=CARTESIAN_POINT('Ctrl Pts',(20.8788680045907,1.67311827371008,-6.48878597561432));
#135484=CARTESIAN_POINT('Ctrl Pts',(20.9062208296114,1.71472632860985,-6.49197988416206));
#135485=CARTESIAN_POINT('Ctrl Pts',(20.9359027452407,1.75460861385274,-6.49510768867772));
#135486=CARTESIAN_POINT('Ctrl Pts',(20.9671387033798,1.79657899770192,-6.49839925422688));
#135487=CARTESIAN_POINT('Ctrl Pts',(21.0009543832482,1.83663788006493,-6.5016174317813));
#135488=CARTESIAN_POINT('Ctrl Pts',(21.0370843899636,1.87446167891545,-6.50477652742008));
#135489=CARTESIAN_POINT('Ctrl Pts',(21.0714470076843,1.91043523272293,-6.50778108805117));
#135490=CARTESIAN_POINT('Ctrl Pts',(21.107902955075,1.94438697496761,-6.51073262798619));
#135491=CARTESIAN_POINT('Ctrl Pts',(21.146192076393,1.97606098262062,-6.51366671243432));
#135492=CARTESIAN_POINT('Ctrl Pts',(21.1845043966793,2.00775418121552,-6.51660257461279));
#135493=CARTESIAN_POINT('Ctrl Pts',(21.2246523245406,2.03716645867982,-6.51952137292581));
#135494=CARTESIAN_POINT('Ctrl Pts',(21.266341359226,2.06406820693224,-6.52247680275527));
#135495=CARTESIAN_POINT('Ctrl Pts',(21.3048348640832,2.08890789403071,-6.52520569425767));
#135496=CARTESIAN_POINT('Ctrl Pts',(21.344642779175,2.11160723173152,-6.52796640405794));
#135497=CARTESIAN_POINT('Ctrl Pts',(21.3855032537724,2.13201127186824,-6.53080895545953));
#135498=CARTESIAN_POINT('Ctrl Pts',(21.388968410253,2.13374162846853,-6.53105001691336));
#135499=CARTESIAN_POINT('Ctrl Pts',(21.3924411512998,2.13545550504126,-6.53129166695737));
#135500=CARTESIAN_POINT('Ctrl Pts',(21.3959213258287,2.13715282208749,-6.53153393610074));
#135501=CARTESIAN_POINT('Ctrl Pts',(21.4026324497046,2.14042590648584,-6.53200112480608));
#135502=CARTESIAN_POINT('Ctrl Pts',(21.4093710802883,2.14363737076525,-6.53247062165335));
#135503=CARTESIAN_POINT('Ctrl Pts',(21.4161360021069,2.14678663364116,-6.53294264747405));
#135504=CARTESIAN_POINT('Ctrl Pts',(21.4161513468401,2.14679377704944,-6.53294371816052));
#135505=CARTESIAN_POINT('Ctrl Pts',(21.4161666917085,2.14680092013772,-6.53294478886));
#135506=CARTESIAN_POINT('Ctrl Pts',(21.4161820367122,2.14680806290598,-6.5329458595725));
#135507=CARTESIAN_POINT('Ctrl Pts',(21.4577876250457,2.16617456689952,-6.53584892979829));
#135508=CARTESIAN_POINT('Ctrl Pts',(21.5005429917933,2.18325238011408,-6.53885504780126));
#135509=CARTESIAN_POINT('Ctrl Pts',(21.5441653242742,2.19794127035611,-6.54190510997097));
#135510=CARTESIAN_POINT('Ctrl Pts',(21.5488627923362,2.1995230425552,-6.54223355571915));
#135511=CARTESIAN_POINT('Ctrl Pts',(21.5535702651596,2.2010771234395,-6.54256251104589));
#135512=CARTESIAN_POINT('Ctrl Pts',(21.5582873547441,2.20260339662812,-6.54289190214734));
#135513=CARTESIAN_POINT('Ctrl Pts',(21.6054538032502,2.21786468952239,-6.54618550260735));
#135514=CARTESIAN_POINT('Ctrl Pts',(21.6535875340928,2.23034517524371,-6.54952212201841));
#135515=CARTESIAN_POINT('Ctrl Pts',(21.7023308204948,2.23996612765215,-6.55284300448456));
#135516=CARTESIAN_POINT('Ctrl Pts',(21.7510286760591,2.2495781129195,-6.55616079174554));
#135517=CARTESIAN_POINT('Ctrl Pts',(21.8003349605609,2.25633620796331,-6.55946257787524));
#135518=CARTESIAN_POINT('Ctrl Pts',(21.8498925316008,2.26019990474393,-6.56271117944452));
#135519=CARTESIAN_POINT('Ctrl Pts',(21.8994245922865,2.26406161264029,-6.56595810875717));
#135520=CARTESIAN_POINT('Ctrl Pts',(21.9492076923783,2.26503198288817,-6.56915181316977));
#135521=CARTESIAN_POINT('Ctrl Pts',(21.9988845893612,2.26310565079043,-6.57227939982553));
#135522=CARTESIAN_POINT('Ctrl Pts',(22.0511644406077,2.2610783833555,-6.57557086477311));
#135523=CARTESIAN_POINT('Ctrl Pts',(22.1033266316716,2.25584243778223,-6.57878892069119));
#135524=CARTESIAN_POINT('Ctrl Pts',(22.1549541755633,2.2474337071581,-6.58194789038805));
#135525=CARTESIAN_POINT('Ctrl Pts',(22.2040543373295,2.23943661872874,-6.58495221543314));
#135526=CARTESIAN_POINT('Ctrl Pts',(22.2526708125535,2.22856984937452,-6.58790352022602));
#135527=CARTESIAN_POINT('Ctrl Pts',(22.3004454236137,2.21490323255278,-6.59083738040785));
#135528=CARTESIAN_POINT('Ctrl Pts',(22.3482489917486,2.201228332142,-6.59377301885657));
#135529=CARTESIAN_POINT('Ctrl Pts',(22.3952094434081,2.18474977396774,-6.59669160440083));
#135530=CARTESIAN_POINT('Ctrl Pts',(22.4409708823338,2.16558060137129,-6.59964683883878));
#135531=CARTESIAN_POINT('Ctrl Pts',(22.4832230133281,2.14788145530833,-6.60237544518339));
#135532=CARTESIAN_POINT('Ctrl Pts',(22.5244533118351,2.12788815848536,-6.60513588226684));
#135533=CARTESIAN_POINT('Ctrl Pts',(22.5643859502812,2.10572903376187,-6.60797816851481));
#135534=CARTESIAN_POINT('Ctrl Pts',(22.5677741073003,2.10384890269889,-6.60821932743834));
#135535=CARTESIAN_POINT('Ctrl Pts',(22.5711529534085,2.10195318318941,-6.60846107559247));
#135536=CARTESIAN_POINT('Ctrl Pts',(22.5745223374019,2.10004195499564,-6.608703443529));
#135537=CARTESIAN_POINT('Ctrl Pts',(22.5810220036043,2.09635512520112,-6.60917098023264));
#135538=CARTESIAN_POINT('Ctrl Pts',(22.5874863489624,2.09261067408924,-6.60964082917019));
#135539=CARTESIAN_POINT('Ctrl Pts',(22.5939142039863,2.08880927703164,-6.61011321169221));
#135540=CARTESIAN_POINT('Ctrl Pts',(22.5939287831095,2.08880065502077,-6.61011428311074));
#135541=CARTESIAN_POINT('Ctrl Pts',(22.593943362045,2.08879203271695,-6.6101153545423));
#135542=CARTESIAN_POINT('Ctrl Pts',(22.5939579407927,2.0887834101202,-6.6101164259869));
#135543=CARTESIAN_POINT('Ctrl Pts',(22.6334564898289,2.06542200309203,-6.61301931639274));
#135544=CARTESIAN_POINT('Ctrl Pts',(22.6717177856026,2.03981823663042,-6.61602527589385));
#135545=CARTESIAN_POINT('Ctrl Pts',(22.7084992502895,2.01214865355727,-6.61907519982099));
#135546=CARTESIAN_POINT('Ctrl Pts',(22.7124618255038,2.00916772810996,-6.61940377708299));
#135547=CARTESIAN_POINT('Ctrl Pts',(22.7164072065831,2.00616287220831,-6.61973286461307));
#135548=CARTESIAN_POINT('Ctrl Pts',(22.7203350777303,2.00313434035199,-6.62006238850735));
#135549=CARTESIAN_POINT('Ctrl Pts',(22.7595934208316,1.97286472654529,-6.62335591867085));
#135550=CARTESIAN_POINT('Ctrl Pts',(22.7971053959507,1.94022488047618,-6.62669248968518));
#135551=CARTESIAN_POINT('Ctrl Pts',(22.8326037837931,1.90546530295001,-6.63001333856003));
#135552=CARTESIAN_POINT('Ctrl Pts',(22.8680690690358,1.87073813907568,-6.63333109071027));
#135553=CARTESIAN_POINT('Ctrl Pts',(22.9015247857167,1.83389536597084,-6.63663285649171));
#135554=CARTESIAN_POINT('Ctrl Pts',(22.9327355656196,1.79520861528196,-6.63988144488369));
#135555=CARTESIAN_POINT('Ctrl Pts',(22.9639302666225,1.75654179489907,-6.64312835969597));
#135556=CARTESIAN_POINT('Ctrl Pts',(22.9928824170569,1.71603293301656,-6.64632205678973));
#135557=CARTESIAN_POINT('Ctrl Pts',(23.0193855766467,1.67397361748084,-6.64944963556714));
#135558=CARTESIAN_POINT('Ctrl Pts',(23.0472785290064,1.62970876367932,-6.65274122069094));
#135559=CARTESIAN_POINT('Ctrl Pts',(23.0724585106709,1.58372635331601,-6.6559593902003));
#135560=CARTESIAN_POINT('Ctrl Pts',(23.0947193002865,1.53639062033585,-6.65911846042949));
#135561=CARTESIAN_POINT('Ctrl Pts',(23.1158894916827,1.49137395451329,-6.66212276182855));
#135562=CARTESIAN_POINT('Ctrl Pts',(23.1344195132852,1.44513344505979,-6.66507403553562));
#135563=CARTESIAN_POINT('Ctrl Pts',(23.150164416456,1.39800397460386,-6.66800785145195));
#135564=CARTESIAN_POINT('Ctrl Pts',(23.1659188599464,1.35084594695641,-6.67094344505731));
#135565=CARTESIAN_POINT('Ctrl Pts',(23.1788843355623,1.30279783682696,-6.67386197248567));
#135566=CARTESIAN_POINT('Ctrl Pts',(23.1889528208304,1.25421707858004,-6.67681713154628));
#135567=CARTESIAN_POINT('Ctrl Pts',(23.198249482924,1.20936039143749,-6.67954575601039));
#135568=CARTESIAN_POINT('Ctrl Pts',(23.2050761545052,1.1640490966972,-6.68230619844614));
#135569=CARTESIAN_POINT('Ctrl Pts',(23.2093826866129,1.11858326311822,-6.68514848154152));
#135570=CARTESIAN_POINT('Ctrl Pts',(23.2097479316627,1.11472722066174,-6.68538954089151));
#135571=CARTESIAN_POINT('Ctrl Pts',(23.210095069409,1.11087004298659,-6.68563118892575));
#135572=CARTESIAN_POINT('Ctrl Pts',(23.2104240801512,1.1070118997018,-6.6858734561609));
#135573=CARTESIAN_POINT('Ctrl Pts',(23.211059522753,1.09956038431777,-6.68634136465898));
#135574=CARTESIAN_POINT('Ctrl Pts',(23.2116273591245,1.09210540896253,-6.68681158883039));
#135575=CARTESIAN_POINT('Ctrl Pts',(23.2121274846818,1.08464832339169,-6.68728435058385));
#135576=CARTESIAN_POINT('Ctrl Pts',(23.2121286181064,1.08463142354659,-6.68728542199443));
#135577=CARTESIAN_POINT('Ctrl Pts',(23.2121297511833,1.08461452369063,-6.68728649341805));
#135578=CARTESIAN_POINT('Ctrl Pts',(23.2121308839124,1.08459762382385,-6.6872875648547));
#135579=CARTESIAN_POINT('Ctrl Pts',(23.2151998645702,1.03880965703489,-6.69019048157388));
#135580=CARTESIAN_POINT('Ctrl Pts',(23.2157197162104,0.992774095079383,
-6.69319646598462));
#135581=CARTESIAN_POINT('Ctrl Pts',(23.2136988736089,0.946790846383176,
-6.69624641501267));
#135582=CARTESIAN_POINT('Ctrl Pts',(23.2134811925711,0.941837624747483,
-6.69657494929291));
#135583=CARTESIAN_POINT('Ctrl Pts',(23.2132340590177,0.936885051607219,
-6.69690399370157));
#135584=CARTESIAN_POINT('Ctrl Pts',(23.2129575042627,0.931933531175082,
-6.69723347436758));
#135585=CARTESIAN_POINT('Ctrl Pts',(23.2101929952465,0.882436921082219,
-6.70052704374327));
#135586=CARTESIAN_POINT('Ctrl Pts',(23.2044859647048,0.833040306351522,
-6.70386365569681));
#135587=CARTESIAN_POINT('Ctrl Pts',(23.1958919117608,0.784105745232262,
-6.70718454778575));
#135588=CARTESIAN_POINT('Ctrl Pts',(23.1873058706464,0.73521680349227,-6.7105023439639));
#135589=CARTESIAN_POINT('Ctrl Pts',(23.1758384782386,0.686788932139672,
-6.71380415601139));
#135590=CARTESIAN_POINT('Ctrl Pts',(23.1615806728929,0.639169867944375,
-6.71705279346231));
#135591=CARTESIAN_POINT('Ctrl Pts',(23.1473302097475,0.591575325664848,
-6.72029975799473));
#135592=CARTESIAN_POINT('Ctrl Pts',(23.1302922787626,0.54478871760092,-6.72349350756752));
#135593=CARTESIAN_POINT('Ctrl Pts',(23.1105906354368,0.499145206274198,
-6.72662114241718));
#135594=CARTESIAN_POINT('Ctrl Pts',(23.0898564998218,0.451109682630735,
-6.72991268536387));
#135595=CARTESIAN_POINT('Ctrl Pts',(23.0661717270767,0.40434040629928,-6.73313082134135));
#135596=CARTESIAN_POINT('Ctrl Pts',(23.0397200949546,0.359213406650139,
-6.73628986628034));
#135597=CARTESIAN_POINT('Ctrl Pts',(23.0145635988948,0.316295934351077,
-6.73929423671743));
#135598=CARTESIAN_POINT('Ctrl Pts',(22.9869046538028,0.274863929787187,
-6.74224558348198));
#135599=CARTESIAN_POINT('Ctrl Pts',(22.9569374945045,0.235226323224293,
-6.74517947716699));
#135600=CARTESIAN_POINT('Ctrl Pts',(22.9269521756465,0.195564696984603,
-6.74811514873881));
#135601=CARTESIAN_POINT('Ctrl Pts',(22.8946555404327,0.157700009658192,
-6.75103375887565));
#135602=CARTESIAN_POINT('Ctrl Pts',(22.8602813054491,0.121923489755126,
-6.75398900607447));
#135603=CARTESIAN_POINT('Ctrl Pts',(22.8285423804401,0.088889786377389,
-6.75671768845158));
#135604=CARTESIAN_POINT('Ctrl Pts',(22.795031725813,0.0576361706875381,
-6.75947819291928));
#135605=CARTESIAN_POINT('Ctrl Pts',(22.7599684665536,0.0283736927536179,
-6.76232054099184));
#135606=CARTESIAN_POINT('Ctrl Pts',(22.7569943620507,0.0258916169504828,
-6.76256163210487));
#135607=CARTESIAN_POINT('Ctrl Pts',(22.7540090790911,0.0234238366124944,
-6.76280331205156));
#135608=CARTESIAN_POINT('Ctrl Pts',(22.7510127464627,0.0209704639387167,
-6.76304561135783));
#135609=CARTESIAN_POINT('Ctrl Pts',(22.7452300253659,0.0162356191540649,
-6.76351323277503));
#135610=CARTESIAN_POINT('Ctrl Pts',(22.7394062714582,0.0115545087102523,
-6.76398316700287));
#135611=CARTESIAN_POINT('Ctrl Pts',(22.7335425367983,0.0069279805368398,
-6.76445563551957));
#135612=CARTESIAN_POINT('Ctrl Pts',(22.7335292417718,0.00691749066676322,
-6.76445670676202));
#135613=CARTESIAN_POINT('Ctrl Pts',(22.7335159465398,0.00690700107725976,
-6.76445777801749));
#135614=CARTESIAN_POINT('Ctrl Pts',(22.7335026511022,0.00689651176833514,
-6.76445884928599));
#135615=CARTESIAN_POINT('Ctrl Pts',(22.6975191189874,-0.0214923534050475,
-6.76735819159388));
#135616=CARTESIAN_POINT('Ctrl Pts',(22.6598937213588,-0.0479238910441021,
-6.77036038496798));
#135617=CARTESIAN_POINT('Ctrl Pts',(22.6208782113788,-0.0722355422069828,
-6.77340642694032));
#135618=CARTESIAN_POINT('Ctrl Pts',(22.6177634576589,-0.0741764320207257,
-6.77364960383508));
#135619=CARTESIAN_POINT('Ctrl Pts',(22.6146398716569,-0.0761038106475597,
-6.77389306019558));
#135620=CARTESIAN_POINT('Ctrl Pts',(22.6115075957382,-0.0780175956295496,
-6.77413676600051));
#135621=CARTESIAN_POINT('Ctrl Pts',(22.5692067673493,-0.103862920944605,
-6.77742796948936));
#135622=CARTESIAN_POINT('Ctrl Pts',(22.5253155148886,-0.127229590285433,
-6.78076406660601));
#135623=CARTESIAN_POINT('Ctrl Pts',(22.4801635910675,-0.147957541694851,
-6.78408577953313));
#135624=CARTESIAN_POINT('Ctrl Pts',(22.4507965966687,-0.16143908536842,
-6.78624623509449));
#135625=CARTESIAN_POINT('Ctrl Pts',(22.4208965137197,-0.173805229005387,
-6.78840095258332));
#135626=CARTESIAN_POINT('Ctrl Pts',(22.3905561784951,-0.185020462416371,
-6.79053837538029));
#135627=CARTESIAN_POINT('Ctrl Pts',(22.3906127229569,-0.185251306619802,
-6.65225448505536));
#135628=CARTESIAN_POINT('Ctrl Pts',(22.4229418914661,-0.173233059039878,
-6.65012827817395));
#135629=CARTESIAN_POINT('Ctrl Pts',(22.4547681000435,-0.159896281965281,
-6.64804342440638));
#135630=CARTESIAN_POINT('Ctrl Pts',(22.5249542668526,-0.127047699454832,
-6.64343073834645));
#135631=CARTESIAN_POINT('Ctrl Pts',(22.562943450965,-0.106846685042448,
-6.64092390595764));
#135632=CARTESIAN_POINT('Ctrl Pts',(22.6682338942969,-0.043771221167721,
-6.63382131291894));
#135633=CARTESIAN_POINT('Ctrl Pts',(22.7326014297101,0.00358078292254316,
-6.62929400300919));
#135634=CARTESIAN_POINT('Ctrl Pts',(22.810506713512,0.0731242077139838,
-6.62303729769182));
#135635=CARTESIAN_POINT('Ctrl Pts',(22.8284492585354,0.0901114018485893,
-6.62153374253444));
#135636=CARTESIAN_POINT('Ctrl Pts',(22.8573897587429,0.119165192594868,
-6.61897932643687));
#135637=CARTESIAN_POINT('Ctrl Pts',(22.8686716815253,0.130938202508655,
-6.61794774962455));
#135638=CARTESIAN_POINT('Ctrl Pts',(22.8963653551783,0.160979326106974,
-6.61532267287721));
#135639=CARTESIAN_POINT('Ctrl Pts',(22.9124770022823,0.179511779669976,
-6.61371169143372));
#135640=CARTESIAN_POINT('Ctrl Pts',(22.9489990013632,0.224078087098607,
-6.60987908201856));
#135641=CARTESIAN_POINT('Ctrl Pts',(22.9689477287969,0.250467396070868,
-6.60764112847349));
#135642=CARTESIAN_POINT('Ctrl Pts',(23.049927730056,0.366808645854362,-6.59799017465999));
#135643=CARTESIAN_POINT('Ctrl Pts',(23.1002705280125,0.463662450552342,
-6.59053615369726));
#135644=CARTESIAN_POINT('Ctrl Pts',(23.1478751937892,0.593860023580723,
-6.58156746065694));
#135645=CARTESIAN_POINT('Ctrl Pts',(23.1571462844445,0.622306021973822,
-6.579663061484));
#135646=CARTESIAN_POINT('Ctrl Pts',(23.173616779965,0.679674107861699,-6.57592415435642));
#135647=CARTESIAN_POINT('Ctrl Pts',(23.1808202093669,0.708575003392693,
-6.57409055540309));
#135648=CARTESIAN_POINT('Ctrl Pts',(23.1991670030157,0.795099497046015,
-6.56872598676445));
#135649=CARTESIAN_POINT('Ctrl Pts',(23.2073284953621,0.853274167238784,
-6.56528446753947));
#135650=CARTESIAN_POINT('Ctrl Pts',(23.2172708468426,0.99548442344696,-6.55702394678011));
#135651=CARTESIAN_POINT('Ctrl Pts',(23.2147802828762,1.07952552150498,-6.5522740699562));
#135652=CARTESIAN_POINT('Ctrl Pts',(23.2008467656394,1.18692093023769,-6.54578160592033));
#135653=CARTESIAN_POINT('Ctrl Pts',(23.1970021781084,1.21105084973372,-6.5442938038775));
#135654=CARTESIAN_POINT('Ctrl Pts',(23.189430441389,1.25107421682301,-6.54175542394405));
#135655=CARTESIAN_POINT('Ctrl Pts',(23.1860903008329,1.26703329452856,-6.5407233980417));
#135656=CARTESIAN_POINT('Ctrl Pts',(23.1768890529206,1.30711479257385,-6.53808015883207));
#135657=CARTESIAN_POINT('Ctrl Pts',(23.1706250219677,1.33113534840014,-6.5364507715613));
#135658=CARTESIAN_POINT('Ctrl Pts',(23.1542184221563,1.38723277235453,-6.53256099081813));
#135659=CARTESIAN_POINT('Ctrl Pts',(23.1434945033475,1.41912035655433,-6.53028367481263));
#135660=CARTESIAN_POINT('Ctrl Pts',(23.0932344276081,1.55092402255907,-6.52067607673287));
#135661=CARTESIAN_POINT('Ctrl Pts',(23.0423104011212,1.64604017452173,-6.51331219644281));
#135662=CARTESIAN_POINT('Ctrl Pts',(22.9625696372737,1.75799863612506,-6.50441697182777));
#135663=CARTESIAN_POINT('Ctrl Pts',(22.9443112688797,1.78179571422997,-6.50250723217336));
#135664=CARTESIAN_POINT('Ctrl Pts',(22.9062836969719,1.8278688999728,-6.49876402185259));
#135665=CARTESIAN_POINT('Ctrl Pts',(22.8865396142467,1.85014068913675,-6.49693125825614));
#135666=CARTESIAN_POINT('Ctrl Pts',(22.8259593021182,1.91380182455314,-6.49159971436625));
#135667=CARTESIAN_POINT('Ctrl Pts',(22.7830343684834,1.95309663528567,-6.48818815045933));
#135668=CARTESIAN_POINT('Ctrl Pts',(22.6744986427988,2.03949877468062,-6.48014601181487));
#135669=CARTESIAN_POINT('Ctrl Pts',(22.6067931185085,2.08354831775119,-6.47557668954084));
#135670=CARTESIAN_POINT('Ctrl Pts',(22.5117677518244,2.13317508698441,-6.46918173980384));
#135671=CARTESIAN_POINT('Ctrl Pts',(22.4877914023894,2.14474843587869,-6.46756850683698));
#135672=CARTESIAN_POINT('Ctrl Pts',(22.44848385361,2.16221469264991,-6.46489678218574));
#135673=CARTESIAN_POINT('Ctrl Pts',(22.4333723103359,2.16858046688527,-6.46386270623205));
#135674=CARTESIAN_POINT('Ctrl Pts',(22.3966486341831,2.18321615882464,-6.46132958118678));
#135675=CARTESIAN_POINT('Ctrl Pts',(22.3749275231949,2.19118929205379,-6.4598168478667));
#135676=CARTESIAN_POINT('Ctrl Pts',(22.3244422896744,2.20816433163066,-6.45628627200453));
#135677=CARTESIAN_POINT('Ctrl Pts',(22.2955503129036,2.21674273094702,-6.45425524132634));
#135678=CARTESIAN_POINT('Ctrl Pts',(22.1694415427855,2.24933203011163,-6.4454114212588));
#135679=CARTESIAN_POINT('Ctrl Pts',(22.0698531090616,2.26278477941171,-6.43851841280116));
#135680=CARTESIAN_POINT('Ctrl Pts',(21.9357225270067,2.264876368253,-6.42972147512304));
#135681=CARTESIAN_POINT('Ctrl Pts',(21.9017195179265,2.2640353659169,-6.4275288580805));
#135682=CARTESIAN_POINT('Ctrl Pts',(21.8395584929326,2.25998542815719,-6.4235844331879));
#135683=CARTESIAN_POINT('Ctrl Pts',(21.8113960304349,2.25719916417087,-6.42182145704969));
#135684=CARTESIAN_POINT('Ctrl Pts',(21.743574011528,2.24818211048376,-6.4176216835447));
#135685=CARTESIAN_POINT('Ctrl Pts',(21.7040710336316,2.2410034873884,-6.41521436637669));
#135686=CARTESIAN_POINT('Ctrl Pts',(21.5560739308449,2.20676277512529,-6.40624580782625));
#135687=CARTESIAN_POINT('Ctrl Pts',(21.4510083410748,2.16724351259546,-6.40002393137641));
#135688=CARTESIAN_POINT('Ctrl Pts',(21.3299869840087,2.10235993287699,-6.39181347945772));
#135689=CARTESIAN_POINT('Ctrl Pts',(21.307833745662,2.08960353908267,-6.3902609318516));
#135690=CARTESIAN_POINT('Ctrl Pts',(21.2722277399349,2.06763762816172,-6.3876583929243));
#135691=CARTESIAN_POINT('Ctrl Pts',(21.2585401188699,2.05882412293911,-6.38663011554596));
#135692=CARTESIAN_POINT('Ctrl Pts',(21.2254481470396,2.03660070931656,-6.38407229850616));
#135693=CARTESIAN_POINT('Ctrl Pts',(21.2062436324016,2.02290895194047,-6.38252763448191));
#135694=CARTESIAN_POINT('Ctrl Pts',(21.1626349070214,1.98994091823309,-6.37889727310592));
#135695=CARTESIAN_POINT('Ctrl Pts',(21.1385363406133,1.97028518491145,-6.37679723784216));
#135696=CARTESIAN_POINT('Ctrl Pts',(21.0493634331188,1.89190494460368,-6.36872172455945));
#135697=CARTESIAN_POINT('Ctrl Pts',(20.9897243191032,1.82735369292184,-6.36268736375753));
#135698=CARTESIAN_POINT('Ctrl Pts',(20.9141747344568,1.72629889302598,-6.35432593481205));
#135699=CARTESIAN_POINT('Ctrl Pts',(20.892530192544,1.69440776998183,-6.35181739378952));
#135700=CARTESIAN_POINT('Ctrl Pts',(20.85771431513,1.63769691624951,-6.34757219712827));
#135701=CARTESIAN_POINT('Ctrl Pts',(20.8438517915657,1.61333653622235,-6.34581255880034));
#135702=CARTESIAN_POINT('Ctrl Pts',(20.8147824893943,1.55805665696229,-6.34194964543567));
#135703=CARTESIAN_POINT('Ctrl Pts',(20.8000064289279,1.52693559631412,-6.33986172053459));
#135704=CARTESIAN_POINT('Ctrl Pts',(20.7707062881251,1.45810102891156,-6.33539696595839));
#135705=CARTESIAN_POINT('Ctrl Pts',(20.756681700617,1.4202165588794,-6.33303522280747));
#135706=CARTESIAN_POINT('Ctrl Pts',(20.7204004420713,1.30563828213752,-6.32606691087302));
#135707=CARTESIAN_POINT('Ctrl Pts',(20.7035668400059,1.22744791854381,-6.32154485298269));
#135708=CARTESIAN_POINT('Ctrl Pts',(20.690949349893,1.12053172370471,-6.31514163156302));
#135709=CARTESIAN_POINT('Ctrl Pts',(20.6885997400898,1.0927662796998,-6.31345795749804));
#135710=CARTESIAN_POINT('Ctrl Pts',(20.6863252941211,1.04854268290466,-6.31071233581132));
#135711=CARTESIAN_POINT('Ctrl Pts',(20.6858013954468,1.03212484759911,-6.30967847347548));
#135712=CARTESIAN_POINT('Ctrl Pts',(20.6853222615321,0.993537912993814,
-6.30720972031712));
#135713=CARTESIAN_POINT('Ctrl Pts',(20.6856298223234,0.971373844165684,
-6.30576351673096));
#135714=CARTESIAN_POINT('Ctrl Pts',(20.6894531847861,0.876222513690097,
-6.29946400872126));
#135715=CARTESIAN_POINT('Ctrl Pts',(20.6987090850081,0.803609462986055,
-6.29443513129044));
#135716=CARTESIAN_POINT('Ctrl Pts',(20.7292486581001,0.662675292926393,
-6.28460518109254));
#135717=CARTESIAN_POINT('Ctrl Pts',(20.7501582003088,0.594532485565407,
-6.2798197683935));
#135718=CARTESIAN_POINT('Ctrl Pts',(20.7881329708965,0.500033280715777,
-6.27321078514778));
#135719=CARTESIAN_POINT('Ctrl Pts',(20.800606706807,0.471987669378895,-6.27125137703142));
#135720=CARTESIAN_POINT('Ctrl Pts',(20.8270225246117,0.417979067579286,
-6.26747542497142));
#135721=CARTESIAN_POINT('Ctrl Pts',(20.8408757780864,0.391994699817149,
-6.26565746122949));
#135722=CARTESIAN_POINT('Ctrl Pts',(20.8821316750368,0.320723060396655,
-6.26064793415078));
#135723=CARTESIAN_POINT('Ctrl Pts',(20.9114885204447,0.276636580457099,
-6.25752406661893));
#135724=CARTESIAN_POINT('Ctrl Pts',(21.0028151189924,0.156558306110455,
-6.24874156481803));
#135725=CARTESIAN_POINT('Ctrl Pts',(21.0709557507471,0.0857624279732416,
-6.24323398612785));
#135726=CARTESIAN_POINT('Ctrl Pts',(21.1631953468981,0.00986762333587077,
-6.23600949412291));
#135727=CARTESIAN_POINT('Ctrl Pts',(21.1801639077479,-0.00338225527553693,
-6.23468766683016));
#135728=CARTESIAN_POINT('Ctrl Pts',(21.211099032642,-0.0262912028573803,
-6.23227438584376));
#135729=CARTESIAN_POINT('Ctrl Pts',(21.2249369620469,-0.036113769134416,
-6.23119260707361));
#135730=CARTESIAN_POINT('Ctrl Pts',(21.2648901438327,-0.0632814662434411,
-6.22806889240433));
#135731=CARTESIAN_POINT('Ctrl Pts',(21.2914575813583,-0.0799372974997237,
-6.22599268088905));
#135732=CARTESIAN_POINT('Ctrl Pts',(21.361958077986,-0.120566655890619,
-6.22053434867788));
#135733=CARTESIAN_POINT('Ctrl Pts',(21.4067450842764,-0.142950912770123,
-6.21711749014903));
#135734=CARTESIAN_POINT('Ctrl Pts',(21.5218832653832,-0.192196230705459,
-6.20860017259085));
#135735=CARTESIAN_POINT('Ctrl Pts',(21.593536129904,-0.215546003688449,
-6.20354251225363));
#135736=CARTESIAN_POINT('Ctrl Pts',(21.6967487534954,-0.239259994538608,
-6.1966837584893));
#135737=CARTESIAN_POINT('Ctrl Pts',(21.7268916389409,-0.245039932475306,
-6.19472805494932));
#135738=CARTESIAN_POINT('Ctrl Pts',(21.7867340547998,-0.254271292050343,
-6.19093171914911));
#135739=CARTESIAN_POINT('Ctrl Pts',(21.8164046932406,-0.257777703760111,
-6.18909060702583));
#135740=CARTESIAN_POINT('Ctrl Pts',(21.9020793423433,-0.264836167150757,
-6.18387153716627));
#135741=CARTESIAN_POINT('Ctrl Pts',(21.9582325827962,-0.265717211201952,
-6.18057226940304));
#135742=CARTESIAN_POINT('Ctrl Pts',(22.0935696736252,-0.25883031456539,
-6.17270785144827));
#135743=CARTESIAN_POINT('Ctrl Pts',(22.1723140692175,-0.247333554259472,
-6.16820851151158));
#135744=CARTESIAN_POINT('Ctrl Pts',(22.2780889139525,-0.221550862167308,
-6.16175186234005));
#135745=CARTESIAN_POINT('Ctrl Pts',(22.3064677635747,-0.213572949850973,
-6.1599758759125));
#135746=CARTESIAN_POINT('Ctrl Pts',(22.349977044977,-0.199683788943705,
-6.15714914733171));
#135747=CARTESIAN_POINT('Ctrl Pts',(22.3653177106432,-0.194459712317254,
-6.15613187305958));
#135748=CARTESIAN_POINT('Ctrl Pts',(22.3839119206128,-0.187726161438603,
-6.15486919788211));
#135749=CARTESIAN_POINT('Ctrl Pts',(22.3872650050902,-0.186495808226498,
-6.15464034546235));
#135750=CARTESIAN_POINT('Ctrl Pts',(22.3906127229914,-0.185251306606962,
-6.15441073460198));
#135751=CARTESIAN_POINT('Origin',(-21.9500000210213,0.999999999999992,-6.00000000000001));
#135752=CARTESIAN_POINT('',(-23.2146807734794,1.00091784938516,-6.44310584370542));
#135753=CARTESIAN_POINT('Ctrl Pts',(-21.5093309148108,-0.185465194729169,
-6.28967656068295));
#135754=CARTESIAN_POINT('Ctrl Pts',(-21.5528890708403,-0.20176031886336,
-6.29243730725128));
#135755=CARTESIAN_POINT('Ctrl Pts',(-21.5973018538419,-0.215616881063163,
-6.29522299047107));
#135756=CARTESIAN_POINT('Ctrl Pts',(-21.6422693820371,-0.22693499812517,
-6.29808522706224));
#135757=CARTESIAN_POINT('Ctrl Pts',(-21.6453764473183,-0.227717031961227,
-6.2982829954586));
#135758=CARTESIAN_POINT('Ctrl Pts',(-21.6484861751713,-0.228486961817531,
-6.29848112933784));
#135759=CARTESIAN_POINT('Ctrl Pts',(-21.6515984731377,-0.22924476131915,
-6.29867964572721));
#135760=CARTESIAN_POINT('Ctrl Pts',(-21.6658493874608,-0.232714652662521,
-6.29958863326223));
#135761=CARTESIAN_POINT('Ctrl Pts',(-21.6801536623721,-0.235930171416049,
-6.30050567807171));
#135762=CARTESIAN_POINT('Ctrl Pts',(-21.6945013876115,-0.238889048051699,
-6.30143245597623));
#135763=CARTESIAN_POINT('Ctrl Pts',(-21.6945179001323,-0.238892453365868,
-6.30143352258708));
#135764=CARTESIAN_POINT('Ctrl Pts',(-21.6945344127108,-0.238895858340165,
-6.30143458921083));
#135765=CARTESIAN_POINT('Ctrl Pts',(-21.6945509253467,-0.238899262974601,
-6.30143565584746));
#135766=CARTESIAN_POINT('Ctrl Pts',(-21.7395092457333,-0.248168930510011,
-6.30433974649248));
#135767=CARTESIAN_POINT('Ctrl Pts',(-21.7850595616849,-0.254945427799025,
-6.30734676297183));
#135768=CARTESIAN_POINT('Ctrl Pts',(-21.8309034069721,-0.259196362451375,
-6.31039760680955));
#135769=CARTESIAN_POINT('Ctrl Pts',(-21.8358278096666,-0.259652984576445,
-6.31072531892709));
#135770=CARTESIAN_POINT('Ctrl Pts',(-21.8407555546012,-0.260080487322827,
-6.31105353674159));
#135771=CARTESIAN_POINT('Ctrl Pts',(-21.8456862402058,-0.260478846979626,
-6.31138218700536));
#135772=CARTESIAN_POINT('Ctrl Pts',(-21.8951053083839,-0.264471509383489,
-6.31467616903842));
#135773=CARTESIAN_POINT('Ctrl Pts',(-21.9448252828204,-0.265534705092938,
-6.31801304290788));
#135774=CARTESIAN_POINT('Ctrl Pts',(-21.9944798553753,-0.263674227481021,
-6.32133409327276));
#135775=CARTESIAN_POINT('Ctrl Pts',(-22.0440882738254,-0.261815479189773,
-6.32465205670931));
#135776=CARTESIAN_POINT('Ctrl Pts',(-22.0936314933926,-0.25703879462773,
-6.32795393272415));
#135777=CARTESIAN_POINT('Ctrl Pts',(-22.1427525738362,-0.249387020616709,
-6.33120258133066));
#135778=CARTESIAN_POINT('Ctrl Pts',(-22.1918484783148,-0.241739168359695,
-6.33444956491144));
#135779=CARTESIAN_POINT('Ctrl Pts',(-22.2405227063286,-0.231219249570335,
-6.33764328070394));
#135780=CARTESIAN_POINT('Ctrl Pts',(-22.2884263109151,-0.2179043325076,
-6.34077088001125));
#135781=CARTESIAN_POINT('Ctrl Pts',(-22.3388295094863,-0.203894647548285,
-6.34406167639909));
#135782=CARTESIAN_POINT('Ctrl Pts',(-22.3883794239626,-0.186790230387356,
-6.34727909684211));
#135783=CARTESIAN_POINT('Ctrl Pts',(-22.4366787021697,-0.166721976528897,
-6.35043750170706));
#135784=CARTESIAN_POINT('Ctrl Pts',(-22.4826232176231,-0.147632121902707,
-6.35344192302581));
#135785=CARTESIAN_POINT('Ctrl Pts',(-22.5274359833547,-0.125860467509555,
-6.35639336480415));
#135786=CARTESIAN_POINT('Ctrl Pts',(-22.570784448847,-0.101557476263163,
-6.35932743540377));
#135787=CARTESIAN_POINT('Ctrl Pts',(-22.6141592340666,-0.0772397290595335,
-6.36226328747218));
#135788=CARTESIAN_POINT('Ctrl Pts',(-22.6560676193217,-0.0503872190281829,
-6.36518216058722));
#135789=CARTESIAN_POINT('Ctrl Pts',(-22.6961892211718,-0.0211919452919621,
-6.36813777916461));
#135790=CARTESIAN_POINT('Ctrl Pts',(-22.7332273305202,0.00575956439951002,
-6.37086624759594));
#135791=CARTESIAN_POINT('Ctrl Pts',(-22.7687429830093,0.0347080253773226,
-6.37362661811217));
#135792=CARTESIAN_POINT('Ctrl Pts',(-22.8024973740039,0.0654651041167603,
-6.37646888522295));
#135793=CARTESIAN_POINT('Ctrl Pts',(-22.8053679515819,0.0680807810107938,
-6.37671060038944));
#135794=CARTESIAN_POINT('Ctrl Pts',(-22.808225822136,0.0707095423226226,
-6.37695290785885));
#135795=CARTESIAN_POINT('Ctrl Pts',(-22.811070856039,0.0733512748601315,
-6.37719583838075));
#135796=CARTESIAN_POINT('Ctrl Pts',(-22.8165231690677,0.078413974716596,
-6.37766139812267));
#135797=CARTESIAN_POINT('Ctrl Pts',(-22.8219282504577,0.0835242027064733,
-6.37812925196743));
#135798=CARTESIAN_POINT('Ctrl Pts',(-22.8272851303427,0.0886810443488697,
-6.37859961831321));
#135799=CARTESIAN_POINT('Ctrl Pts',(-22.827297335773,0.0886927940002537,
-6.37860069002357));
#135800=CARTESIAN_POINT('Ctrl Pts',(-22.8273095409531,0.0887045438936312,
-6.37860176174696));
#135801=CARTESIAN_POINT('Ctrl Pts',(-22.8273217458829,0.0887162940289741,
-6.37860283348341));
#135802=CARTESIAN_POINT('Ctrl Pts',(-22.8599946799189,0.12017173059851,
-6.3814719015195));
#135803=CARTESIAN_POINT('Ctrl Pts',(-22.8909971419964,0.153490508933891,
-6.38444240110765));
#135804=CARTESIAN_POINT('Ctrl Pts',(-22.9201335387744,0.188451018775665,
-6.3874568890493));
#135805=CARTESIAN_POINT('Ctrl Pts',(-22.9223326145792,0.191089670764765,
-6.38768440817415));
#135806=CARTESIAN_POINT('Ctrl Pts',(-22.9245210576273,0.193737650453255,
-6.387912177879));
#135807=CARTESIAN_POINT('Ctrl Pts',(-22.9266987828115,0.196394850598419,
-6.38814017346644));
#135808=CARTESIAN_POINT('Ctrl Pts',(-22.9576869063787,0.234205703426636,
-6.39138445584307));
#135809=CARTESIAN_POINT('Ctrl Pts',(-22.9865058911464,0.273888863401147,
-6.39467389636256));
#135810=CARTESIAN_POINT('Ctrl Pts',(-23.0129544751761,0.315148437923321,
-6.39795091134187));
#135811=CARTESIAN_POINT('Ctrl Pts',(-23.0393781887874,0.356369214796404,
-6.40122484484302));
#135812=CARTESIAN_POINT('Ctrl Pts',(-23.0634362208576,0.399163291678379,
-6.40448608013678));
#135813=CARTESIAN_POINT('Ctrl Pts',(-23.0849637300028,0.443220519601541,
-6.40769721656754));
#135814=CARTESIAN_POINT('Ctrl Pts',(-23.1064909775948,0.487277212241604,
-6.41090831398387));
#135815=CARTESIAN_POINT('Ctrl Pts',(-23.1254878302226,0.532596958409967,
-6.41406920989122));
#135816=CARTESIAN_POINT('Ctrl Pts',(-23.1418228872495,0.578856055528787,
-6.4171654666348));
#135817=CARTESIAN_POINT('Ctrl Pts',(-23.1581563751267,0.625110708986886,
-6.42026142595116));
#135818=CARTESIAN_POINT('Ctrl Pts',(-23.1718284901437,0.672304482803547,
-6.42329279987827));
#135819=CARTESIAN_POINT('Ctrl Pts',(-23.1827414943878,0.720101049882449,
-6.42626855500388));
#135820=CARTESIAN_POINT('Ctrl Pts',(-23.1936686979045,0.767959806663703,
-6.4292481819834));
#135821=CARTESIAN_POINT('Ctrl Pts',(-23.2018293666031,0.816422871565319,
-6.43217222471905));
#135822=CARTESIAN_POINT('Ctrl Pts',(-23.2071615621788,0.865140613466418,
-6.43507151987879));
#135823=CARTESIAN_POINT('Ctrl Pts',(-23.2121017465369,0.910276734805267,
-6.43775766527513));
#135824=CARTESIAN_POINT('Ctrl Pts',(-23.214614170614,0.955631272551833,
-6.44042302676632));
#135825=CARTESIAN_POINT('Ctrl Pts',(-23.2146807734792,1.00091784928355,
-6.44310584369939));
#135826=CARTESIAN_POINT('Ctrl Pts',(-23.2146807734804,1.00091785003632,
-6.443105843744));
#135827=CARTESIAN_POINT('Ctrl Pts',(-23.2147523872175,1.04961158575364,
-6.4459905037947));
#135828=CARTESIAN_POINT('Ctrl Pts',(-23.211997092343,1.09822149555741,-6.44889468223683));
#135829=CARTESIAN_POINT('Ctrl Pts',(-23.2064230785462,1.14645855753,-6.45188194418482));
#135830=CARTESIAN_POINT('Ctrl Pts',(-23.2040363039612,1.16711351063344,
-6.45316108003847));
#135831=CARTESIAN_POINT('Ctrl Pts',(-23.2011326193651,1.18770074639772,
-6.45445544945693));
#135832=CARTESIAN_POINT('Ctrl Pts',(-23.1977119408825,1.20820041278777,
-6.45577004299616));
#135833=CARTESIAN_POINT('Ctrl Pts',(-23.1977091502273,1.20821713680927,
-6.45577111546681));
#135834=CARTESIAN_POINT('Ctrl Pts',(-23.197706359228,1.20823386077257,-6.45577218795093));
#135835=CARTESIAN_POINT('Ctrl Pts',(-23.1977035678845,1.20825058467767,
-6.4557732604485));
#135836=CARTESIAN_POINT('Ctrl Pts',(-23.1901486642958,1.2535146281704,-6.45867602608016));
#135837=CARTESIAN_POINT('Ctrl Pts',(-23.180056154529,1.29843270908024,-6.46168188285201));
#135838=CARTESIAN_POINT('Ctrl Pts',(-23.167503299968,1.34271493338495,-6.46473173138053));
#135839=CARTESIAN_POINT('Ctrl Pts',(-23.1661509436738,1.34748558889334,
-6.46506030061821));
#135840=CARTESIAN_POINT('Ctrl Pts',(-23.1647700680414,1.35224883035924,
-6.46538938044148));
#135841=CARTESIAN_POINT('Ctrl Pts',(-23.1633607966667,1.3570042714992,-6.46571889695301));
#135842=CARTESIAN_POINT('Ctrl Pts',(-23.1492747632291,1.4045361408835,-6.46901250007524));
#135843=CARTESIAN_POINT('Ctrl Pts',(-23.1323481091942,1.45129317265826,
-6.47234917997492));
#135844=CARTESIAN_POINT('Ctrl Pts',(-23.1127182200878,1.49693579420182,
-6.47567016663973));
#135845=CARTESIAN_POINT('Ctrl Pts',(-23.0931066271162,1.54253587431553,
-6.47898805796259));
#135846=CARTESIAN_POINT('Ctrl Pts',(-23.0707970907848,1.58702380654452,
-6.48228999161174));
#135847=CARTESIAN_POINT('Ctrl Pts',(-23.0459581859298,1.63008211916181,
-6.48553876892156));
#135848=CARTESIAN_POINT('Ctrl Pts',(-23.0211320689732,1.67311826392066,
-6.48878587365224));
#135849=CARTESIAN_POINT('Ctrl Pts',(-22.9937792480166,1.71472631648939,
-6.4919797815873));
#135850=CARTESIAN_POINT('Ctrl Pts',(-22.9640973368353,1.75460859993243,
-6.49510758545456));
#135851=CARTESIAN_POINT('Ctrl Pts',(-22.9328613760098,1.79657899178639,
-6.49839915109771));
#135852=CARTESIAN_POINT('Ctrl Pts',(-22.8990456926618,1.83663788183948,
-6.50161732867082));
#135853=CARTESIAN_POINT('Ctrl Pts',(-22.8629156817652,1.87446168789097,
-6.50477642427912));
#135854=CARTESIAN_POINT('Ctrl Pts',(-22.828553068191,1.91043524004335,-6.50778098417097));
#135855=CARTESIAN_POINT('Ctrl Pts',(-22.7920971253035,1.94438698114695,
-6.51073252334852));
#135856=CARTESIAN_POINT('Ctrl Pts',(-22.7538080087705,1.97606098822029,
-6.51366660703195));
#135857=CARTESIAN_POINT('Ctrl Pts',(-22.7154956932696,2.00775418623713,
-6.51660246844543));
#135858=CARTESIAN_POINT('Ctrl Pts',(-22.6753477704758,2.03716646368514,
-6.5195212659862));
#135859=CARTESIAN_POINT('Ctrl Pts',(-22.6336587410667,2.06406821252966,
-6.52247669504206));
#135860=CARTESIAN_POINT('Ctrl Pts',(-22.595165241663,2.08890789979943,-6.52520558578889));
#135861=CARTESIAN_POINT('Ctrl Pts',(-22.5553573322426,2.11160723825521,
-6.52796629483141));
#135862=CARTESIAN_POINT('Ctrl Pts',(-22.5144968634658,2.13201127977266,
-6.53080884547288));
#135863=CARTESIAN_POINT('Ctrl Pts',(-22.5110317067516,2.13374163685317,
-6.53104990691283));
#135864=CARTESIAN_POINT('Ctrl Pts',(-22.5075589654691,2.13545551390369,
-6.5312915569432));
#135865=CARTESIAN_POINT('Ctrl Pts',(-22.5040787907026,2.13715283142528,
-6.53153382607317));
#135866=CARTESIAN_POINT('Ctrl Pts',(-22.4973676365808,2.14042593126798,
-6.53200101682631));
#135867=CARTESIAN_POINT('Ctrl Pts',(-22.4906289754993,2.14363741043556,
-6.53247051574278));
#135868=CARTESIAN_POINT('Ctrl Pts',(-22.4838640229481,2.14678668763567,
-6.53294254365717));
#135869=CARTESIAN_POINT('Ctrl Pts',(-22.4838486762386,2.146793831964,-6.53294361448142));
#135870=CARTESIAN_POINT('Ctrl Pts',(-22.4838333293938,2.14680097597224,
-6.53294468531869));
#135871=CARTESIAN_POINT('Ctrl Pts',(-22.4838179824138,2.14680811966039,
-6.53294575616898));
#135872=CARTESIAN_POINT('Ctrl Pts',(-22.4422123954647,2.16617462284804,
-6.5358488259889));
#135873=CARTESIAN_POINT('Ctrl Pts',(-22.3994570302705,2.1832524354923,-6.53885494363662));
#135874=CARTESIAN_POINT('Ctrl Pts',(-22.3558346994545,2.19794132542384,
-6.54190500550471));
#135875=CARTESIAN_POINT('Ctrl Pts',(-22.3511372275183,2.1995230989544,-6.54223345150383));
#135876=CARTESIAN_POINT('Ctrl Pts',(-22.3464297508048,2.20107718112541,
-6.542562407083));
#135877=CARTESIAN_POINT('Ctrl Pts',(-22.3417126573151,2.20260345555568,
-6.54289179843821));
#135878=CARTESIAN_POINT('Ctrl Pts',(-22.2945462066872,2.21786474891735,
-6.54618539885695));
#135879=CARTESIAN_POINT('Ctrl Pts',(-22.2464124737228,2.23034523495559,
-6.54952201828973));
#135880=CARTESIAN_POINT('Ctrl Pts',(-22.1976691852061,2.2399661875372,-6.55284290082326));
#135881=CARTESIAN_POINT('Ctrl Pts',(-22.1489713275507,2.24957817297327,
-6.55616068815007));
#135882=CARTESIAN_POINT('Ctrl Pts',(-22.0996650409653,2.25633626804522,
-6.55946247439116));
#135883=CARTESIAN_POINT('Ctrl Pts',(-22.0501074678495,2.26019996472128,
-6.5627110760994));
#135884=CARTESIAN_POINT('Ctrl Pts',(-22.0005754051105,2.26406167251145,
-6.56595800554953));
#135885=CARTESIAN_POINT('Ctrl Pts',(-21.950792302973,2.26503204252326,-6.5691517101272));
#135886=CARTESIAN_POINT('Ctrl Pts',(-21.9011154039486,2.26310571006556,
-6.5722792969579));
#135887=CARTESIAN_POINT('Ctrl Pts',(-21.8488355501432,2.26107844223591,
-6.57557076211541));
#135888=CARTESIAN_POINT('Ctrl Pts',(-21.7966733565268,2.2558424960804,-6.57878881825307));
#135889=CARTESIAN_POINT('Ctrl Pts',(-21.7450458100928,2.2474337646913,-6.58194778816075));
#135890=CARTESIAN_POINT('Ctrl Pts',(-21.6959456463445,2.23943667560541,
-6.58495211337968));
#135891=CARTESIAN_POINT('Ctrl Pts',(-21.6473291691393,2.22856990548032,
-6.58790341833928));
#135892=CARTESIAN_POINT('Ctrl Pts',(-21.5995545560935,2.21490328777289,
-6.59083727866739));
#135893=CARTESIAN_POINT('Ctrl Pts',(-21.5517509859884,2.20122838648063,
-6.59377291726144));
#135894=CARTESIAN_POINT('Ctrl Pts',(-21.5047905323539,2.18474982731193,
-6.59669150293038));
#135895=CARTESIAN_POINT('Ctrl Pts',(-21.4590290914463,2.16558065360346,
-6.59964673746386));
#135896=CARTESIAN_POINT('Ctrl Pts',(-21.4167769564816,2.14788150561707,
-6.6023753440349));
#135897=CARTESIAN_POINT('Ctrl Pts',(-21.3755466541024,2.12788820653758,
-6.60513578132295));
#135898=CARTESIAN_POINT('Ctrl Pts',(-21.3356140119275,2.10572907923901,
-6.60797806776067));
#135899=CARTESIAN_POINT('Ctrl Pts',(-21.3322258568059,2.10384894918605,
-6.60821922654272));
#135900=CARTESIAN_POINT('Ctrl Pts',(-21.328847012584,2.10195323070465,-6.6084609745545));
#135901=CARTESIAN_POINT('Ctrl Pts',(-21.3254776304655,2.10004200355688,
-6.60870334234774));
#135902=CARTESIAN_POINT('Ctrl Pts',(-21.3189779645595,2.09635517389664,
-6.60917087901383));
#135903=CARTESIAN_POINT('Ctrl Pts',(-21.3125136194912,2.09261072292676,
-6.60964072791275));
#135904=CARTESIAN_POINT('Ctrl Pts',(-21.3060857647504,2.08880932601868,
-6.61011311039498));
#135905=CARTESIAN_POINT('Ctrl Pts',(-21.3060711837952,2.08880070292431,
-6.6101141819481));
#135906=CARTESIAN_POINT('Ctrl Pts',(-21.3060566030277,2.08879207953692,
-6.61011525351425));
#135907=CARTESIAN_POINT('Ctrl Pts',(-21.306042022448,2.08878345585653,-6.61011632509345));
#135908=CARTESIAN_POINT('Ctrl Pts',(-21.2665434693734,2.06542204605492,
-6.61301921569763));
#135909=CARTESIAN_POINT('Ctrl Pts',(-21.2282821698809,2.03981827656591,
-6.6160251753714));
#135910=CARTESIAN_POINT('Ctrl Pts',(-21.1915007018088,2.0121486902521,-6.6190750994482));
#135911=CARTESIAN_POINT('Ctrl Pts',(-21.1875381283282,2.00916776603422,
-6.61940367655232));
#135912=CARTESIAN_POINT('Ctrl Pts',(-21.1835927489682,2.00616291138487,
-6.61973276392372));
#135913=CARTESIAN_POINT('Ctrl Pts',(-21.1796648795256,2.00313438080335,
-6.62006228765863));
#135914=CARTESIAN_POINT('Ctrl Pts',(-21.1404065330904,1.97286476403174,
-6.62335581793822));
#135915=CARTESIAN_POINT('Ctrl Pts',(-21.1028945549724,1.94022491479254,
-6.62669238904534));
#135916=CARTESIAN_POINT('Ctrl Pts',(-21.067396164469,1.90546533392439,-6.63001323799809));
#135917=CARTESIAN_POINT('Ctrl Pts',(-21.0319308765439,1.87073816668763,
-6.63333099022841));
#135918=CARTESIAN_POINT('Ctrl Pts',(-20.9984751575207,1.83389539004587,
-6.63663275607506));
#135919=CARTESIAN_POINT('Ctrl Pts',(-20.967264375618,1.79520863567327,-6.63988134452721));
#135920=CARTESIAN_POINT('Ctrl Pts',(-20.9360696725984,1.75654181158648,
-6.64312825940148));
#135921=CARTESIAN_POINT('Ctrl Pts',(-20.9071175204923,1.71603294585134,
-6.64632195655213));
#135922=CARTESIAN_POINT('Ctrl Pts',(-20.8806143595794,1.67397362633977,
-6.64944953539169));
#135923=CARTESIAN_POINT('Ctrl Pts',(-20.852721407826,1.62970877152585,-6.65274112034504));
#135924=CARTESIAN_POINT('Ctrl Pts',(-20.8275414267647,1.58372636025973,
-6.65595928970062));
#135925=CARTESIAN_POINT('Ctrl Pts',(-20.8052806377126,1.53639062643641,
-6.65911835980036));
#135926=CARTESIAN_POINT('Ctrl Pts',(-20.7841104453188,1.49137395655138,
-6.66212266129391));
#135927=CARTESIAN_POINT('Ctrl Pts',(-20.7655804230656,1.44513344291141,
-6.66507393510946));
#135928=CARTESIAN_POINT('Ctrl Pts',(-20.749835519601,1.39800396817185,-6.66800775115554));
#135929=CARTESIAN_POINT('Ctrl Pts',(-20.7340810758135,1.35084593622912,
-6.67094334489131));
#135930=CARTESIAN_POINT('Ctrl Pts',(-20.721115600259,1.30279782170665,-6.67386187247146));
#135931=CARTESIAN_POINT('Ctrl Pts',(-20.7110471154209,1.25421705900154,
-6.67681703171073));
#135932=CARTESIAN_POINT('Ctrl Pts',(-20.7017504542369,1.2093603702151,-6.67954565618941));
#135933=CARTESIAN_POINT('Ctrl Pts',(-20.6949237836073,1.16404907382507,
-6.68230609865919));
#135934=CARTESIAN_POINT('Ctrl Pts',(-20.690617252492,1.11858323857537,-6.68514838180113));
#135935=CARTESIAN_POINT('Ctrl Pts',(-20.6902520072694,1.11472719326355,
-6.68538944132471));
#135936=CARTESIAN_POINT('Ctrl Pts',(-20.689904869376,1.1108700127313,-6.68563108953346));
#135937=CARTESIAN_POINT('Ctrl Pts',(-20.6895758585126,1.10701186658802,
-6.6858733569441));
#135938=CARTESIAN_POINT('Ctrl Pts',(-20.6889404172309,1.09956036391026,
-6.68634126463657));
#135939=CARTESIAN_POINT('Ctrl Pts',(-20.6883725819451,1.09210540127322,
-6.68681148799471));
#135940=CARTESIAN_POINT('Ctrl Pts',(-20.6878724572385,1.08464832842542,
-6.68728424892598));
#135941=CARTESIAN_POINT('Ctrl Pts',(-20.687871323671,1.0846314264489,-6.68728532047166));
#135942=CARTESIAN_POINT('Ctrl Pts',(-20.6878701904512,1.08461452446153,
-6.68728639203037));
#135943=CARTESIAN_POINT('Ctrl Pts',(-20.6878690575793,1.08459762246331,
-6.68728746360212));
#135944=CARTESIAN_POINT('Ctrl Pts',(-20.6848000770319,1.03880965400266,
-6.69019038034012));
#135945=CARTESIAN_POINT('Ctrl Pts',(-20.6842802255432,0.992774090407304,
-6.69319636476006));
#135946=CARTESIAN_POINT('Ctrl Pts',(-20.6863010683395,0.946790840098534,
-6.69624631378546));
#135947=CARTESIAN_POINT('Ctrl Pts',(-20.6865187494249,0.941837617682455,
-6.69657484810565));
#135948=CARTESIAN_POINT('Ctrl Pts',(-20.6867658830337,0.936885043762289,
-6.69690389255425));
#135949=CARTESIAN_POINT('Ctrl Pts',(-20.6870424378518,0.931933522550874,
-6.69723337326016));
#135950=CARTESIAN_POINT('Ctrl Pts',(-20.6898069471317,0.882436911237792,
-6.70052694259754));
#135951=CARTESIAN_POINT('Ctrl Pts',(-20.6955139779276,0.833040295320728,
-6.70386355449708));
#135952=CARTESIAN_POINT('Ctrl Pts',(-20.704108031124,0.784105733031032,
-6.70718444651916));
#135953=CARTESIAN_POINT('Ctrl Pts',(-20.7126940724883,0.735216790134869,
-6.71050224262962));
#135954=CARTESIAN_POINT('Ctrl Pts',(-20.7241614651429,0.686788917641545,
-6.71380405459674));
#135955=CARTESIAN_POINT('Ctrl Pts',(-20.7384192707434,0.639169852304406,
-6.71705269195841));
#135956=CARTESIAN_POINT('Ctrl Pts',(-20.7526697341407,0.59157530889364,
-6.72029965640093));
#135957=CARTESIAN_POINT('Ctrl Pts',(-20.7697076653843,0.544788699697114,
-6.72349340587503));
#135958=CARTESIAN_POINT('Ctrl Pts',(-20.7894093089887,0.499145187221971,
-6.72662104062077));
#135959=CARTESIAN_POINT('Ctrl Pts',(-20.8101434456976,0.451109660515009,
-6.72991258358517));
#135960=CARTESIAN_POINT('Ctrl Pts',(-20.8338282197867,0.404340381200418,
-6.73313071956871));
#135961=CARTESIAN_POINT('Ctrl Pts',(-20.8602798534964,0.359213378678562,
-6.73628976450706));
#135962=CARTESIAN_POINT('Ctrl Pts',(-20.8854363500905,0.316295905311972,
-6.73929413482702));
#135963=CARTESIAN_POINT('Ctrl Pts',(-20.9130952957426,0.274863899665037,
-6.74224548147274));
#135964=CARTESIAN_POINT('Ctrl Pts',(-20.9430624556387,0.235226291994243,
-6.74517937503937));
#135965=CARTESIAN_POINT('Ctrl Pts',(-20.9730477750942,0.195564664646751,
-6.74811504649268));
#135966=CARTESIAN_POINT('Ctrl Pts',(-21.0053444109433,0.157699976187537,
-6.75103365651137));
#135967=CARTESIAN_POINT('Ctrl Pts',(-21.0397186466094,0.121923455120705,
-6.75398890359384));
#135968=CARTESIAN_POINT('Ctrl Pts',(-21.0714575718499,0.0888897510833839,
-6.75671758582924));
#135969=CARTESIAN_POINT('Ctrl Pts',(-21.1049682267046,0.0576361346627014,
-6.75947809015584));
#135970=CARTESIAN_POINT('Ctrl Pts',(-21.1400314862003,0.0283736559177723,
-6.76232043808688));
#135971=CARTESIAN_POINT('Ctrl Pts',(-21.1430055912075,0.0258915796416098,
-6.76256152922717));
#135972=CARTESIAN_POINT('Ctrl Pts',(-21.1459908746752,0.0234237988346693,
-6.76280320920131));
#135973=CARTESIAN_POINT('Ctrl Pts',(-21.1489872078154,0.0209704256960743,
-6.76304550853523));
#135974=CARTESIAN_POINT('Ctrl Pts',(-21.1547699320427,0.0162355782598507,
-6.76351313017908));
#135975=CARTESIAN_POINT('Ctrl Pts',(-21.1605936891247,0.0115544652196716,
-6.76398306463605));
#135976=CARTESIAN_POINT('Ctrl Pts',(-21.1664574270013,0.00692793450649951,
-6.76445553338469));
#135977=CARTESIAN_POINT('Ctrl Pts',(-21.1664707237123,0.00691744330732976,
-6.7644566047628));
#135978=CARTESIAN_POINT('Ctrl Pts',(-21.1664840206289,0.00690695238880424,
-6.76445767615394));
#135979=CARTESIAN_POINT('Ctrl Pts',(-21.1664973177511,0.00689646175092878,
-6.76445874755812));
#135980=CARTESIAN_POINT('Ctrl Pts',(-21.2024808513942,-0.0214924043354978,
-6.76735808981954));
#135981=CARTESIAN_POINT('Ctrl Pts',(-21.2401062505285,-0.0479239427983001,
-6.77036028314935));
#135982=CARTESIAN_POINT('Ctrl Pts',(-21.279121761994,-0.0722355947060704,
-6.77340632508014));
#135983=CARTESIAN_POINT('Ctrl Pts',(-21.2822365164627,-0.0741764849719107,
-6.77364950202077));
#135984=CARTESIAN_POINT('Ctrl Pts',(-21.2853601032168,-0.0761038640448651,
-6.77389295842728));
#135985=CARTESIAN_POINT('Ctrl Pts',(-21.288492379891,-0.0780176494669613,
-6.77413666427833));
#135986=CARTESIAN_POINT('Ctrl Pts',(-21.3307932105313,-0.103862975867311,
-6.77742786777135));
#135987=CARTESIAN_POINT('Ctrl Pts',(-21.3746844652608,-0.127229646128756,
-6.78076396489562));
#135988=CARTESIAN_POINT('Ctrl Pts',(-21.4198363913639,-0.147957598299775,
-6.78408567783295));
#135989=CARTESIAN_POINT('Ctrl Pts',(-21.4492032374382,-0.161439073695795,
-6.7862461223799));
#135990=CARTESIAN_POINT('Ctrl Pts',(-21.4791031666279,-0.1738051603732,
-6.78840082891751));
#135991=CARTESIAN_POINT('Ctrl Pts',(-21.5094433440835,-0.185020348671025,
-6.79053824099259));
#135992=CARTESIAN_POINT('Ctrl Pts',(-21.5093868170662,-0.185251135625031,
-6.6522544014516));
#135993=CARTESIAN_POINT('Ctrl Pts',(-21.4970021902249,-0.180647191407368,
-6.65143989621879));
#135994=CARTESIAN_POINT('Ctrl Pts',(-21.4846892091089,-0.175848947059488,
-6.65063124382325));
#135995=CARTESIAN_POINT('Ctrl Pts',(-21.4228283175852,-0.150618288101447,
-6.64657067847646));
#135996=CARTESIAN_POINT('Ctrl Pts',(-21.3745383918806,-0.12724318529751,
-6.64341097068174));
#135997=CARTESIAN_POINT('Ctrl Pts',(-21.2403132319356,-0.0513896722782414,
-6.63444713150408));
#135998=CARTESIAN_POINT('Ctrl Pts',(-21.158980200687,0.00835566288177159,
-6.62880279875395));
#135999=CARTESIAN_POINT('Ctrl Pts',(-21.0710275547414,0.0907333471529403,
-6.62147891500746));
#136000=CARTESIAN_POINT('Ctrl Pts',(-21.0567892706854,0.104716306006347,
-6.62024791148091));
#136001=CARTESIAN_POINT('Ctrl Pts',(-21.0310187702787,0.131251481673118,
-6.61792044664163));
#136002=CARTESIAN_POINT('Ctrl Pts',(-21.0193984880813,0.143710801499513,
-6.61682998867927));
#136003=CARTESIAN_POINT('Ctrl Pts',(-20.9853955898538,0.18167850615026,
-6.61352208669295));
#136004=CARTESIAN_POINT('Ctrl Pts',(-20.9637852400462,0.207856197129783,
-6.61126205115897));
#136005=CARTESIAN_POINT('Ctrl Pts',(-20.9079975393363,0.28126054778753,
-6.60504335474356));
#136006=CARTESIAN_POINT('Ctrl Pts',(-20.8759888639061,0.330033209153253,
-6.60103926331554));
#136007=CARTESIAN_POINT('Ctrl Pts',(-20.8152027207198,0.438275255375555,
-6.59259353366974));
#136008=CARTESIAN_POINT('Ctrl Pts',(-20.7874817405927,0.498150565786792,
-6.58817795239542));
#136009=CARTESIAN_POINT('Ctrl Pts',(-20.7539781127685,0.588399833319446,
-6.5819365895114));
#136010=CARTESIAN_POINT('Ctrl Pts',(-20.7444346797864,0.617252623269691,
-6.57999827978544));
#136011=CARTESIAN_POINT('Ctrl Pts',(-20.727723115405,0.67463437518271,-6.57624768814011));
#136012=CARTESIAN_POINT('Ctrl Pts',(-20.7204924025503,0.703124860166806,
-6.5744345002805));
#136013=CARTESIAN_POINT('Ctrl Pts',(-20.7029092879162,0.784152653289509,
-6.56939514297486));
#136014=CARTESIAN_POINT('Ctrl Pts',(-20.6948902639548,0.837132860561267,
-6.5662393159371));
#136015=CARTESIAN_POINT('Ctrl Pts',(-20.6815577796816,0.990469720607132,
-6.55729075366656));
#136016=CARTESIAN_POINT('Ctrl Pts',(-20.6848022537679,1.09113985981767,
-6.55165734920069));
#136017=CARTESIAN_POINT('Ctrl Pts',(-20.7029290791665,1.21018232131975,
-6.54434215780434));
#136018=CARTESIAN_POINT('Ctrl Pts',(-20.7064195791314,1.22993503473715,
-6.54310532642317));
#136019=CARTESIAN_POINT('Ctrl Pts',(-20.7137321490241,1.26625315219018,
-6.54077498739096));
#136020=CARTESIAN_POINT('Ctrl Pts',(-20.7174212348531,1.28283989428573,
-6.53968780408896));
#136021=CARTESIAN_POINT('Ctrl Pts',(-20.7293704513592,1.33188114774661,
-6.53641291504399));
#136022=CARTESIAN_POINT('Ctrl Pts',(-20.7385865838009,1.3640861994133,-6.53418390452247));
#136023=CARTESIAN_POINT('Ctrl Pts',(-20.7668278921536,1.44975726022328,
-6.52810247375362));
#136024=CARTESIAN_POINT('Ctrl Pts',(-20.7881913990345,1.50237282705595,
-6.52420636252505));
#136025=CARTESIAN_POINT('Ctrl Pts',(-20.8426835133907,1.61433427157042,
-6.5157285708729));
#136026=CARTESIAN_POINT('Ctrl Pts',(-20.8772098222052,1.67281483091745,
-6.51117820991828));
#136027=CARTESIAN_POINT('Ctrl Pts',(-20.9338196190595,1.75317121262564,
-6.50480300606975));
#136028=CARTESIAN_POINT('Ctrl Pts',(-20.9522720193142,1.77745004081163,
-6.50285730414519));
#136029=CARTESIAN_POINT('Ctrl Pts',(-20.9901798717367,1.8237518588822,-6.49910083611303));
#136030=CARTESIAN_POINT('Ctrl Pts',(-21.0095606392189,1.84581074791794,
-6.49728888167223));
#136031=CARTESIAN_POINT('Ctrl Pts',(-21.0660112356979,1.90571999077067,
-6.49228408434947));
#136032=CARTESIAN_POINT('Ctrl Pts',(-21.1047170012583,1.94194602072816,
-6.48915952161548));
#136033=CARTESIAN_POINT('Ctrl Pts',(-21.2214056149115,2.03815581941333,
-6.48036169293891));
#136034=CARTESIAN_POINT('Ctrl Pts',(-21.3042471389755,2.09161185924171,
-6.47484143699861));
#136035=CARTESIAN_POINT('Ctrl Pts',(-21.4115689812116,2.14433692125753,
-6.46760842362708));
#136036=CARTESIAN_POINT('Ctrl Pts',(-21.4309417711391,2.15325339096281,
-6.46629878194238));
#136037=CARTESIAN_POINT('Ctrl Pts',(-21.4658365575232,2.16825665692896,
-6.46391709360524));
#136038=CARTESIAN_POINT('Ctrl Pts',(-21.4812701598006,2.17453398374778,
-6.46285492664888));
#136039=CARTESIAN_POINT('Ctrl Pts',(-21.524815411337,2.19125034860985,-6.45983860796339));
#136040=CARTESIAN_POINT('Ctrl Pts',(-21.5531798186893,2.20099658192033,
-6.45785296301066));
#136041=CARTESIAN_POINT('Ctrl Pts',(-21.6769200678191,2.23865272427844,
-6.4491735438664));
#136042=CARTESIAN_POINT('Ctrl Pts',(-21.7750595854177,2.25627697119716,
-6.44228095537805));
#136043=CARTESIAN_POINT('Ctrl Pts',(-21.9165692210142,2.26476848774623,
-6.43283376779055));
#136044=CARTESIAN_POINT('Ctrl Pts',(-21.9589846805841,2.26517858140536,
-6.43005853257355));
#136045=CARTESIAN_POINT('Ctrl Pts',(-22.029775093487,2.2623017950378,-6.42552209856486));
#136046=CARTESIAN_POINT('Ctrl Pts',(-22.0581601695301,2.26018707563593,
-6.42372849983404));
#136047=CARTESIAN_POINT('Ctrl Pts',(-22.1192118056452,2.25356032943692,
-6.41991696570142));
#136048=CARTESIAN_POINT('Ctrl Pts',(-22.1518223336909,2.24872501247293,
-6.41790996584829));
#136049=CARTESIAN_POINT('Ctrl Pts',(-22.220899121435,2.23570543425117,-6.41369533146793));
#136050=CARTESIAN_POINT('Ctrl Pts',(-22.2572665399047,2.22716820459328,
-6.41149876216713));
#136051=CARTESIAN_POINT('Ctrl Pts',(-22.3824485176305,2.1918667567163,-6.40392538894816));
#136052=CARTESIAN_POINT('Ctrl Pts',(-22.4686448810944,2.15696274461396,
-6.39870509394675));
#136053=CARTESIAN_POINT('Ctrl Pts',(-22.5722422474158,2.10109017614784,
-6.39165795826604));
#136054=CARTESIAN_POINT('Ctrl Pts',(-22.5938828845439,2.08857688778398,
-6.39013778916279));
#136055=CARTESIAN_POINT('Ctrl Pts',(-22.6289704645237,2.06687579206379,
-6.38756910176284));
#136056=CARTESIAN_POINT('Ctrl Pts',(-22.6426354602233,2.05805524863577,
-6.38654076399397));
#136057=CARTESIAN_POINT('Ctrl Pts',(-22.6760951616742,2.03553150371386,
-6.38395047645573));
#136058=CARTESIAN_POINT('Ctrl Pts',(-22.6956738591022,2.0215233755612,-6.3823721386644));
#136059=CARTESIAN_POINT('Ctrl Pts',(-22.7403970504793,1.98755395507167,
-6.3786386253462));
#136060=CARTESIAN_POINT('Ctrl Pts',(-22.7652051100249,1.9671766794096,-6.37646805421133));
#136061=CARTESIAN_POINT('Ctrl Pts',(-22.8549911663522,1.88751602877188,
-6.36829710044216));
#136062=CARTESIAN_POINT('Ctrl Pts',(-22.9145128670383,1.82244252281694,
-6.36224766542795));
#136063=CARTESIAN_POINT('Ctrl Pts',(-22.989086276843,1.72157137713819,-6.35395080733568));
#136064=CARTESIAN_POINT('Ctrl Pts',(-23.0100213250107,1.69044969438836,
-6.35151397885211));
#136065=CARTESIAN_POINT('Ctrl Pts',(-23.0441127035126,1.63455532280189,
-6.34734289030684));
#136066=CARTESIAN_POINT('Ctrl Pts',(-23.0578852617868,1.61019136543082,
-6.34558822531375));
#136067=CARTESIAN_POINT('Ctrl Pts',(-23.0871268986927,1.55420266516301,
-6.34168662776561));
#136068=CARTESIAN_POINT('Ctrl Pts',(-23.1021070341037,1.52234843119303,
-6.33955695681918));
#136069=CARTESIAN_POINT('Ctrl Pts',(-23.1319632385754,1.45130543625157,
-6.33496610105155));
#136070=CARTESIAN_POINT('Ctrl Pts',(-23.1462596107942,1.41191863480103,
-6.33252203161919));
#136071=CARTESIAN_POINT('Ctrl Pts',(-23.182207903786,1.29509416136878,-6.32544540608318));
#136072=CARTESIAN_POINT('Ctrl Pts',(-23.1984639498658,1.2162237043578,-6.32088955103311));
#136073=CARTESIAN_POINT('Ctrl Pts',(-23.2098865673701,1.1109099850932,-6.31455818574808));
#136074=CARTESIAN_POINT('Ctrl Pts',(-23.2118728653557,1.08539242329968,
-6.31300424434368));
#136075=CARTESIAN_POINT('Ctrl Pts',(-23.2138550976213,1.04354800777466,
-6.31039881337899));
#136076=CARTESIAN_POINT('Ctrl Pts',(-23.2143114567595,1.0272510540721,-6.30936911836072));
#136077=CARTESIAN_POINT('Ctrl Pts',(-23.2146576302375,0.98727302373077,
-6.30680415675638));
#136078=CARTESIAN_POINT('Ctrl Pts',(-23.2141976115936,0.963597598331454,
-6.30525361561269));
#136079=CARTESIAN_POINT('Ctrl Pts',(-23.2115916996031,0.908784870456056,
-6.30161036620721));
#136080=CARTESIAN_POINT('Ctrl Pts',(-23.2089570647934,0.87768596553925,
-6.29950334034772));
#136081=CARTESIAN_POINT('Ctrl Pts',(-23.1945338626333,0.759579094743743,
-6.29141267589574));
#136082=CARTESIAN_POINT('Ctrl Pts',(-23.1748455365704,0.67377459892076,
-6.28537099253779));
#136083=CARTESIAN_POINT('Ctrl Pts',(-23.1339265523788,0.554164623880316,
-6.27699618822844));
#136084=CARTESIAN_POINT('Ctrl Pts',(-23.1197603227409,0.518219415416183,
-6.27448223154372));
#136085=CARTESIAN_POINT('Ctrl Pts',(-23.0924083533556,0.457171300286188,
-6.27021532486726));
#136086=CARTESIAN_POINT('Ctrl Pts',(-23.0799839556492,0.431760352740889,
-6.26843986115372));
#136087=CARTESIAN_POINT('Ctrl Pts',(-23.0502495411082,0.375785753884799,
-6.26452035056393));
#136088=CARTESIAN_POINT('Ctrl Pts',(-23.0324973490981,0.34548316596362,
-6.26239268909699));
#136089=CARTESIAN_POINT('Ctrl Pts',(-22.991038177419,0.281025173994651,
-6.25782025231511));
#136090=CARTESIAN_POINT('Ctrl Pts',(-22.9668621667606,0.247220524323781,
-6.25539186112436));
#136091=CARTESIAN_POINT('Ctrl Pts',(-22.8910336525855,0.151527541332093,
-6.24831199079154));
#136092=CARTESIAN_POINT('Ctrl Pts',(-22.8350872144647,0.0933200213287932,
-6.24373967145049));
#136093=CARTESIAN_POINT('Ctrl Pts',(-22.7542397875024,0.0238665009735284,
-6.23737024999725));
#136094=CARTESIAN_POINT('Ctrl Pts',(-22.733971408656,0.00751479920781506,
-6.23578962104664));
#136095=CARTESIAN_POINT('Ctrl Pts',(-22.6999867559428,-0.0182118570375911,
-6.23313925031822));
#136096=CARTESIAN_POINT('Ctrl Pts',(-22.68656546832,-0.0279624341031814,
-6.23209166121726));
#136097=CARTESIAN_POINT('Ctrl Pts',(-22.6527815928084,-0.0515050878096002,
-6.22945063463704));
#136098=CARTESIAN_POINT('Ctrl Pts',(-22.6322030976972,-0.064971209058915,
-6.22784051876266));
#136099=CARTESIAN_POINT('Ctrl Pts',(-22.583066427279,-0.0951165239884055,
-6.22401479469022));
#136100=CARTESIAN_POINT('Ctrl Pts',(-22.5542202376943,-0.111292487676677,
-6.22178335526167));
#136101=CARTESIAN_POINT('Ctrl Pts',(-22.4299148142328,-0.174727142567352,
-6.21230976520936));
#136102=CARTESIAN_POINT('Ctrl Pts',(-22.3292998411566,-0.210966985010121,
-6.20503261708783));
#136103=CARTESIAN_POINT('Ctrl Pts',(-22.1959551179931,-0.240714213003921,
-6.19620797740491));
#136104=CARTESIAN_POINT('Ctrl Pts',(-22.1663606706167,-0.246215860613299,
-6.19429483274812));
#136105=CARTESIAN_POINT('Ctrl Pts',(-22.1065187448456,-0.255144184014924,
-6.19051003223404));
#136106=CARTESIAN_POINT('Ctrl Pts',(-22.076287695335,-0.258545463157658,
-6.1886402899011));
#136107=CARTESIAN_POINT('Ctrl Pts',(-21.9815568978915,-0.265755262406095,
-6.18288797933221));
#136108=CARTESIAN_POINT('Ctrl Pts',(-21.9168684953216,-0.265715493425707,
-6.17911856337654));
#136109=CARTESIAN_POINT('Ctrl Pts',(-21.7648057862798,-0.253950863845791,
-6.17030528920132));
#136110=CARTESIAN_POINT('Ctrl Pts',(-21.6781073295134,-0.238047029935697,
-6.16532090699785));
#136111=CARTESIAN_POINT('Ctrl Pts',(-21.5750936585617,-0.207801460718238,
-6.15878424981587));
#136112=CARTESIAN_POINT('Ctrl Pts',(-21.5565470372811,-0.201887598518051,
-6.1575814016423));
#136113=CARTESIAN_POINT('Ctrl Pts',(-21.5285172000524,-0.192231600010188,
-6.15571343033484));
#136114=CARTESIAN_POINT('Ctrl Pts',(-21.518930357273,-0.188798915329577,
-6.15506523016673));
#136115=CARTESIAN_POINT('Ctrl Pts',(-21.5093868082137,-0.185251132334142,
-6.15441066307283));
#136116=CARTESIAN_POINT('Ctrl Pts',(-20.9936430045563,1.82409301376269,
-6.00117192218052));
#136117=CARTESIAN_POINT('Ctrl Pts',(-20.7271798796497,1.51487473521959,
-6.02690195485214));
#136118=CARTESIAN_POINT('Ctrl Pts',(-20.5209353847399,0.623305030710792,
-6.07835570240434));
#136119=CARTESIAN_POINT('Ctrl Pts',(-21.4536811939941,-0.39338969715931,
-6.15553316483713));
#136120=CARTESIAN_POINT('Ctrl Pts',(-22.8180405859452,-0.196442644913706,
-6.23270430947889));
#136121=CARTESIAN_POINT('Ctrl Pts',(-23.4278797311105,1.03891461924669,
-6.30987545412066));
#136122=CARTESIAN_POINT('Ctrl Pts',(-22.7535238523448,2.24109353052079,
-6.38704659876242));
#136123=CARTESIAN_POINT('Ctrl Pts',(-21.3808545992212,2.36444027989689,
-6.46421774340418));
#136124=CARTESIAN_POINT('Ctrl Pts',(-20.5027990432502,1.30223244993389,
-6.54138888804594));
#136125=CARTESIAN_POINT('Ctrl Pts',(-20.8823603280752,-0.0226928241682067,
-6.6185600326877));
#136126=CARTESIAN_POINT('Ctrl Pts',(-22.1897133690524,-0.458853923907108,
-6.69573117732946));
#136127=CARTESIAN_POINT('Ctrl Pts',(-23.2887511850415,0.372721156485589,
-6.77290232197122));
#136128=CARTESIAN_POINT('Ctrl Pts',(-23.2244061652798,1.74941481466079,
-6.85007346661298));
#136129=CARTESIAN_POINT('Ctrl Pts',(-22.052592595292,2.47485743098409,-6.92724461125474));
#136130=CARTESIAN_POINT('Ctrl Pts',(-20.7916257543038,1.91864064422539,
-7.00441575589651));
#136131=CARTESIAN_POINT('Ctrl Pts',(-20.5372939483187,0.56411783578739,
-7.08158690053826));
#136132=CARTESIAN_POINT('Ctrl Pts',(-21.5106140510918,-0.411620184201609,
-7.15875804518003));
#136133=CARTESIAN_POINT('Ctrl Pts',(-22.8657628892087,-0.160649838355007,
-7.23592918982179));
#136134=CARTESIAN_POINT('Ctrl Pts',(-23.4251088531142,1.09893188787309,
-7.31310033446354));
#136135=CARTESIAN_POINT('Ctrl Pts',(-22.7025719108783,2.27254429285729,
-7.39027147910531));
#136136=CARTESIAN_POINT('Ctrl Pts',(-21.3260507987151,2.34030020089029,
-7.46744262374707));
#136137=CARTESIAN_POINT('Ctrl Pts',(-20.4917335473499,1.24333930698749,
-7.54461376838883));
#136138=CARTESIAN_POINT('Ctrl Pts',(-20.9246853421692,-0.0651126387312084,
-7.62178491303059));
#136139=CARTESIAN_POINT('Ctrl Pts',(-22.2485912883136,-0.447918175746809,
-7.69895605767235));
#136140=CARTESIAN_POINT('Ctrl Pts',(-23.3131243221307,0.427413029548789,
-7.77612720231412));
#136141=CARTESIAN_POINT('Ctrl Pts',(-23.1928787033875,1.80055940816669,
-7.85329834695587));
#136142=CARTESIAN_POINT('Ctrl Pts',(-21.9929993552513,2.47753865674549,
-7.93046949159765));
#136143=CARTESIAN_POINT('Ctrl Pts',(-20.7548625344256,1.87150078275659,
-8.00764063623939));
#136144=CARTESIAN_POINT('Ctrl Pts',(-20.5571190900327,0.505939988512289,
-8.08482166293017));
#136145=CARTESIAN_POINT('Ctrl Pts',(-21.2299640074188,-0.114446298241111,
-8.13627897474035));
#136146=CARTESIAN_POINT('Ctrl Pts',(-21.6244020672167,-0.219727019003528,
-8.16201257166996));
#136147=CARTESIAN_POINT('Ctrl Pts',(-20.9215174516537,1.88624361572157,
-5.9462028619613));
#136148=CARTESIAN_POINT('Ctrl Pts',(-20.6349584840009,1.5537050300928,-5.97193289463292));
#136149=CARTESIAN_POINT('Ctrl Pts',(-20.413159653239,0.594895835747109,
-6.02338664218513));
#136150=CARTESIAN_POINT('Ctrl Pts',(-21.4162503295794,-0.498474932679462,
-6.10056410461792));
#136151=CARTESIAN_POINT('Ctrl Pts',(-22.8835055792575,-0.286674729579892,
-6.17773524925968));
#136152=CARTESIAN_POINT('Ctrl Pts',(-23.5393369477972,1.0418494421014,-6.25490639390145));
#136153=CARTESIAN_POINT('Ctrl Pts',(-22.8141231887923,2.33469304989657,
-6.3320775385432));
#136154=CARTESIAN_POINT('Ctrl Pts',(-21.3379313733521,2.4673422379482,-6.40924868318497));
#136155=CARTESIAN_POINT('Ctrl Pts',(-20.3936555237423,1.32502590696021,
-6.48641982782672));
#136156=CARTESIAN_POINT('Ctrl Pts',(-20.8018421723771,-0.0998212230013129,
-6.56359097246849));
#136157=CARTESIAN_POINT('Ctrl Pts',(-22.2077918245531,-0.568876273358851,
-6.64076211711025));
#136158=CARTESIAN_POINT('Ctrl Pts',(-23.389715747691,0.325413683822369,
-6.71793326175202));
#136159=CARTESIAN_POINT('Ctrl Pts',(-23.3205180212025,1.80593341276833,
-6.79510440639377));
#136160=CARTESIAN_POINT('Ctrl Pts',(-22.060329816869,2.58608671652385,-6.87227555103553));
#136161=CARTESIAN_POINT('Ctrl Pts',(-20.7042646715523,1.98792174243761,
-6.94944669567729));
#136162=CARTESIAN_POINT('Ctrl Pts',(-20.4307519301931,0.531244921642298,
-7.02661784031905));
#136163=CARTESIAN_POINT('Ctrl Pts',(-21.4774768905197,-0.518080307901676,
-7.10378898496081));
#136164=CARTESIAN_POINT('Ctrl Pts',(-22.9348269542584,-0.248182537834989,
-7.18096012960258));
#136165=CARTESIAN_POINT('Ctrl Pts',(-23.5363570985653,1.10639303155661,
-7.25813127424434));
#136166=CARTESIAN_POINT('Ctrl Pts',(-22.7593286060459,2.36851573358007,
-7.3353024188861));
#136167=CARTESIAN_POINT('Ctrl Pts',(-21.2789944360103,2.44138158721428,
-7.41247356352786));
#136168=CARTESIAN_POINT('Ctrl Pts',(-20.3817555016178,1.26169122134304,
-7.48964470816962));
#136169=CARTESIAN_POINT('Ctrl Pts',(-20.8473592109878,-0.145440211645416,
-7.56681585281138));
#136170=CARTESIAN_POINT('Ctrl Pts',(-22.2711101383608,-0.557115784156377,
-7.64398699745315));
#136171=CARTESIAN_POINT('Ctrl Pts',(-23.4159270330431,0.384230252492084,
-7.7211581420949));
#136172=CARTESIAN_POINT('Ctrl Pts',(-23.2866128535148,1.86093517678805,
-7.79832928673667));
#136173=CARTESIAN_POINT('Ctrl Pts',(-21.9962422349526,2.58897015222068,
-7.87550043137843));
#136174=CARTESIAN_POINT('Ctrl Pts',(-20.6647288808513,1.93722673522966,
-7.95267157602019));
#136175=CARTESIAN_POINT('Ctrl Pts',(-20.4520722241179,0.468679477131948,
-8.02985260271096));
#136176=CARTESIAN_POINT('Ctrl Pts',(-21.1756610696071,-0.198494466505865,
-8.08130991452115));
#136177=CARTESIAN_POINT('Ctrl Pts',(-21.5998464545764,-0.311715140721045,
-8.10704351145075));
#136178=CARTESIAN_POINT('Ctrl Pts',(-20.8493918987509,1.94839421768056,
-5.89123380174209));
#136179=CARTESIAN_POINT('Ctrl Pts',(-20.542737088352,1.59253532496602,-5.91696383441371));
#136180=CARTESIAN_POINT('Ctrl Pts',(-20.305383921738,0.566486640783421,
-5.96841758196591));
#136181=CARTESIAN_POINT('Ctrl Pts',(-21.3788194651646,-0.603560168199624,
-6.04559504439872));
#136182=CARTESIAN_POINT('Ctrl Pts',(-22.9489705725699,-0.376906814246074,
-6.12276618904047));
#136183=CARTESIAN_POINT('Ctrl Pts',(-23.6507941644838,1.04478426495611,
-6.19993733368224));
#136184=CARTESIAN_POINT('Ctrl Pts',(-22.8747225252399,2.42829256927247,
-6.27710847832399));
#136185=CARTESIAN_POINT('Ctrl Pts',(-21.2950081474827,2.57024419599943,
-6.35427962296576));
#136186=CARTESIAN_POINT('Ctrl Pts',(-20.2845120042343,1.34781936398652,
-6.43145076760751));
#136187=CARTESIAN_POINT('Ctrl Pts',(-20.7213240166791,-0.176949621834419,
-6.50862191224927));
#136188=CARTESIAN_POINT('Ctrl Pts',(-22.2258702800536,-0.678898622810493,
-6.58579305689104));
#136189=CARTESIAN_POINT('Ctrl Pts',(-23.4906803103405,0.278106211159241,
-6.6629642015328));
#136190=CARTESIAN_POINT('Ctrl Pts',(-23.4166298771255,1.86245201087587,
-6.74013534617456));
#136191=CARTESIAN_POINT('Ctrl Pts',(-22.0680670384458,2.69731600206373,
-6.81730649081632));
#136192=CARTESIAN_POINT('Ctrl Pts',(-20.6169035888008,2.05720284064994,
-6.89447763545808));
#136193=CARTESIAN_POINT('Ctrl Pts',(-20.3242099120676,0.498372007497316,
-6.97164878009984));
#136194=CARTESIAN_POINT('Ctrl Pts',(-21.4443397299475,-0.624540431601641,
-7.04881992474161));
#136195=CARTESIAN_POINT('Ctrl Pts',(-23.003891019308,-0.335715237314962,
-7.12599106938337));
#136196=CARTESIAN_POINT('Ctrl Pts',(-23.647605344016,1.11385417524012,-7.20316221402513));
#136197=CARTESIAN_POINT('Ctrl Pts',(-22.8160853012138,2.46448717430285,
-7.28033335866689));
#136198=CARTESIAN_POINT('Ctrl Pts',(-21.2319380733055,2.54246297353816,
-7.35750450330865));
#136199=CARTESIAN_POINT('Ctrl Pts',(-20.2717774558857,1.28004313569848,
-7.43467564795041));
#136200=CARTESIAN_POINT('Ctrl Pts',(-20.7700330798062,-0.225767784559823,
-7.51184679259217));
#136201=CARTESIAN_POINT('Ctrl Pts',(-22.293628988408,-0.666313392565936,
-7.58901793723394));
#136202=CARTESIAN_POINT('Ctrl Pts',(-23.5187297439555,0.341047475435277,
-7.66618908187569));
#136203=CARTESIAN_POINT('Ctrl Pts',(-23.3803470036423,1.92131094540931,
-7.74336022651746));
#136204=CARTESIAN_POINT('Ctrl Pts',(-21.9994851146537,2.70040164769598,
-7.82053137115922));
#136205=CARTESIAN_POINT('Ctrl Pts',(-20.5745952272768,2.00295268770264,
-7.89770251580098));
#136206=CARTESIAN_POINT('Ctrl Pts',(-20.3470253582032,0.431418965751602,
-7.97488354249176));
#136207=CARTESIAN_POINT('Ctrl Pts',(-21.1213581317953,-0.282542634770624,
-8.02634085430194));
#136208=CARTESIAN_POINT('Ctrl Pts',(-21.5752908419361,-0.403703262438664,
-8.05207445123154));
#136209=CARTESIAN_POINT('Ctrl Pts',(-20.7772663458482,2.01054481963934,
-5.83626474152288));
#136210=CARTESIAN_POINT('Ctrl Pts',(-20.4505156927031,1.63136561983912,
-5.8619947741945));
#136211=CARTESIAN_POINT('Ctrl Pts',(-20.1976081902372,0.538077445819645,
-5.9134485217467));
#136212=CARTESIAN_POINT('Ctrl Pts',(-21.3413886007498,-0.708645403719883,
-5.9906259841795));
#136213=CARTESIAN_POINT('Ctrl Pts',(-23.0144355658823,-0.467138898912465,
-6.06779712882125));
#136214=CARTESIAN_POINT('Ctrl Pts',(-23.7622513811704,1.04771908781081,
-6.14496827346302));
#136215=CARTESIAN_POINT('Ctrl Pts',(-22.9353218616875,2.52189208864826,
-6.22213941810477));
#136216=CARTESIAN_POINT('Ctrl Pts',(-21.2520849216134,2.67314615405075,
-6.29931056274654));
#136217=CARTESIAN_POINT('Ctrl Pts',(-20.1753684847264,1.37061282101294,
-6.37648170738831));
#136218=CARTESIAN_POINT('Ctrl Pts',(-20.640805860981,-0.254078020667521,
-6.45365285203007));
#136219=CARTESIAN_POINT('Ctrl Pts',(-22.2439487355543,-0.788920972262233,
-6.53082399667182));
#136220=CARTESIAN_POINT('Ctrl Pts',(-23.5916448729899,0.230798738496012,
-6.60799514131358));
#136221=CARTESIAN_POINT('Ctrl Pts',(-23.5127417330482,1.9189706089834,-6.68516628595534));
#136222=CARTESIAN_POINT('Ctrl Pts',(-22.0758042600227,2.8085452876036,-6.76233743059711));
#136223=CARTESIAN_POINT('Ctrl Pts',(-20.5295425060494,2.12648393886206,
-6.83950857523886));
#136224=CARTESIAN_POINT('Ctrl Pts',(-20.217667893942,0.465499093352224,
-6.91667971988063));
#136225=CARTESIAN_POINT('Ctrl Pts',(-21.4112025693755,-0.731000555301602,
-6.99385086452238));
#136226=CARTESIAN_POINT('Ctrl Pts',(-23.0729550843577,-0.423247936795041,
-7.07102200916415));
#136227=CARTESIAN_POINT('Ctrl Pts',(-23.758853589467,1.12131531892362,-7.14819315380591));
#136228=CARTESIAN_POINT('Ctrl Pts',(-22.8728419963814,2.56045861502574,
-7.22536429844767));
#136229=CARTESIAN_POINT('Ctrl Pts',(-21.1848817106007,2.64354435986205,
-7.30253544308943));
#136230=CARTESIAN_POINT('Ctrl Pts',(-20.1617994101534,1.29839505005402,
-7.37970658773119));
#136231=CARTESIAN_POINT('Ctrl Pts',(-20.6927069486246,-0.30609535747403,
-7.45687773237295));
#136232=CARTESIAN_POINT('Ctrl Pts',(-22.3161478384553,-0.775511000975397,
-7.53404887701472));
#136233=CARTESIAN_POINT('Ctrl Pts',(-23.6215324548678,0.297864698378567,
-7.61122002165647));
#136234=CARTESIAN_POINT('Ctrl Pts',(-23.4740811537695,1.98168671403077,
-7.68839116629823));
#136235=CARTESIAN_POINT('Ctrl Pts',(-22.0027279943549,2.81183314317116,
-7.76556231094));
#136236=CARTESIAN_POINT('Ctrl Pts',(-20.4844615737024,2.06867864017571,
-7.84273345558175));
#136237=CARTESIAN_POINT('Ctrl Pts',(-20.2419784922884,0.394158454371154,
-7.91991448227254));
#136238=CARTESIAN_POINT('Ctrl Pts',(-21.0670551939834,-0.366590803035485,
-7.97137179408272));
#136239=CARTESIAN_POINT('Ctrl Pts',(-21.5507352292958,-0.495691384156185,
-7.99710539101233));
#136240=CARTESIAN_POINT('Ctrl Pts',(-21.5514861791641,-0.490649428218476,
-8.00000000000001));
#136241=CARTESIAN_POINT('Ctrl Pts',(-21.4053161238347,-0.437239491620633,
-8.00000000000001));
#136242=CARTESIAN_POINT('Ctrl Pts',(-21.2682206866264,-0.360071395527733,
-8.));
#136243=CARTESIAN_POINT('Ctrl Pts',(-21.0263626032413,-0.171118288369296,
-8.));
#136244=CARTESIAN_POINT('Ctrl Pts',(-20.9206285329538,-0.0601882408216436,
-8.));
#136245=CARTESIAN_POINT('Ctrl Pts',(-20.7358892338651,0.203461517749917,
-8.));
#136246=CARTESIAN_POINT('Ctrl Pts',(-20.6619493872077,0.35988357861727,
-8.));
#136247=CARTESIAN_POINT('Ctrl Pts',(-20.5805393518183,0.685725923832186,
-8.));
#136248=CARTESIAN_POINT('Ctrl Pts',(-20.5715184850394,0.853392047783976,
-8.));
#136249=CARTESIAN_POINT('Ctrl Pts',(-20.6100559739075,1.17524495044367,
-8.));
#136250=CARTESIAN_POINT('Ctrl Pts',(-20.6557618690624,1.33069459916174,
-8.));
#136251=CARTESIAN_POINT('Ctrl Pts',(-20.8004717406764,1.61978786133916,
-8.));
#136252=CARTESIAN_POINT('Ctrl Pts',(-20.8928208619793,1.73842020633026,
-8.00000000000001));
#136253=CARTESIAN_POINT('Ctrl Pts',(-21.001487092682,1.83623171117383,-8.00000000000001));
#136254=CARTESIAN_POINT('Ctrl Pts',(-20.9918838682989,1.82521129893649,
-6.00000000000001));
#136255=CARTESIAN_POINT('Ctrl Pts',(-20.9541736575533,1.7899949737847,-6.00000000000002));
#136256=CARTESIAN_POINT('Ctrl Pts',(-20.9189421950651,1.75244099022259,
-6.));
#136257=CARTESIAN_POINT('Ctrl Pts',(-20.8861950831707,1.71288999786489,
-6.00000000000001));
#136258=CARTESIAN_POINT('Ctrl Pts',(-20.8534479712762,1.67333900550718,
-6.00000000000002));
#136259=CARTESIAN_POINT('Ctrl Pts',(-20.8231848002971,1.63179022769739,
-6.00000000000002));
#136260=CARTESIAN_POINT('Ctrl Pts',(-20.7954373175153,1.58853787365536,
-6.00000000000003));
#136261=CARTESIAN_POINT('Ctrl Pts',(-20.7732296613486,1.55392091706439,
-6.00000000000004));
#136262=CARTESIAN_POINT('Ctrl Pts',(-20.7526338659112,1.51821167100359,
-6.00000000000001));
#136263=CARTESIAN_POINT('Ctrl Pts',(-20.7336809691674,1.48154464880145,
-6.00000000000003));
#136264=CARTESIAN_POINT('Ctrl Pts',(-20.7265367050108,1.46772307334569,
-6.00000000000004));
#136265=CARTESIAN_POINT('Ctrl Pts',(-20.7196260261576,1.45376528333739,
-6.00000000000004));
#136266=CARTESIAN_POINT('Ctrl Pts',(-20.7129511478733,1.43967807833951,
-6.00000000000002));
#136267=CARTESIAN_POINT('Ctrl Pts',(-20.7070329743969,1.42718788459759,
-6.00000000000001));
#136268=CARTESIAN_POINT('Ctrl Pts',(-20.7012980994116,1.4145908100944,-6.00000000000002));
#136269=CARTESIAN_POINT('Ctrl Pts',(-20.6957608152527,1.40192135070849,
-6.00000000000002));
#136270=CARTESIAN_POINT('Ctrl Pts',(-20.6737369136607,1.3515300544102,-6.00000000000005));
#136271=CARTESIAN_POINT('Ctrl Pts',(-20.6547985766653,1.2999241035713,-6.00000000000003));
#136272=CARTESIAN_POINT('Ctrl Pts',(-20.638977977284,1.24744397487004,-6.00000000000003));
#136273=CARTESIAN_POINT('Ctrl Pts',(-20.6231888036185,1.19506809162579,
-6.00000000000002));
#136274=CARTESIAN_POINT('Ctrl Pts',(-20.610504532974,1.14182048266499,-6.00000000000001));
#136275=CARTESIAN_POINT('Ctrl Pts',(-20.6009967006508,1.08800620437009,
-6.));
#136276=CARTESIAN_POINT('Ctrl Pts',(-20.5944877417198,1.05116553286749,
-5.99999999999999));
#136277=CARTESIAN_POINT('Ctrl Pts',(-20.5894682777219,1.0140585905501,-6.00000000000001));
#136278=CARTESIAN_POINT('Ctrl Pts',(-20.5859737043841,0.976777961364623,
-6.));
#136279=CARTESIAN_POINT('Ctrl Pts',(-20.5845817085914,0.961927942790997,
-6.));
#136280=CARTESIAN_POINT('Ctrl Pts',(-20.5834317834929,0.947050334331592,
-6.00000000000002));
#136281=CARTESIAN_POINT('Ctrl Pts',(-20.5825266608602,0.932150896779572,
-6.00000000000001));
#136282=CARTESIAN_POINT('Ctrl Pts',(-20.5818018340487,0.92021935134809,
-5.99999999999999));
#136283=CARTESIAN_POINT('Ctrl Pts',(-20.5812340735239,0.908271702282496,
-5.99999999999999));
#136284=CARTESIAN_POINT('Ctrl Pts',(-20.5808252608828,0.896333462267451,
-5.99999999999998));
#136285=CARTESIAN_POINT('Ctrl Pts',(-20.5788807239938,0.839548652388208,
-5.99999999999997));
#136286=CARTESIAN_POINT('Ctrl Pts',(-20.5805204587098,0.782868892275996,
-6.00000000000001));
#136287=CARTESIAN_POINT('Ctrl Pts',(-20.5858064535069,0.726625924331545,
-6.00000000000003));
#136288=CARTESIAN_POINT('Ctrl Pts',(-20.5884730759742,0.698253069701404,
-6.00000000000004));
#136289=CARTESIAN_POINT('Ctrl Pts',(-20.5920683585492,0.669990976519162,
-6.00000000000004));
#136290=CARTESIAN_POINT('Ctrl Pts',(-20.596605014284,0.641880555611109,
-6.00000000000004));
#136291=CARTESIAN_POINT('Ctrl Pts',(-20.6053457226608,0.587720618010693,
-6.00000000000002));
#136292=CARTESIAN_POINT('Ctrl Pts',(-20.6175775576439,0.534123432324477,
-6.00000000000002));
#136293=CARTESIAN_POINT('Ctrl Pts',(-20.6330757343097,0.481297854682912,
-6.00000000000002));
#136294=CARTESIAN_POINT('Ctrl Pts',(-20.641649315731,0.452074778910586,
-6.00000000000002));
#136295=CARTESIAN_POINT('Ctrl Pts',(-20.6512234402395,0.423087837825986,
-5.99999999999999));
#136296=CARTESIAN_POINT('Ctrl Pts',(-20.6617666141062,0.394373265917769,
-6.00000000000002));
#136297=CARTESIAN_POINT('Ctrl Pts',(-20.6648813824875,0.385890123953785,
-6.00000000000002));
#136298=CARTESIAN_POINT('Ctrl Pts',(-20.6680800797172,0.377432774733792,
-6.00000000000001));
#136299=CARTESIAN_POINT('Ctrl Pts',(-20.671358423858,0.369010458514467,
-6.00000000000001));
#136300=CARTESIAN_POINT('Ctrl Pts',(-20.6919756536175,0.31604322226919,
-6.00000000000001));
#136301=CARTESIAN_POINT('Ctrl Pts',(-20.7157726857117,0.26436761155119,
-6.00000000000002));
#136302=CARTESIAN_POINT('Ctrl Pts',(-20.7424735625905,0.21420120207078,
-6.00000000000001));
#136303=CARTESIAN_POINT('Ctrl Pts',(-20.7697924963213,0.162873568812587,
-6.00000000000001));
#136304=CARTESIAN_POINT('Ctrl Pts',(-20.8001515955868,0.113124889015486,
-6.));
#136305=CARTESIAN_POINT('Ctrl Pts',(-20.8333103098429,0.0651935718726574,
-6.00000000000003));
#136306=CARTESIAN_POINT('Ctrl Pts',(-20.8552521517862,0.0334763775098842,
-6.00000000000005));
#136307=CARTESIAN_POINT('Ctrl Pts',(-20.878421006149,0.002555091943291,
-5.99999999999998));
#136308=CARTESIAN_POINT('Ctrl Pts',(-20.9027587660785,-0.0274968485461307,
-6.00000000000002));
#136309=CARTESIAN_POINT('Ctrl Pts',(-20.9161338002876,-0.044012161921713,
-6.00000000000003));
#136310=CARTESIAN_POINT('Ctrl Pts',(-20.9298620146726,-0.0602648435553045,
-5.99999999999998));
#136311=CARTESIAN_POINT('Ctrl Pts',(-20.9439348110724,-0.0762420159595881,
-5.99999999999999));
#136312=CARTESIAN_POINT('Ctrl Pts',(-20.9530636035687,-0.0866061459742095,
-5.99999999999999));
#136313=CARTESIAN_POINT('Ctrl Pts',(-20.9623391710389,-0.0968560195668169,
-6.00000000000001));
#136314=CARTESIAN_POINT('Ctrl Pts',(-20.9717431138342,-0.106971189160145,
-6.00000000000001));
#136315=CARTESIAN_POINT('Ctrl Pts',(-21.0128363116122,-0.151172294346014,
-6.00000000000001));
#136316=CARTESIAN_POINT('Ctrl Pts',(-21.0564377688707,-0.192874028286213,
-6.00000000000002));
#136317=CARTESIAN_POINT('Ctrl Pts',(-21.1023016041767,-0.231816412469469,
-6.00000000000002));
#136318=CARTESIAN_POINT('Ctrl Pts',(-21.1275553688095,-0.25325905453901,
-6.00000000000003));
#136319=CARTESIAN_POINT('Ctrl Pts',(-21.1534959236055,-0.273864748872313,
-6.00000000000004));
#136320=CARTESIAN_POINT('Ctrl Pts',(-21.1800879138415,-0.293586475167077,
-6.00000000000003));
#136321=CARTESIAN_POINT('Ctrl Pts',(-21.1924609844341,-0.302762859089012,
-6.00000000000002));
#136322=CARTESIAN_POINT('Ctrl Pts',(-21.2049751417566,-0.311747822082119,
-6.00000000000005));
#136323=CARTESIAN_POINT('Ctrl Pts',(-21.2176270836379,-0.3205363747662,
-6.00000000000002));
#136324=CARTESIAN_POINT('Ctrl Pts',(-21.2273289074436,-0.327275655617109,
-6.00000000000001));
#136325=CARTESIAN_POINT('Ctrl Pts',(-21.2371108740145,-0.333898730182812,
-6.00000000000006));
#136326=CARTESIAN_POINT('Ctrl Pts',(-21.2469630024738,-0.340398020720054,
-6.00000000000005));
#136327=CARTESIAN_POINT('Ctrl Pts',(-21.2977187567768,-0.373880774727412,
-6.00000000000003));
#136328=CARTESIAN_POINT('Ctrl Pts',(-21.3503919444321,-0.404121965629313,
-6.));
#136329=CARTESIAN_POINT('Ctrl Pts',(-21.4047548111353,-0.43084736906057,
-6.00000000000003));
#136330=CARTESIAN_POINT('Ctrl Pts',(-21.4148035193166,-0.435787428266307,
-6.00000000000003));
#136331=CARTESIAN_POINT('Ctrl Pts',(-21.4249100656712,-0.44060726441391,
-6.00000000000002));
#136332=CARTESIAN_POINT('Ctrl Pts',(-21.4350731491762,-0.445305004100473,
-6.00000000000002));
#136333=CARTESIAN_POINT('Ctrl Pts',(-21.4726735185508,-0.462685235932125,
-6.00000000000001));
#136334=CARTESIAN_POINT('Ctrl Pts',(-21.5110472512579,-0.478395093363263,
-6.00000000000004));
#136335=CARTESIAN_POINT('Ctrl Pts',(-21.5500883508879,-0.492459335223598,
-6.00000000000006));
#136336=CARTESIAN_POINT('Ctrl Pts',(-22.3494288790946,-0.495721457493081,
-6.00294356625675));
#136337=CARTESIAN_POINT('Ctrl Pts',(-22.8330683941797,-0.366577429477468,
-6.02867458008192));
#136338=CARTESIAN_POINT('Ctrl Pts',(-23.6580915401405,0.394190827129925,
-6.08012930878768));
#136339=CARTESIAN_POINT('Ctrl Pts',(-23.4156065885705,2.06872657277341,
-6.15730775237402));
#136340=CARTESIAN_POINT('Ctrl Pts',(-21.8972695958558,2.81191799254906,
-6.23447889701578));
#136341=CARTESIAN_POINT('Ctrl Pts',(-20.4258482304807,1.98173169021987,
-6.31165004165755));
#136342=CARTESIAN_POINT('Ctrl Pts',(-20.2783902012899,0.2978324463073,-6.3888211862993));
#136343=CARTESIAN_POINT('Ctrl Pts',(-21.5838352020395,-0.775593405817618,
-6.46599233094107));
#136344=CARTESIAN_POINT('Ctrl Pts',(-23.207351366242,-0.306155785057727,
-6.54316347558283));
#136345=CARTESIAN_POINT('Ctrl Pts',(-23.7382834590338,1.29840883098511,
-6.62033462022458));
#136346=CARTESIAN_POINT('Ctrl Pts',(-22.7151537867526,2.64362052392713,
-6.69750576486635));
#136347=CARTESIAN_POINT('Ctrl Pts',(-21.0271152873712,2.56053089525116,
-6.77467690950811));
#136348=CARTESIAN_POINT('Ctrl Pts',(-20.1410626558735,1.1213209453176,-6.85184805414987));
#136349=CARTESIAN_POINT('Ctrl Pts',(-20.8269929323425,-0.423313875344182,
-6.92901919879164));
#136350=CARTESIAN_POINT('Ctrl Pts',(-22.4888224346674,-0.731080747060635,
-7.0061903434334));
#136351=CARTESIAN_POINT('Ctrl Pts',(-23.6824124023475,0.465474331375493,
-7.08336148807515));
#136352=CARTESIAN_POINT('Ctrl Pts',(-23.3705233422915,2.12653612459561,
-7.16053263271692));
#136353=CARTESIAN_POINT('Ctrl Pts',(-21.8241899541753,2.80862907641399,
-7.23770377735867));
#136354=CARTESIAN_POINT('Ctrl Pts',(-20.3871859100543,1.91901317583765,
-7.31487492200044));
#136355=CARTESIAN_POINT('Ctrl Pts',(-20.3082791180656,0.23076311617535,
-7.3920460666422));
#136356=CARTESIAN_POINT('Ctrl Pts',(-21.6560376834298,-0.789003872540381,
-7.46921721128396));
#136357=CARTESIAN_POINT('Ctrl Pts',(-23.2592548439766,-0.254136074614078,
-7.54638835592573));
#136358=CARTESIAN_POINT('Ctrl Pts',(-23.724713747306,1.37062990962013,-7.62355950056747));
#136359=CARTESIAN_POINT('Ctrl Pts',(-22.6479475054437,2.67322381241457,
-7.70073064520925));
#136360=CARTESIAN_POINT('Ctrl Pts',(-20.9646324202764,2.5219623366835,-7.77790178985101));
#136361=CARTESIAN_POINT('Ctrl Pts',(-20.137664945086,1.04772174268297,-7.85507293449276));
#136362=CARTESIAN_POINT('Ctrl Pts',(-20.8855146423405,-0.467207615859468,
-7.93224407913453));
#136363=CARTESIAN_POINT('Ctrl Pts',(-22.5586407113732,-0.708723385526007,
-8.00941522377629));
#136364=CARTESIAN_POINT('Ctrl Pts',(-23.7023760809268,0.537950929960438,
-8.08658636841805));
#136365=CARTESIAN_POINT('Ctrl Pts',(-23.4496155782475,1.63112624023658,
-8.13803379817922));
#136366=CARTESIAN_POINT('Ctrl Pts',(-23.123028433054,2.01031205541452,-8.16375751305981));
#136367=CARTESIAN_POINT('Ctrl Pts',(-22.3249001525792,-0.403869950441567,
-5.94805471546504));
#136368=CARTESIAN_POINT('Ctrl Pts',(-22.7788396067957,-0.282656592632247,
-5.97378572929022));
#136369=CARTESIAN_POINT('Ctrl Pts',(-23.5531984937602,0.43139326561541,
-6.02524045799597));
#136370=CARTESIAN_POINT('Ctrl Pts',(-23.3256044218573,2.0030966081544,-6.10241890158232));
#136371=CARTESIAN_POINT('Ctrl Pts',(-21.9005077449073,2.70064901433409,
-6.17959004622408));
#136372=CARTESIAN_POINT('Ctrl Pts',(-20.5194456300734,1.92144403785305,
-6.25676119086584));
#136373=CARTESIAN_POINT('Ctrl Pts',(-20.3810429247468,0.340952204793195,
-6.33393233550761));
#136374=CARTESIAN_POINT('Ctrl Pts',(-21.6063212005416,-0.666555102316617,
-6.41110348014935));
#136375=CARTESIAN_POINT('Ctrl Pts',(-23.1301380486332,-0.225945411193953,
-6.48827462479113));
#136376=CARTESIAN_POINT('Ctrl Pts',(-23.6284658669989,1.28008369383731,
-6.56544576943288));
#136377=CARTESIAN_POINT('Ctrl Pts',(-22.6681660764697,2.54268660913492,
-6.64261691407464));
#136378=CARTESIAN_POINT('Ctrl Pts',(-21.0837891775504,2.46469947302274,
-6.71978805871641));
#136379=CARTESIAN_POINT('Ctrl Pts',(-20.2521485952495,1.11387068670934,
-6.79695920335817));
#136380=CARTESIAN_POINT('Ctrl Pts',(-20.8959562363107,-0.335908881718829,
-6.87413034799992));
#136381=CARTESIAN_POINT('Ctrl Pts',(-22.4557336195818,-0.624775943683584,
-6.95130149264168));
#136382=CARTESIAN_POINT('Ctrl Pts',(-23.576025823976,0.498299285497095,
-7.02847263728345));
#136383=CARTESIAN_POINT('Ctrl Pts',(-23.2832897151967,2.05735610429587,
-7.10564378192521));
#136384=CARTESIAN_POINT('Ctrl Pts',(-21.8319158874927,2.69756206889499,
-7.18281492656696));
#136385=CARTESIAN_POINT('Ctrl Pts',(-20.4831575434186,1.8625770360886,-7.25998607120874));
#136386=CARTESIAN_POINT('Ctrl Pts',(-20.4090963780835,0.278001568699366,
-7.3371572158505));
#136387=CARTESIAN_POINT('Ctrl Pts',(-21.674089763641,-0.679142038981393,
-7.41432836049225));
#136388=CARTESIAN_POINT('Ctrl Pts',(-23.1788541597446,-0.177120205165915,
-7.49149950513402));
#136389=CARTESIAN_POINT('Ctrl Pts',(-23.6157294644854,1.34786971213385,
-7.56867064977578));
#136390=CARTESIAN_POINT('Ctrl Pts',(-22.6050868993022,2.57047197447387,
-7.64584179441754));
#136391=CARTESIAN_POINT('Ctrl Pts',(-21.0251433520911,2.42849939035783,
-7.72301293905929));
#136392=CARTESIAN_POINT('Ctrl Pts',(-20.2489595361832,1.04479117431909,
-7.80018408370107));
#136393=CARTESIAN_POINT('Ctrl Pts',(-20.9508841573504,-0.377107129569758,
-7.87735522834283));
#136394=CARTESIAN_POINT('Ctrl Pts',(-22.5212643908144,-0.603791536545408,
-7.95452637298458));
#136395=CARTESIAN_POINT('Ctrl Pts',(-23.5947635430329,0.566325132391112,
-8.03169751762634));
#136396=CARTESIAN_POINT('Ctrl Pts',(-23.3575249364778,1.59236909329918,
-8.08314494738751));
#136397=CARTESIAN_POINT('Ctrl Pts',(-23.0509933446224,1.94826929710738,
-8.1088686622681));
#136398=CARTESIAN_POINT('Ctrl Pts',(-22.300371426064,-0.312018443390052,
-5.89316586467334));
#136399=CARTESIAN_POINT('Ctrl Pts',(-22.7246108194117,-0.198735755787229,
-5.91889687849851));
#136400=CARTESIAN_POINT('Ctrl Pts',(-23.4483054473798,0.468595704100783,
-5.97035160720427));
#136401=CARTESIAN_POINT('Ctrl Pts',(-23.2356022551438,1.9374666435354,-6.04753005079061));
#136402=CARTESIAN_POINT('Ctrl Pts',(-21.9037458939589,2.58938003611924,
-6.12470119543238));
#136403=CARTESIAN_POINT('Ctrl Pts',(-20.6130430296662,1.86115638548621,
-6.20187234007413));
#136404=CARTESIAN_POINT('Ctrl Pts',(-20.4836956482035,0.3840719632792,-6.2790434847159));
#136405=CARTESIAN_POINT('Ctrl Pts',(-21.6288071990437,-0.557516798815514,
-6.35621462935766));
#136406=CARTESIAN_POINT('Ctrl Pts',(-23.0529247310244,-0.145735037330184,
-6.43338577399942));
#136407=CARTESIAN_POINT('Ctrl Pts',(-23.5186482749642,1.2617585566895,-6.51055691864117));
#136408=CARTESIAN_POINT('Ctrl Pts',(-22.6211783661869,2.4417526943427,-6.58772806328294));
#136409=CARTESIAN_POINT('Ctrl Pts',(-21.1404630677295,2.36886805079411,
-6.6648992079247));
#136410=CARTESIAN_POINT('Ctrl Pts',(-20.3632345346257,1.10642042810096,
-6.74207035256646));
#136411=CARTESIAN_POINT('Ctrl Pts',(-20.9649195402789,-0.248503888093268,
-6.81924149720822));
#136412=CARTESIAN_POINT('Ctrl Pts',(-22.4226448044962,-0.518471140306853,
-6.89641264184999));
#136413=CARTESIAN_POINT('Ctrl Pts',(-23.4696392456045,0.531124239618692,
-6.97358378649174));
#136414=CARTESIAN_POINT('Ctrl Pts',(-23.1960560881021,1.98817608399623,
-7.05075493113352));
#136415=CARTESIAN_POINT('Ctrl Pts',(-21.8396418208102,2.586495061376,-7.12792607577527));
#136416=CARTESIAN_POINT('Ctrl Pts',(-20.579129176783,1.80614089633934,-7.20509722041702));
#136417=CARTESIAN_POINT('Ctrl Pts',(-20.5099136381014,0.325240021223374,
-7.2822683650588));
#136418=CARTESIAN_POINT('Ctrl Pts',(-21.6921418438521,-0.569280205422404,
-7.35943950970054));
#136419=CARTESIAN_POINT('Ctrl Pts',(-23.0984534755126,-0.100104335717859,
-7.43661065434232));
#136420=CARTESIAN_POINT('Ctrl Pts',(-23.5067451816648,1.32510951464757,
-7.51378179898406));
#136421=CARTESIAN_POINT('Ctrl Pts',(-22.5622262931607,2.46772013653318,
-7.59095294362584));
#136422=CARTESIAN_POINT('Ctrl Pts',(-21.0856542839059,2.33503644403196,
-7.66812408826759));
#136423=CARTESIAN_POINT('Ctrl Pts',(-20.3602541272804,1.04186060595509,
-7.74529523290936));
#136424=CARTESIAN_POINT('Ctrl Pts',(-21.0162536723602,-0.287006643279932,
-7.82246637755112));
#136425=CARTESIAN_POINT('Ctrl Pts',(-22.4838880702559,-0.49885968756481,
-7.89963752219288));
#136426=CARTESIAN_POINT('Ctrl Pts',(-23.4871510051389,0.594699334821902,
-7.97680866683464));
#136427=CARTESIAN_POINT('Ctrl Pts',(-23.2654342947082,1.55361194636178,
-8.02825609659581));
#136428=CARTESIAN_POINT('Ctrl Pts',(-22.978958256191,1.88622653880024,-8.0539798114764));
#136429=CARTESIAN_POINT('Ctrl Pts',(-22.2758426995487,-0.220166936338542,
-5.83827701388163));
#136430=CARTESIAN_POINT('Ctrl Pts',(-22.6703820320277,-0.114814918942012,
-5.86400802770681));
#136431=CARTESIAN_POINT('Ctrl Pts',(-23.3434124009993,0.505798142586267,
-5.91546275641256));
#136432=CARTESIAN_POINT('Ctrl Pts',(-23.1456000884306,1.87183667891629,
-5.99264119999891));
#136433=CARTESIAN_POINT('Ctrl Pts',(-21.9069840430104,2.47811105790429,
-6.06981234464067));
#136434=CARTESIAN_POINT('Ctrl Pts',(-20.706640429259,1.80086873311939,-6.14698348928243));
#136435=CARTESIAN_POINT('Ctrl Pts',(-20.5863483716603,0.427191721765094,
-6.2241546339242));
#136436=CARTESIAN_POINT('Ctrl Pts',(-21.6512931975458,-0.44847849531461,
-6.30132577856596));
#136437=CARTESIAN_POINT('Ctrl Pts',(-22.9757114134156,-0.0655246634663076,
-6.37849692320771));
#136438=CARTESIAN_POINT('Ctrl Pts',(-23.4088306829294,1.24343341954179,
-6.45566806784948));
#136439=CARTESIAN_POINT('Ctrl Pts',(-22.574190655904,2.34081877955049,-6.53283921249123));
#136440=CARTESIAN_POINT('Ctrl Pts',(-21.1971369579087,2.27303662856569,
-6.610010357133));
#136441=CARTESIAN_POINT('Ctrl Pts',(-20.4743204740017,1.09897016949269,
-6.68718150177476));
#136442=CARTESIAN_POINT('Ctrl Pts',(-21.0338828442468,-0.161098894467706,
-6.76435264641652));
#136443=CARTESIAN_POINT('Ctrl Pts',(-22.3895559894107,-0.412166336930007,
-6.84152379105829));
#136444=CARTESIAN_POINT('Ctrl Pts',(-23.3632526672331,0.56394919374029,
-6.91869493570004));
#136445=CARTESIAN_POINT('Ctrl Pts',(-23.1088224610074,1.91899606369649,
-6.99586608034181));
#136446=CARTESIAN_POINT('Ctrl Pts',(-21.8473677541276,2.47542805385689,
-7.07303722498357));
#136447=CARTESIAN_POINT('Ctrl Pts',(-20.6751008101473,1.74970475659019,
-7.15020836962532));
#136448=CARTESIAN_POINT('Ctrl Pts',(-20.6107308981193,0.372478473747391,
-7.22737951426709));
#136449=CARTESIAN_POINT('Ctrl Pts',(-21.7101939240631,-0.459418371863309,
-7.30455065890885));
#136450=CARTESIAN_POINT('Ctrl Pts',(-23.0180527912807,-0.0230884662698116,
-7.38172180355061));
#136451=CARTESIAN_POINT('Ctrl Pts',(-23.3977608988442,1.30234931716139,
-7.45889294819237));
#136452=CARTESIAN_POINT('Ctrl Pts',(-22.5193656870193,2.36496829859259,
-7.53606409283414));
#136453=CARTESIAN_POINT('Ctrl Pts',(-21.1461652157205,2.24157349770619,
-7.61323523747589));
#136454=CARTESIAN_POINT('Ctrl Pts',(-20.4715487183776,1.03893003759129,
-7.69040638211766));
#136455=CARTESIAN_POINT('Ctrl Pts',(-21.0816231873701,-0.196906156990209,
-7.76757752675942));
#136456=CARTESIAN_POINT('Ctrl Pts',(-22.4465117496972,-0.393927838584109,
-7.84474867140118));
#136457=CARTESIAN_POINT('Ctrl Pts',(-23.3795384672449,0.623073537252594,
-7.92191981604294));
#136458=CARTESIAN_POINT('Ctrl Pts',(-23.1733436529386,1.51485479942439,
-7.97336724580411));
#136459=CARTESIAN_POINT('Ctrl Pts',(-22.9069231677594,1.82418378049299,
-7.9990909606847));
#136460=CARTESIAN_POINT('Ctrl Pts',(-22.9081161737437,1.8252112989365,-8.));
#136461=CARTESIAN_POINT('Ctrl Pts',(-22.9458263014938,1.7899950512915,-8.));
#136462=CARTESIAN_POINT('Ctrl Pts',(-22.9810576730778,1.7524411352478,-8.));
#136463=CARTESIAN_POINT('Ctrl Pts',(-23.0138046909494,1.71289020318495,
-8.));
#136464=CARTESIAN_POINT('Ctrl Pts',(-23.046551708821,1.67333927112209,-8.));
#136465=CARTESIAN_POINT('Ctrl Pts',(-23.0768147826443,1.63179054638159,
-8.00000000000002));
#136466=CARTESIAN_POINT('Ctrl Pts',(-23.1045621698079,1.58853824094364,
-8.00000000000001));
#136467=CARTESIAN_POINT('Ctrl Pts',(-23.1267698135901,1.55392122326679,
-8.00000000000001));
#136468=CARTESIAN_POINT('Ctrl Pts',(-23.1473655883184,1.51821190695519,
-8.));
#136469=CARTESIAN_POINT('Ctrl Pts',(-23.1663184581739,1.48154480791058,
-8.));
#136470=CARTESIAN_POINT('Ctrl Pts',(-23.1734626007625,1.46772341907179,
-8.));
#136471=CARTESIAN_POINT('Ctrl Pts',(-23.1803731644546,1.45376581899129,
-8.00000000000001));
#136472=CARTESIAN_POINT('Ctrl Pts',(-23.1870479342029,1.43967880704949,
-8.00000000000001));
#136473=CARTESIAN_POINT('Ctrl Pts',(-23.1929663010849,1.4271881732021,-8.00000000000001));
#136474=CARTESIAN_POINT('Ctrl Pts',(-23.1987013567933,1.41459065047149,
-8.00000000000002));
#136475=CARTESIAN_POINT('Ctrl Pts',(-23.2042388080911,1.40192073735314,
-8.00000000000001));
#136476=CARTESIAN_POINT('Ctrl Pts',(-23.2260392040861,1.35204054728949,
-8.));
#136477=CARTESIAN_POINT('Ctrl Pts',(-23.2448162561212,1.30097015180589,
-8.00000000000002));
#136478=CARTESIAN_POINT('Ctrl Pts',(-23.2605389470064,1.24903997091589,
-8.00000000000001));
#136479=CARTESIAN_POINT('Ctrl Pts',(-23.2765523292268,1.19614967106579,
-8.));
#136480=CARTESIAN_POINT('Ctrl Pts',(-23.289397971074,1.14236657698248,-8.00000000000001));
#136481=CARTESIAN_POINT('Ctrl Pts',(-23.2990023606596,1.08800528941673,
-8.));
#136482=CARTESIAN_POINT('Ctrl Pts',(-23.305511272655,1.05116454763219,-8.));
#136483=CARTESIAN_POINT('Ctrl Pts',(-23.3105306914628,1.0140575372159,-7.99999999999998));
#136484=CARTESIAN_POINT('Ctrl Pts',(-23.3140252228657,0.976776843801469,
-8.));
#136485=CARTESIAN_POINT('Ctrl Pts',(-23.315417198095,0.961926840816698,
-8.00000000000001));
#136486=CARTESIAN_POINT('Ctrl Pts',(-23.3165671044889,0.947049248713289,
-7.99999999999999));
#136487=CARTESIAN_POINT('Ctrl Pts',(-23.3174722103952,0.932149828344294,
-7.99999999999999));
#136488=CARTESIAN_POINT('Ctrl Pts',(-23.3181970285803,0.920218218178783,
-8.));
#136489=CARTESIAN_POINT('Ctrl Pts',(-23.3187647796848,0.908270504603085,
-8.00000000000002));
#136490=CARTESIAN_POINT('Ctrl Pts',(-23.3191735821551,0.896332200675252,
-8.00000000000001));
#136491=CARTESIAN_POINT('Ctrl Pts',(-23.3211180629428,0.839547312335889,
-8.));
#136492=CARTESIAN_POINT('Ctrl Pts',(-23.3194782836048,0.782867486104685,
-7.99999999999999));
#136493=CARTESIAN_POINT('Ctrl Pts',(-23.3141922606772,0.726624469789134,
-7.99999999999999));
#136494=CARTESIAN_POINT('Ctrl Pts',(-23.3115256230824,0.698251580794284,
-7.99999999999999));
#136495=CARTESIAN_POINT('Ctrl Pts',(-23.3079303289237,0.66998945784058,
-8.00000000000002));
#136496=CARTESIAN_POINT('Ctrl Pts',(-23.3033936657804,0.641879012493639,
-8.00000000000001));
#136497=CARTESIAN_POINT('Ctrl Pts',(-23.294652936409,0.587718986164878,
-7.99999999999998));
#136498=CARTESIAN_POINT('Ctrl Pts',(-23.2824210905532,0.534121732388085,
-8.));
#136499=CARTESIAN_POINT('Ctrl Pts',(-23.2669229101663,0.481296104319126,
-8.00000000000001));
#136500=CARTESIAN_POINT('Ctrl Pts',(-23.258349314679,0.452072959722687,
-8.00000000000001));
#136501=CARTESIAN_POINT('Ctrl Pts',(-23.2487751754921,0.423085955886089,
-7.99999999999999));
#136502=CARTESIAN_POINT('Ctrl Pts',(-23.2382319859601,0.394371326985252,
-8.));
#136503=CARTESIAN_POINT('Ctrl Pts',(-23.2351171946824,0.385888118429588,
-8.00000000000001));
#136504=CARTESIAN_POINT('Ctrl Pts',(-23.2319184736363,0.377430703827278,
-8.));
#136505=CARTESIAN_POINT('Ctrl Pts',(-23.2286401046448,0.369008323085798,
-8.));
#136506=CARTESIAN_POINT('Ctrl Pts',(-23.2080228662233,0.316041060317681,
-8.00000000000002));
#136507=CARTESIAN_POINT('Ctrl Pts',(-23.1842258309568,0.264365440852388,
-7.99999999999999));
#136508=CARTESIAN_POINT('Ctrl Pts',(-23.1575249531342,0.214199037169825,
-8.));
#136509=CARTESIAN_POINT('Ctrl Pts',(-23.1301428741228,0.162752772425961,
-8.00000000000002));
#136510=CARTESIAN_POINT('Ctrl Pts',(-23.0997065813885,0.112892778633516,
-8.00000000000004));
#136511=CARTESIAN_POINT('Ctrl Pts',(-23.066458234878,0.0648591349457721,
-8.00000000000002));
#136512=CARTESIAN_POINT('Ctrl Pts',(-23.0445846382061,0.0332585093815861,
-8.00000000000001));
#136513=CARTESIAN_POINT('Ctrl Pts',(-23.0214928135711,0.00244848622698404,
-8.00000000000001));
#136514=CARTESIAN_POINT('Ctrl Pts',(-22.9972402439659,-0.0274982596333189,
-7.99999999999999));
#136515=CARTESIAN_POINT('Ctrl Pts',(-22.9838653736619,-0.0440133691011212,
-7.99999999999998));
#136516=CARTESIAN_POINT('Ctrl Pts',(-22.9701373308597,-0.060265851750123,
-8.00000000000002));
#136517=CARTESIAN_POINT('Ctrl Pts',(-22.9560647132586,-0.0762428306815151,
-8.00000000000001));
#136518=CARTESIAN_POINT('Ctrl Pts',(-22.9469359143498,-0.0866069741528238,
-8.));
#136519=CARTESIAN_POINT('Ctrl Pts',(-22.9376603395824,-0.0968568604488173,
-8.));
#136520=CARTESIAN_POINT('Ctrl Pts',(-22.928256388654,-0.106972041920554,
-8.));
#136521=CARTESIAN_POINT('Ctrl Pts',(-22.8871632797553,-0.151173065183216,
-8.00000000000001));
#136522=CARTESIAN_POINT('Ctrl Pts',(-22.8435619105751,-0.19287471672912,
-7.99999999999999));
#136523=CARTESIAN_POINT('Ctrl Pts',(-22.7976981582322,-0.231817022324734,
-8.));
#136524=CARTESIAN_POINT('Ctrl Pts',(-22.7724444422472,-0.25325961860342,
-8.));
#136525=CARTESIAN_POINT('Ctrl Pts',(-22.7465039347115,-0.273865268493912,
-7.99999999999998));
#136526=CARTESIAN_POINT('Ctrl Pts',(-22.71991198962,-0.293586952417093,
-7.99999999999999));
#136527=CARTESIAN_POINT('Ctrl Pts',(-22.7075388639141,-0.302763373076619,
-7.99999999999999));
#136528=CARTESIAN_POINT('Ctrl Pts',(-22.6950246492845,-0.311748370900717,
-7.99999999999998));
#136529=CARTESIAN_POINT('Ctrl Pts',(-22.6823726478889,-0.32053695648976,
-8.));
#136530=CARTESIAN_POINT('Ctrl Pts',(-22.6726708307602,-0.327276226233617,
-8.00000000000001));
#136531=CARTESIAN_POINT('Ctrl Pts',(-22.6628888705827,-0.333899289710013,
-8.00000000000002));
#136532=CARTESIAN_POINT('Ctrl Pts',(-22.6530367480453,-0.340398569322225,
-8.00000000000002));
#136533=CARTESIAN_POINT('Ctrl Pts',(-22.6022810630418,-0.373881241456408,
-8.00000000000001));
#136534=CARTESIAN_POINT('Ctrl Pts',(-22.5496079356719,-0.404122359348019,
-7.99999999999998));
#136535=CARTESIAN_POINT('Ctrl Pts',(-22.4952451157902,-0.430847702929976,
-8.00000000000002));
#136536=CARTESIAN_POINT('Ctrl Pts',(-22.4851965086495,-0.435787705655013,
-8.00000000000002));
#136537=CARTESIAN_POINT('Ctrl Pts',(-22.4750900639388,-0.440607487982115,
-8.00000000000002));
#136538=CARTESIAN_POINT('Ctrl Pts',(-22.4649270826171,-0.445305176587642,
-8.00000000000002));
#136539=CARTESIAN_POINT('Ctrl Pts',(-22.4273267498864,-0.46268537724355,
-8.00000000000001));
#136540=CARTESIAN_POINT('Ctrl Pts',(-22.3889530471574,-0.4783952106442,
-8.));
#136541=CARTESIAN_POINT('Ctrl Pts',(-22.3499119716047,-0.492459434737854,
-8.00000000000002));
#136542=CARTESIAN_POINT('',(-22.9090732202108,1.8254401058412,-5.99954788385073));
#136543=CARTESIAN_POINT('Ctrl Pts',(-22.900798095226,1.8336325761921,-6.00000000000001));
#136544=CARTESIAN_POINT('Ctrl Pts',(-22.9033489063661,1.83072325332144,
-5.99984929461692));
#136545=CARTESIAN_POINT('Ctrl Pts',(-22.9058863641674,1.8278022226256,-5.99969858923382));
#136546=CARTESIAN_POINT('Ctrl Pts',(-22.9084103617212,1.82486960717409,
-5.99954788385073));
#136547=CARTESIAN_POINT('Ctrl Pts',(-22.3485138628787,-0.490649428218507,
-6.));
#136548=CARTESIAN_POINT('Ctrl Pts',(-22.4044028679726,-0.470227815790022,
-6.));
#136549=CARTESIAN_POINT('Ctrl Pts',(-22.4588173702241,-0.446392867385509,
-6.00000000000003));
#136550=CARTESIAN_POINT('Ctrl Pts',(-22.5115730856902,-0.419418969216882,
-6.00000000000002));
#136551=CARTESIAN_POINT('Ctrl Pts',(-22.565456234803,-0.39186861634361,
-6.00000000000001));
#136552=CARTESIAN_POINT('Ctrl Pts',(-22.6176097455121,-0.361042932611707,
-6.));
#136553=CARTESIAN_POINT('Ctrl Pts',(-22.6678060374361,-0.327189985610635,
-6.00000000000003));
#136554=CARTESIAN_POINT('Ctrl Pts',(-22.7055462084096,-0.301737587459099,
-6.00000000000005));
#136555=CARTESIAN_POINT('Ctrl Pts',(-22.7421794219536,-0.274572932256311,
-6.00000000000003));
#136556=CARTESIAN_POINT('Ctrl Pts',(-22.7775935489668,-0.245789659304715,
-6.));
#136557=CARTESIAN_POINT('Ctrl Pts',(-22.79478021356,-0.231820983529406,
-5.99999999999999));
#136558=CARTESIAN_POINT('Ctrl Pts',(-22.8116795392235,-0.217470962941808,
-6.00000000000005));
#136559=CARTESIAN_POINT('Ctrl Pts',(-22.8282773830848,-0.202749708172314,
-6.00000000000002));
#136560=CARTESIAN_POINT('Ctrl Pts',(-22.8358955754876,-0.195992845523012,
-6.00000000000001));
#136561=CARTESIAN_POINT('Ctrl Pts',(-22.8434519976646,-0.189156144639804,
-6.00000000000003));
#136562=CARTESIAN_POINT('Ctrl Pts',(-22.8509394373616,-0.182245914402203,
-6.00000000000003));
#136563=CARTESIAN_POINT('Ctrl Pts',(-22.8944102507364,-0.142126281898408,
-6.00000000000003));
#136564=CARTESIAN_POINT('Ctrl Pts',(-22.9354415666047,-0.0996417229512457,
-6.00000000000002));
#136565=CARTESIAN_POINT('Ctrl Pts',(-22.9738282935603,-0.0550316376893066,
-6.00000000000001));
#136566=CARTESIAN_POINT('Ctrl Pts',(-23.0115902613443,-0.0111475992181314,
-6.00000000000001));
#136567=CARTESIAN_POINT('Ctrl Pts',(-23.0467935106165,0.03479427217587,
-6.00000000000001));
#136568=CARTESIAN_POINT('Ctrl Pts',(-23.0792001586263,0.082590657958306,
-6.00000000000003));
#136569=CARTESIAN_POINT('Ctrl Pts',(-23.1022939499262,0.116651562924882,
-6.00000000000003));
#136570=CARTESIAN_POINT('Ctrl Pts',(-23.1239666670789,0.151654784425088,
-6.00000000000001));
#136571=CARTESIAN_POINT('Ctrl Pts',(-23.144116612275,0.187530760613085,
-6.00000000000002));
#136572=CARTESIAN_POINT('Ctrl Pts',(-23.1568808693999,0.210256886178785,
-6.00000000000003));
#136573=CARTESIAN_POINT('Ctrl Pts',(-23.1690338052687,0.23333328147849,
-5.99999999999999));
#136574=CARTESIAN_POINT('Ctrl Pts',(-23.1805465357337,0.256742489999805,
-6.00000000000001));
#136575=CARTESIAN_POINT('Ctrl Pts',(-23.1851137868955,0.266029230025591,
-6.00000000000002));
#136576=CARTESIAN_POINT('Ctrl Pts',(-23.1895802294321,0.275368546163185,
-6.00000000000001));
#136577=CARTESIAN_POINT('Ctrl Pts',(-23.1939379823001,0.284745750340967,
-6.00000000000001));
#136578=CARTESIAN_POINT('Ctrl Pts',(-23.2174796042975,0.335403647389285,
-6.));
#136579=CARTESIAN_POINT('Ctrl Pts',(-23.2379015456237,0.387262745342791,
-6.00000000000002));
#136580=CARTESIAN_POINT('Ctrl Pts',(-23.254989552808,0.440133962889093,
-6.00000000000001));
#136581=CARTESIAN_POINT('Ctrl Pts',(-23.2645258105778,0.469639659702598,
-6.00000000000001));
#136582=CARTESIAN_POINT('Ctrl Pts',(-23.2730228982952,0.499460843070488,
-6.00000000000003));
#136583=CARTESIAN_POINT('Ctrl Pts',(-23.2804365582016,0.529565852679068,
-6.00000000000002));
#136584=CARTESIAN_POINT('Ctrl Pts',(-23.2933860024121,0.582150291040888,
-6.));
#136585=CARTESIAN_POINT('Ctrl Pts',(-23.3030321297007,0.635601394376387,
-5.99999999999998));
#136586=CARTESIAN_POINT('Ctrl Pts',(-23.3094241819638,0.689622624956746,
-5.99999999999999));
#136587=CARTESIAN_POINT('Ctrl Pts',(-23.3124570061112,0.715253969293792,
-6.));
#136588=CARTESIAN_POINT('Ctrl Pts',(-23.3147566567809,0.741013543589083,
-6.00000000000002));
#136589=CARTESIAN_POINT('Ctrl Pts',(-23.3163252005774,0.766868579593576,
-6.00000000000001));
#136590=CARTESIAN_POINT('Ctrl Pts',(-23.3172283381346,0.781755415466084,
-6.00000000000001));
#136591=CARTESIAN_POINT('Ctrl Pts',(-23.3178890663563,0.79668034899549,
-6.00000000000002));
#136592=CARTESIAN_POINT('Ctrl Pts',(-23.3183070192964,0.811601449950553,
-6.00000000000001));
#136593=CARTESIAN_POINT('Ctrl Pts',(-23.3198670669725,0.867295827560084,
-5.99999999999998));
#136594=CARTESIAN_POINT('Ctrl Pts',(-23.3180563498196,0.923011937479286,
-5.99999999999999));
#136595=CARTESIAN_POINT('Ctrl Pts',(-23.3129681477124,0.978431297783051,
-6.));
#136596=CARTESIAN_POINT('Ctrl Pts',(-23.3078908445592,1.03373194954259,
-6.00000000000002));
#136597=CARTESIAN_POINT('Ctrl Pts',(-23.2995496495147,1.08873825785068,
-6.));
#136598=CARTESIAN_POINT('Ctrl Pts',(-23.2879882369054,1.14311837677537,
-6.));
#136599=CARTESIAN_POINT('Ctrl Pts',(-23.2803755700282,1.17892522357717,
-6.));
#136600=CARTESIAN_POINT('Ctrl Pts',(-23.2713657489019,1.21446022763029,
-6.00000000000002));
#136601=CARTESIAN_POINT('Ctrl Pts',(-23.2609609427906,1.24962142831958,
-5.99999999999999));
#136602=CARTESIAN_POINT('Ctrl Pts',(-23.2551733467015,1.26917958494658,
-5.99999999999997));
#136603=CARTESIAN_POINT('Ctrl Pts',(-23.2489539947974,1.28862196500248,
-5.99999999999997));
#136604=CARTESIAN_POINT('Ctrl Pts',(-23.2423022650395,1.30792997183709,
-6.));
#136605=CARTESIAN_POINT('Ctrl Pts',(-23.2386072618587,1.31865547471599,
-6.00000000000001));
#136606=CARTESIAN_POINT('Ctrl Pts',(-23.2347819386265,1.32933040930559,
-6.00000000000001));
#136607=CARTESIAN_POINT('Ctrl Pts',(-23.2308275153244,1.33994985949573,
-6.00000000000001));
#136608=CARTESIAN_POINT('Ctrl Pts',(-23.2121715534761,1.39004972045208,
-6.));
#136609=CARTESIAN_POINT('Ctrl Pts',(-23.1906400792063,1.43893237474899,
-6.00000000000003));
#136610=CARTESIAN_POINT('Ctrl Pts',(-23.1662615812377,1.48628287293513,
-6.00000000000002));
#136611=CARTESIAN_POINT('Ctrl Pts',(-23.1528667473223,1.5122997366416,-6.00000000000001));
#136612=CARTESIAN_POINT('Ctrl Pts',(-23.138611706844,1.53785350946739,-6.));
#136613=CARTESIAN_POINT('Ctrl Pts',(-23.1234964888878,1.56288705326999,
-5.99999999999999));
#136614=CARTESIAN_POINT('Ctrl Pts',(-23.1168576664729,1.57388214789589,
-5.99999999999999));
#136615=CARTESIAN_POINT('Ctrl Pts',(-23.1100516986934,1.58477863417229,
-5.99999999999999));
#136616=CARTESIAN_POINT('Ctrl Pts',(-23.1030821447323,1.59556564650599,
-5.99999999999999));
#136617=CARTESIAN_POINT('Ctrl Pts',(-23.0751444036478,1.6388058250503,-5.99999999999998));
#136618=CARTESIAN_POINT('Ctrl Pts',(-23.0446406097003,1.68019930939369,
-5.99999999999999));
#136619=CARTESIAN_POINT('Ctrl Pts',(-23.0115864199713,1.7194450443779,-5.99999999999999));
#136620=CARTESIAN_POINT('Ctrl Pts',(-23.0020837523893,1.73072770405349,
-5.99999999999998));
#136621=CARTESIAN_POINT('Ctrl Pts',(-22.9923700884712,1.7418326038274,-6.00000000000002));
#136622=CARTESIAN_POINT('Ctrl Pts',(-22.9824453147852,1.75275193981372,
-6.00000000000001));
#136623=CARTESIAN_POINT('Ctrl Pts',(-22.9593362153627,1.77817680378731,
-5.99999999999997));
#136624=CARTESIAN_POINT('Ctrl Pts',(-22.9350827358701,1.8025961952395,-5.99999999999997));
#136625=CARTESIAN_POINT('Ctrl Pts',(-22.9097689137086,1.8259702051831,-6.00000000000002));
#136626=CARTESIAN_POINT('Origin',(-21.3427505978759,0.999999999999992,-8.00000000000001));
#136627=CARTESIAN_POINT('',(-17.5765008460949,-4.73438257217951,-8.00000000000001));
#136628=CARTESIAN_POINT('',(-17.2475487670954,-4.96527972955151,-8.00000000000001));
#136629=CARTESIAN_POINT('Origin',(-18.0333567745876,-5.73502369695961,-8.00000000000001));
#136630=CARTESIAN_POINT('',(-23.3621001638699,-2.09289074983501,-8.00000000000001));
#136631=CARTESIAN_POINT('',(-20.026783119352,-3.61567382106381,-8.00000000000001));
#136632=CARTESIAN_POINT('',(-23.3621001638699,4.09289074983499,-8.00000000000001));
#136633=CARTESIAN_POINT('Origin',(-21.9500000210213,0.999999999999992,-8.00000000000001));
#136634=CARTESIAN_POINT('',(-17.5765008460949,6.73438257217959,-8.00000000000001));
#136635=CARTESIAN_POINT('',(-23.1108487927725,4.20760288347129,-8.00000000000001));
#136636=CARTESIAN_POINT('',(-17.2475487670954,6.96527972955149,-8.00000000000001));
#136637=CARTESIAN_POINT('Origin',(-18.0333567745876,7.73502369695969,-8.00000000000001));
#136638=CARTESIAN_POINT('Origin',(-2.10213452200837E-8,0.999999999999992,
-8.00000000000001));
#136639=CARTESIAN_POINT('Ctrl Pts',(22.9063568733139,1.82409293608429,-6.00117200355571));
#136640=CARTESIAN_POINT('Ctrl Pts',(23.1728199782998,1.51487469222179,-6.02690203666603));
#136641=CARTESIAN_POINT('Ctrl Pts',(23.3790636548542,0.62330421389329,-6.07835578465692));
#136642=CARTESIAN_POINT('Ctrl Pts',(22.4463190818302,-0.39338932020661,
-6.1555332475284));
#136643=CARTESIAN_POINT('Ctrl Pts',(21.0819593047411,-0.196442803679409,
-6.23270439217017));
#136644=CARTESIAN_POINT('Ctrl Pts',(20.4721203926454,1.03891473966289,-6.30987553681192));
#136645=CARTESIAN_POINT('Ctrl Pts',(21.1464761479847,2.24109341156569,-6.38704668145369));
#136646=CARTESIAN_POINT('Ctrl Pts',(22.5191453930256,2.36444026682549,-6.46421782609544));
#136647=CARTESIAN_POINT('Ctrl Pts',(23.3972008937867,1.30223241594259,-6.54138897073721));
#136648=CARTESIAN_POINT('Ctrl Pts',(23.0176396334798,-0.0226927722025083,
-6.61856011537897));
#136649=CARTESIAN_POINT('Ctrl Pts',(21.7102866388558,-0.45885387376241,
-6.69573126002073));
#136650=CARTESIAN_POINT('Ctrl Pts',(20.6112488676729,0.37272118441749,-6.77290240466248));
#136651=CARTESIAN_POINT('Ctrl Pts',(20.6755938840128,1.74941478365189,-6.85007354930426));
#136652=CARTESIAN_POINT('Ctrl Pts',(21.8474074087956,2.47485737455439,-6.92724469394601));
#136653=CARTESIAN_POINT('Ctrl Pts',(23.1083742006497,1.91864060809139,-7.00441583858777));
#136654=CARTESIAN_POINT('Ctrl Pts',(23.3627059966256,0.564117852774593,
-7.08158698322954));
#136655=CARTESIAN_POINT('Ctrl Pts',(22.3893859320526,-0.411620128968209,
-7.1587581278713));
#136656=CARTESIAN_POINT('Ctrl Pts',(21.0342371459635,-0.16064979403871,
-7.23592927251305));
#136657=CARTESIAN_POINT('Ctrl Pts',(20.4748912050807,1.09893188571729,-7.31310041715483));
#136658=CARTESIAN_POINT('Ctrl Pts',(21.1974281169335,2.27254424007929,-7.39027156179657));
#136659=CARTESIAN_POINT('Ctrl Pts',(22.5739491795643,2.34030015500749,-7.46744270643835));
#136660=CARTESIAN_POINT('Ctrl Pts',(23.4082663916087,1.24333928571779,-7.5446138510801));
#136661=CARTESIAN_POINT('Ctrl Pts',(22.9753146249661,-0.0651125751728099,
-7.62178499572186));
#136662=CARTESIAN_POINT('Ctrl Pts',(21.6514087126462,-0.447918160579306,
-7.69895614036363));
#136663=CARTESIAN_POINT('Ctrl Pts',(20.5868757451666,0.42741312763809,-7.77612728500538));
#136664=CARTESIAN_POINT('Ctrl Pts',(20.7071213310053,1.80055923895449,-7.85329842964714));
#136665=CARTESIAN_POINT('Ctrl Pts',(21.9070006438952,2.47753884950259,-7.9304695742889));
#136666=CARTESIAN_POINT('Ctrl Pts',(23.1451374810536,1.87150031592389,-8.00764071893066));
#136667=CARTESIAN_POINT('Ctrl Pts',(23.3428805758158,0.505941210960477,
-8.08482174569748));
#136668=CARTESIAN_POINT('Ctrl Pts',(22.6700359089709,-0.114446174087646,
-8.13627905758372));
#136669=CARTESIAN_POINT('Ctrl Pts',(22.2755978923469,-0.219726881556652,
-8.16201265458937));
#136670=CARTESIAN_POINT('Ctrl Pts',(22.9784824811563,1.88624358746325,-5.94620290068195));
#136671=CARTESIAN_POINT('Ctrl Pts',(23.2650414452598,1.55370501838886,-5.97193293379227));
#136672=CARTESIAN_POINT('Ctrl Pts',(23.4868394097826,0.594894932059846,
-6.02338668178316));
#136673=CARTESIAN_POINT('Ctrl Pts',(22.4837500003388,-0.498474620763636,
-6.10056414465465));
#136674=CARTESIAN_POINT('Ctrl Pts',(21.0164942449583,-0.286674980573953,
-6.17773528929641));
#136675=CARTESIAN_POINT('Ctrl Pts',(20.3606630861593,1.04184957420938,-6.25490643393818));
#136676=CARTESIAN_POINT('Ctrl Pts',(21.0858767576635,2.33469300522009,-6.33207757857993));
#136677=CARTESIAN_POINT('Ctrl Pts',(22.5620686564872,2.46734231541453,-6.4092487232217));
#136678=CARTESIAN_POINT('Ctrl Pts',(23.5063445056212,1.32502589067852,-6.48641986786346));
#136679=CARTESIAN_POINT('Ctrl Pts',(23.0981578578932,-0.0998212357164752,
-6.5635910125052));
#136680=CARTESIAN_POINT('Ctrl Pts',(21.6922081678721,-0.568876317289018,
-6.64076215714698));
#136681=CARTESIAN_POINT('Ctrl Pts',(20.5102842191986,0.325413671784407,
-6.71793330178873));
#136682=CARTESIAN_POINT('Ctrl Pts',(20.5794819463231,1.80593342968993,-6.79510444643051));
#136683=CARTESIAN_POINT('Ctrl Pts',(21.8396701806453,2.58608675476861,-6.87227559107226));
#136684=CARTESIAN_POINT('Ctrl Pts',(23.1957353577051,1.98792176519896,-6.94944673571402));
#136685=CARTESIAN_POINT('Ctrl Pts',(23.4692481053602,0.531244910672686,
-7.02661788035579));
#136686=CARTESIAN_POINT('Ctrl Pts',(22.4225231208266,-0.518080343191016,
-7.10378902499754));
#136687=CARTESIAN_POINT('Ctrl Pts',(20.9651730221392,-0.248182568030355,
-7.18096016963931));
#136688=CARTESIAN_POINT('Ctrl Pts',(20.3636428650717,1.10639303587442,-7.25813131428107));
#136689=CARTESIAN_POINT('Ctrl Pts',(21.1406713733825,2.3685157621811,-7.33530245892283));
#136690=CARTESIAN_POINT('Ctrl Pts',(22.6210055824841,2.44138162777535,-7.41247360356459));
#136691=CARTESIAN_POINT('Ctrl Pts',(23.5182445305545,1.26169121479189,-7.48964474820635));
#136692=CARTESIAN_POINT('Ctrl Pts',(23.0526408224449,-0.145440214739043,
-7.56681589284811));
#136693=CARTESIAN_POINT('Ctrl Pts',(21.6288898426426,-0.557115864968094,
-7.64398703748988));
#136694=CARTESIAN_POINT('Ctrl Pts',(20.4840729478942,0.384230319571,-7.72115818213162));
#136695=CARTESIAN_POINT('Ctrl Pts',(20.6133871001022,1.86093504851414,-7.79832932677341));
#136696=CARTESIAN_POINT('Ctrl Pts',(21.9037577612453,2.58897045862498,-7.87550047141513));
#136697=CARTESIAN_POINT('Ctrl Pts',(23.2352712159626,1.93722629164813,-7.95267161605693));
#136698=CARTESIAN_POINT('Ctrl Pts',(23.4479275099613,0.468680758633138,
-8.02985264282373));
#136699=CARTESIAN_POINT('Ctrl Pts',(22.7243388887756,-0.198494407743786,
-8.08130995470997));
#136700=CARTESIAN_POINT('Ctrl Pts',(22.3001535237779,-0.311715074725019,
-8.10704355171562));
#136701=CARTESIAN_POINT('Ctrl Pts',(23.0506080889988,1.94839423884221,-5.8912337978082));
#136702=CARTESIAN_POINT('Ctrl Pts',(23.3572629122198,1.59253534455582,-5.91696383091851));
#136703=CARTESIAN_POINT('Ctrl Pts',(23.5946151647109,0.5664856502263,-5.96841757890941));
#136704=CARTESIAN_POINT('Ctrl Pts',(22.5211809188473,-0.603559921320658,
-6.04559504178089));
#136705=CARTESIAN_POINT('Ctrl Pts',(20.9510291851757,-0.376907157468498,
-6.12276618642265));
#136706=CARTESIAN_POINT('Ctrl Pts',(20.249205779673,1.04478440875577,-6.19993733106441));
#136707=CARTESIAN_POINT('Ctrl Pts',(21.0252773673422,2.42829259887449,-6.27710847570617));
#136708=CARTESIAN_POINT('Ctrl Pts',(22.6049919199487,2.57024436400366,-6.35427962034794));
#136709=CARTESIAN_POINT('Ctrl Pts',(23.6154881174555,1.34781936541443,-6.43145076498969));
#136710=CARTESIAN_POINT('Ctrl Pts',(23.1786760823068,-0.176949699230544,
-6.50862190963147));
#136711=CARTESIAN_POINT('Ctrl Pts',(21.6741296968885,-0.678898760815727,
-6.58579305427322));
#136712=CARTESIAN_POINT('Ctrl Pts',(20.4093195707243,0.27810615915123,-6.66296419891498));
#136713=CARTESIAN_POINT('Ctrl Pts',(20.4833700086334,1.86245207572798,-6.74013534355674));
#136714=CARTESIAN_POINT('Ctrl Pts',(21.8319329524951,2.69731613498273,-6.8173064881985));
#136715=CARTESIAN_POINT('Ctrl Pts',(23.2830965147605,2.05720292230642,-6.89447763284026));
#136716=CARTESIAN_POINT('Ctrl Pts',(23.5757902140948,0.498371968570677,
-6.97164877748203));
#136717=CARTESIAN_POINT('Ctrl Pts',(22.4556603096006,-0.624540557413726,
-7.04881992212377));
#136718=CARTESIAN_POINT('Ctrl Pts',(20.8961088983147,-0.335715342022009,
-7.12599106676556));
#136719=CARTESIAN_POINT('Ctrl Pts',(20.2523945250627,1.11385418603145,-7.2031622114073));
#136720=CARTESIAN_POINT('Ctrl Pts',(21.0839146298315,2.46448728428302,-7.28033335604907));
#136721=CARTESIAN_POINT('Ctrl Pts',(22.668061985404,2.54246310054321,-7.35750450069083));
#136722=CARTESIAN_POINT('Ctrl Pts',(23.6282226695004,1.28004314386601,-7.43467564533259));
#136723=CARTESIAN_POINT('Ctrl Pts',(23.1299670199237,-0.225767854305383,
-7.51184678997435));
#136724=CARTESIAN_POINT('Ctrl Pts',(21.606370972639,-0.666313569356887,
-7.58901793461611));
#136725=CARTESIAN_POINT('Ctrl Pts',(20.3812701506218,0.341047511504016,
-7.66618907925788));
#136726=CARTESIAN_POINT('Ctrl Pts',(20.5196528691991,1.92131085807378,-7.74336022389963));
#136727=CARTESIAN_POINT('Ctrl Pts',(21.9005148785954,2.70040206774737,-7.8205313685414));
#136728=CARTESIAN_POINT('Ctrl Pts',(23.3254049508715,2.00295226737237,-7.89770251318316));
#136729=CARTESIAN_POINT('Ctrl Pts',(23.5529744441067,0.431420306305785,
-7.97488353994999));
#136730=CARTESIAN_POINT('Ctrl Pts',(22.7786418685801,-0.282542641399823,
-8.02634085183622));
#136731=CARTESIAN_POINT('Ctrl Pts',(22.3247091552089,-0.403703267893301,
-8.05207444884186));
#136732=CARTESIAN_POINT('Ctrl Pts',(23.122733696841,2.01054489022106,-5.83626469493445));
#136733=CARTESIAN_POINT('Ctrl Pts',(23.4494843791796,1.63136567072288,-5.86199472804476));
#136734=CARTESIAN_POINT('Ctrl Pts',(23.7023909196395,0.538076368392755,
-5.91344847603567));
#136735=CARTESIAN_POINT('Ctrl Pts',(22.5586118373558,-0.708645221877573,
-5.99062593890713));
#136736=CARTESIAN_POINT('Ctrl Pts',(20.885564125393,-0.467139334363051,
-6.06779708354891));
#136737=CARTESIAN_POINT('Ctrl Pts',(20.1377484731868,1.04771924330226,-6.14496822819066));
#136738=CARTESIAN_POINT('Ctrl Pts',(20.964677977021,2.52189219252879,-6.22213937283243));
#136739=CARTESIAN_POINT('Ctrl Pts',(22.6479151834103,2.6731464125927,-6.29931051747418));
#136740=CARTESIAN_POINT('Ctrl Pts',(23.72463172929,1.37061284015026,-6.37648166211595));
#136741=CARTESIAN_POINT('Ctrl Pts',(23.2591943067203,-0.254078162744511,
-6.4536528067577));
#136742=CARTESIAN_POINT('Ctrl Pts',(21.6560512259048,-0.78892120434233,
-6.53082395139948));
#136743=CARTESIAN_POINT('Ctrl Pts',(20.3083549222499,0.230798646518151,
-6.60799509604123));
#136744=CARTESIAN_POINT('Ctrl Pts',(20.3872580709438,1.91897072176602,-6.685166240683));
#136745=CARTESIAN_POINT('Ctrl Pts',(21.8241957243447,2.80854551519707,-6.76233738532475));
#136746=CARTESIAN_POINT('Ctrl Pts',(23.3704576718158,2.12648407941399,-6.83950852996651));
#136747=CARTESIAN_POINT('Ctrl Pts',(23.6823323228293,0.465499026468774,
-6.91667967460828));
#136748=CARTESIAN_POINT('Ctrl Pts',(22.4887974983745,-0.731000771636436,
-6.99385081925003));
#136749=CARTESIAN_POINT('Ctrl Pts',(20.8270447744904,-0.423248116013548,
-7.0710219638918));
#136750=CARTESIAN_POINT('Ctrl Pts',(20.1411461850536,1.12131533618847,-7.14819310853356));
#136751=CARTESIAN_POINT('Ctrl Pts',(21.0271578862804,2.56045880638504,-7.22536425317532));
#136752=CARTESIAN_POINT('Ctrl Pts',(22.7151183883238,2.64354457331116,-7.30253539781708));
#136753=CARTESIAN_POINT('Ctrl Pts',(23.7382008084462,1.29839507294001,-7.37970654245884));
#136754=CARTESIAN_POINT('Ctrl Pts',(23.2072932174024,-0.306095493871621,
-7.4568776871006));
#136755=CARTESIAN_POINT('Ctrl Pts',(21.5838521026352,-0.775511273745666,
-7.53404883174237));
#136756=CARTESIAN_POINT('Ctrl Pts',(20.2784673533496,0.297864703436921,
-7.61121997638412));
#136757=CARTESIAN_POINT('Ctrl Pts',(20.4259186382961,1.98168666763342,-7.68839112102589));
#136758=CARTESIAN_POINT('Ctrl Pts',(21.8972719959456,2.81183367686976,-7.76556226566763));
#136759=CARTESIAN_POINT('Ctrl Pts',(23.4155386857805,2.06867824309672,-7.84273341030942));
#136760=CARTESIAN_POINT('Ctrl Pts',(23.658021378252,0.394159853978335,-7.91991443707622));
#136761=CARTESIAN_POINT('Ctrl Pts',(22.8329448483847,-0.36659087505587,
-7.97137174896246));
#136762=CARTESIAN_POINT('Ctrl Pts',(22.3492647866401,-0.495691461061565,
-7.99710534596811));
#136763=CARTESIAN_POINT('Ctrl Pts',(22.3485138208359,-0.490649428218493,
-8.00000000000001));
#136764=CARTESIAN_POINT('Ctrl Pts',(22.4946838404348,-0.4372395046764,-8.00000000000001));
#136765=CARTESIAN_POINT('Ctrl Pts',(22.6317792133684,-0.360071372937282,
-8.));
#136766=CARTESIAN_POINT('Ctrl Pts',(22.8736371924913,-0.171118184548593,
-8.));
#136767=CARTESIAN_POINT('Ctrl Pts',(22.9793712212907,-0.060188077426786,
-7.99999999999999));
#136768=CARTESIAN_POINT('Ctrl Pts',(23.1641105979564,0.203461914247813,
-7.99999999999999));
#136769=CARTESIAN_POINT('Ctrl Pts',(23.238050538628,0.3598842296734,-8.));
#136770=CARTESIAN_POINT('Ctrl Pts',(23.3194606150182,0.685726918729976,
-8.));
#136771=CARTESIAN_POINT('Ctrl Pts',(23.3284814781232,0.853393148949051,
-7.99999999999999));
#136772=CARTESIAN_POINT('Ctrl Pts',(23.2899438559561,1.17524600463165,-7.99999999999999));
#136773=CARTESIAN_POINT('Ctrl Pts',(23.2442379373553,1.33069545188236,-7.99999999999999));
#136774=CARTESIAN_POINT('Ctrl Pts',(23.0995280621159,1.61978829999637,-7.99999999999999));
#136775=CARTESIAN_POINT('Ctrl Pts',(23.0071789540993,1.73842050470344,-8.00000000000001));
#136776=CARTESIAN_POINT('Ctrl Pts',(22.8985126966394,1.83623195014015,-8.00000000000001));
#136777=CARTESIAN_POINT('Ctrl Pts',(22.908116131701,1.82521129893649,-6.));
#136778=CARTESIAN_POINT('Ctrl Pts',(22.9450075044187,1.79075965967929,-5.99999999999999));
#136779=CARTESIAN_POINT('Ctrl Pts',(22.9795265199656,1.75407059764649,-5.99999999999999));
#136780=CARTESIAN_POINT('Ctrl Pts',(23.0116681749775,1.71546357193199,-6.));
#136781=CARTESIAN_POINT('Ctrl Pts',(23.045222326383,1.67515992279949,-6.00000000000001));
#136782=CARTESIAN_POINT('Ctrl Pts',(23.0761861970359,1.63276557070519,-6.00000000000003));
#136783=CARTESIAN_POINT('Ctrl Pts',(23.1045263085396,1.58859440245256,-6.));
#136784=CARTESIAN_POINT('Ctrl Pts',(23.1267477757339,1.55395981161368,-5.99999999999998));
#136785=CARTESIAN_POINT('Ctrl Pts',(23.1473556422849,1.51823166591899,-5.99999999999999));
#136786=CARTESIAN_POINT('Ctrl Pts',(23.1663188241877,1.48154470230262,-5.99999999999999));
#136787=CARTESIAN_POINT('Ctrl Pts',(23.1734630474769,1.46772318958289,-5.99999999999999));
#136788=CARTESIAN_POINT('Ctrl Pts',(23.1803736876164,1.45376546342369,-6.00000000000003));
#136789=CARTESIAN_POINT('Ctrl Pts',(23.1870485294143,1.43967832332659,-6.00000000000002));
#136790=CARTESIAN_POINT('Ctrl Pts',(23.1929667679057,1.42718798164059,-6.00000000000001));
#136791=CARTESIAN_POINT('Ctrl Pts',(23.1987017036428,1.41459075646318,-5.99999999999998));
#136792=CARTESIAN_POINT('Ctrl Pts',(23.2042390439871,1.40192114455257,-5.99999999999998));
#136793=CARTESIAN_POINT('Ctrl Pts',(23.2260395195741,1.35204095876289,-5.99999999999999));
#136794=CARTESIAN_POINT('Ctrl Pts',(23.2448166472336,1.3009705679638,-6.00000000000002));
#136795=CARTESIAN_POINT('Ctrl Pts',(23.2605394064777,1.24904038991027,-6.00000000000002));
#136796=CARTESIAN_POINT('Ctrl Pts',(23.2765528398699,1.19615015389059,-6.00000000000003));
#136797=CARTESIAN_POINT('Ctrl Pts',(23.2893985326549,1.14236712377669,-6.));
#136798=CARTESIAN_POINT('Ctrl Pts',(23.2990029696711,1.0880058968445,-6.));
#136799=CARTESIAN_POINT('Ctrl Pts',(23.3055119128261,1.05116520172179,-6.));
#136800=CARTESIAN_POINT('Ctrl Pts',(23.3105313616353,1.01405823651869,-6.00000000000003));
#136801=CARTESIAN_POINT('Ctrl Pts',(23.3140259208794,0.976777585749033,
-6.00000000000001));
#136802=CARTESIAN_POINT('Ctrl Pts',(23.315417909761,0.96192757241519,-6.));
#136803=CARTESIAN_POINT('Ctrl Pts',(23.3165678285733,0.947049969453592,
-6.));
#136804=CARTESIAN_POINT('Ctrl Pts',(23.3174729455847,0.932150537677407,
-6.));
#136805=CARTESIAN_POINT('Ctrl Pts',(23.3181977694971,0.920218970493191,
-5.99999999999999));
#136806=CARTESIAN_POINT('Ctrl Pts',(23.318765526856,0.90827129975029,-6.00000000000003));
#136807=CARTESIAN_POINT('Ctrl Pts',(23.3191743360792,0.89633303825873,-6.00000000000003));
#136808=CARTESIAN_POINT('Ctrl Pts',(23.321118854114,0.839548202064488,-6.00000000000002));
#136809=CARTESIAN_POINT('Ctrl Pts',(23.3194791044103,0.78286841978709,-6.));
#136810=CARTESIAN_POINT('Ctrl Pts',(23.3141931001774,0.726625435644048,
-6.));
#136811=CARTESIAN_POINT('Ctrl Pts',(23.3115264726282,0.69825256941879,-6.));
#136812=CARTESIAN_POINT('Ctrl Pts',(23.3079311861598,0.669990466186293,
-5.99999999999998));
#136813=CARTESIAN_POINT('Ctrl Pts',(23.3033945279323,0.641880037021434,
-5.99999999999999));
#136814=CARTESIAN_POINT('Ctrl Pts',(23.294653812508,0.587720069603197,-5.99999999999998));
#136815=CARTESIAN_POINT('Ctrl Pts',(23.2824219738809,0.534122861038484,
-6.));
#136816=CARTESIAN_POINT('Ctrl Pts',(23.2669237959758,0.481297266457223,
-6.));
#136817=CARTESIAN_POINT('Ctrl Pts',(23.2583502098308,0.45207416755008,-5.99999999999999));
#136818=CARTESIAN_POINT('Ctrl Pts',(23.2487760803925,0.423087205372294,
-6.));
#136819=CARTESIAN_POINT('Ctrl Pts',(23.238232901264,0.394372614307267,-6.));
#136820=CARTESIAN_POINT('Ctrl Pts',(23.2351181252019,0.385889449998696,
-6.));
#136821=CARTESIAN_POINT('Ctrl Pts',(23.2319194199829,0.377432078840496,
-6.));
#136822=CARTESIAN_POINT('Ctrl Pts',(23.2286410675058,0.369009740971795,
-6.));
#136823=CARTESIAN_POINT('Ctrl Pts',(23.2077852194334,0.315429474593194,
-5.99999999999999));
#136824=CARTESIAN_POINT('Ctrl Pts',(23.1836756483089,0.263170910526294,
-6.00000000000001));
#136825=CARTESIAN_POINT('Ctrl Pts',(23.1565976811258,0.212459265016296,
-5.99999999999999));
#136826=CARTESIAN_POINT('Ctrl Pts',(23.1295197139427,0.161747619506298,
-5.99999999999998));
#136827=CARTESIAN_POINT('Ctrl Pts',(23.0994728236393,0.112582008396492,
-6.00000000000002));
#136828=CARTESIAN_POINT('Ctrl Pts',(23.0666892022875,0.0651929005834847,
-6.));
#136829=CARTESIAN_POINT('Ctrl Pts',(23.0447474031548,0.0334757734987984,
-5.99999999999999));
#136830=CARTESIAN_POINT('Ctrl Pts',(23.0215785960864,0.00255455394179094,
-5.99999999999999));
#136831=CARTESIAN_POINT('Ctrl Pts',(22.9972408872701,-0.0274973225056871,
-6.));
#136832=CARTESIAN_POINT('Ctrl Pts',(22.9838659081576,-0.0440125673387116,
-6.00000000000001));
#136833=CARTESIAN_POINT('Ctrl Pts',(22.9701377514496,-0.0602651820845042,
-5.99999999999998));
#136834=CARTESIAN_POINT('Ctrl Pts',(22.956065015152,-0.0762422894537602,
-5.99999999999998));
#136835=CARTESIAN_POINT('Ctrl Pts',(22.9469362204977,-0.0866064239944117,
-5.99999999999998));
#136836=CARTESIAN_POINT('Ctrl Pts',(22.9376606505719,-0.0968563018597042,
-6.));
#136837=CARTESIAN_POINT('Ctrl Pts',(22.9282567050398,-0.106971475448321,
-6.));
#136838=CARTESIAN_POINT('Ctrl Pts',(22.8871635371534,-0.151172553076501,
-6.));
#136839=CARTESIAN_POINT('Ctrl Pts',(22.8435621095159,-0.192874259302599,
-6.));
#136840=CARTESIAN_POINT('Ctrl Pts',(22.7976983021094,-0.231816617053861,
-6.));
#136841=CARTESIAN_POINT('Ctrl Pts',(22.7724445538394,-0.253259243719703,
-6.));
#136842=CARTESIAN_POINT('Ctrl Pts',(22.7465040149394,-0.273864923103498,
-5.99999999999998));
#136843=CARTESIAN_POINT('Ctrl Pts',(22.7199120398876,-0.293586635146076,
-5.99999999999999));
#136844=CARTESIAN_POINT('Ctrl Pts',(22.7075389507337,-0.302763031442103,
-5.99999999999999));
#136845=CARTESIAN_POINT('Ctrl Pts',(22.6950247741115,-0.311748006167511,
-6.));
#136846=CARTESIAN_POINT('Ctrl Pts',(22.6823728121875,-0.320536569935376,
-6.00000000000001));
#136847=CARTESIAN_POINT('Ctrl Pts',(22.6726709906612,-0.327275847026208,
-6.00000000000002));
#136848=CARTESIAN_POINT('Ctrl Pts',(22.6628890262749,-0.333898917838801,
-6.));
#136849=CARTESIAN_POINT('Ctrl Pts',(22.653036899842,-0.340398204679071,
-6.));
#136850=CARTESIAN_POINT('Ctrl Pts',(22.6022811687816,-0.373880931194739,
-5.99999999999999));
#136851=CARTESIAN_POINT('Ctrl Pts',(22.5496080013315,-0.404122097580018,
-6.00000000000001));
#136852=CARTESIAN_POINT('Ctrl Pts',(22.4952451503003,-0.430847480914457,
-6.));
#136853=CARTESIAN_POINT('Ctrl Pts',(22.4851964761634,-0.435787521092942,
-6.));
#136854=CARTESIAN_POINT('Ctrl Pts',(22.4750899640567,-0.440607339109571,
-6.));
#136855=CARTESIAN_POINT('Ctrl Pts',(22.4649269149819,-0.445305061588132,
-6.));
#136856=CARTESIAN_POINT('Ctrl Pts',(22.4273265579104,-0.462685282948391,
-6.00000000000001));
#136857=CARTESIAN_POINT('Ctrl Pts',(22.3889528352634,-0.478395132310893,
-5.99999999999998));
#136858=CARTESIAN_POINT('Ctrl Pts',(22.3499117437079,-0.492459368208522,
-6.));
#136859=CARTESIAN_POINT('Ctrl Pts',(21.5505711827703,-0.495721263066522,
-6.00294344809566));
#136860=CARTESIAN_POINT('Ctrl Pts',(21.0669317275038,-0.366577253429168,
-6.02867446208544));
#136861=CARTESIAN_POINT('Ctrl Pts',(20.2419081461725,0.39418733824399,-6.0801291909558));
#136862=CARTESIAN_POINT('Ctrl Pts',(20.4843940653702,2.0687275523926,-6.15730763470675));
#136863=CARTESIAN_POINT('Ctrl Pts',(22.0027303798341,2.8119166544984,-6.23447877934852));
#136864=CARTESIAN_POINT('Ctrl Pts',(23.474151242975,1.98173179924762,-6.31164992399027));
#136865=CARTESIAN_POINT('Ctrl Pts',(23.6216093115122,0.297832438268553,
-6.38882106863204));
#136866=CARTESIAN_POINT('Ctrl Pts',(22.3161646492079,-0.775592716702653,
-6.4659922132738));
#136867=CARTESIAN_POINT('Ctrl Pts',(20.6926490543717,-0.306155437729512,
-6.54316335791556));
#136868=CARTESIAN_POINT('Ctrl Pts',(20.161717095599,1.29840877217903,-6.62033450255732));
#136869=CARTESIAN_POINT('Ctrl Pts',(21.1848464639594,2.64361998303321,-6.69750564719908));
#136870=CARTESIAN_POINT('Ctrl Pts',(22.872884415153,2.56053040974976,-6.77467679184084));
#136871=CARTESIAN_POINT('Ctrl Pts',(23.7589367722621,1.12132090164701,-6.8518479364826));
#136872=CARTESIAN_POINT('Ctrl Pts',(23.0730067097267,-0.423313420904212,
-6.92901908112437));
#136873=CARTESIAN_POINT('Ctrl Pts',(21.4111777371304,-0.731080198416203,
-7.00619022576612));
#136874=CARTESIAN_POINT('Ctrl Pts',(20.2175881473881,0.465474500993284,
-7.08336137040789));
#136875=CARTESIAN_POINT('Ctrl Pts',(20.5294771087722,2.12653576813143,-7.16053251504964));
#136876=CARTESIAN_POINT('Ctrl Pts',(22.0758100061732,2.80862849930232,-7.23770365969141));
#136877=CARTESIAN_POINT('Ctrl Pts',(23.5128135928929,1.91901288970015,-7.31487480433317));
#136878=CARTESIAN_POINT('Ctrl Pts',(23.5917203626195,0.230763349660865,
-7.39204594897493));
#136879=CARTESIAN_POINT('Ctrl Pts',(22.2439622189305,-0.789003284417116,
-7.46921709361669));
#136880=CARTESIAN_POINT('Ctrl Pts',(20.6407455810999,-0.254135713524417,
-7.54638823825845));
#136881=CARTESIAN_POINT('Ctrl Pts',(20.1752867958861,1.37062985966854,-7.62355938290021));
#136882=CARTESIAN_POINT('Ctrl Pts',(21.2520527599446,2.67322315928684,-7.70073052754197));
#136883=CARTESIAN_POINT('Ctrl Pts',(22.9353671726951,2.521962068814,-7.77790167218374));
#136884=CARTESIAN_POINT('Ctrl Pts',(23.7623346813402,1.04772135592905,-7.85507281682549));
#136885=CARTESIAN_POINT('Ctrl Pts',(23.0144845836534,-0.467206524124539,
-7.93224396146726));
#136886=CARTESIAN_POINT('Ctrl Pts',(21.3413603808458,-0.708723826378064,
-8.00941510610901));
#136887=CARTESIAN_POINT('Ctrl Pts',(20.1976216968665,0.537953632605372,
-8.08658625075078));
#136888=CARTESIAN_POINT('Ctrl Pts',(20.4503846191707,1.63112615715144,-8.13803368051195));
#136889=CARTESIAN_POINT('Ctrl Pts',(20.7769717213703,2.01031192241115,-8.16375739539253));
#136890=CARTESIAN_POINT('Ctrl Pts',(21.575099891413,-0.403869820655514,
-5.94805463602293));
#136891=CARTESIAN_POINT('Ctrl Pts',(21.121160476301,-0.282656475545542,
-5.97378565001271));
#136892=CARTESIAN_POINT('Ctrl Pts',(20.3468011516327,0.43138996963465,-6.02524037888307));
#136893=CARTESIAN_POINT('Ctrl Pts',(20.5743961402856,2.0030975652717,-6.10241882263404));
#136894=CARTESIAN_POINT('Ctrl Pts',(21.9994922341333,2.70064782229422,-6.17958996727579));
#136895=CARTESIAN_POINT('Ctrl Pts',(23.3805539294197,1.92144417477625,-6.25676111191756));
#136896=CARTESIAN_POINT('Ctrl Pts',(23.5189566768722,0.3409521725077,-6.3339322565593));
#136897=CARTESIAN_POINT('Ctrl Pts',(22.2936786727421,-0.666554518081695,
-6.41110340120108));
#136898=CARTESIAN_POINT('Ctrl Pts',(20.7698623018489,-0.225945131216578,
-6.48827454584284));
#136899=CARTESIAN_POINT('Ctrl Pts',(20.2715345905649,1.28008364915676,-6.5654456904846));
#136900=CARTESIAN_POINT('Ctrl Pts',(21.2318341318864,2.54268615936893,-6.64261683512636));
#136901=CARTESIAN_POINT('Ctrl Pts',(22.816210575759,2.46469907232,-6.71978797976812));
#136902=CARTESIAN_POINT('Ctrl Pts',(23.6478509317407,1.11387064999528,-6.79695912440989));
#136903=CARTESIAN_POINT('Ctrl Pts',(23.0040434673074,-0.335908505335176,
-6.87413026905164));
#136904=CARTESIAN_POINT('Ctrl Pts',(21.4442665226809,-0.624775489724847,
-6.9513014136934));
#136905=CARTESIAN_POINT('Ctrl Pts',(20.3239746309601,0.498299425864994,
-7.02847255833517));
#136906=CARTESIAN_POINT('Ctrl Pts',(20.616710658116,2.05735580941485,-7.10564370297692));
#136907=CARTESIAN_POINT('Ctrl Pts',(22.0680840797235,2.69756159094942,-7.18281484761869));
#136908=CARTESIAN_POINT('Ctrl Pts',(23.4168420451171,1.86257679990351,-7.25998599226045));
#136909=CARTESIAN_POINT('Ctrl Pts',(23.4909031923374,0.278001760743005,
-7.33715713690221));
#136910=CARTESIAN_POINT('Ctrl Pts',(22.225910155073,-0.67914155000885,-7.41432828154396));
#136911=CARTESIAN_POINT('Ctrl Pts',(20.7211461930974,-0.177119910439378,
-7.49149942618573));
#136912=CARTESIAN_POINT('Ctrl Pts',(20.2842709828186,1.34786967830866,-7.56867057082749));
#136913=CARTESIAN_POINT('Ctrl Pts',(21.2949133251971,2.57047142040939,-7.64584171546925));
#136914=CARTESIAN_POINT('Ctrl Pts',(22.8748563005945,2.42849919256336,-7.72301286011102));
#136915=CARTESIAN_POINT('Ctrl Pts',(23.6510401770406,1.04479081299699,-7.80018400475277));
#136916=CARTESIAN_POINT('Ctrl Pts',(22.9491151536813,-0.377106156573719,
-7.87735514939454));
#136917=CARTESIAN_POINT('Ctrl Pts',(21.3787366128868,-0.603792010530775,
-7.95452629403629));
#136918=CARTESIAN_POINT('Ctrl Pts',(20.3052343094811,0.566327652788141,
-8.03169743867806));
#136919=CARTESIAN_POINT('Ctrl Pts',(20.5424751959788,1.59236903755359,-8.08314486843923));
#136920=CARTESIAN_POINT('Ctrl Pts',(20.8490067589877,1.94826920786929,-8.10886858331982));
#136921=CARTESIAN_POINT('Ctrl Pts',(21.5996286000554,-0.312018378244399,
-5.89316582395021));
#136922=CARTESIAN_POINT('Ctrl Pts',(21.1753892250981,-0.198735697662014,
-5.91889683793999));
#136923=CARTESIAN_POINT('Ctrl Pts',(20.4516941570929,0.468592601025395,
-5.97035156681035));
#136924=CARTESIAN_POINT('Ctrl Pts',(20.664398215201,1.9374675781506,-6.0475300105613));
#136925=CARTESIAN_POINT('Ctrl Pts',(21.9962540884326,2.58937899009016,-6.12470115520306));
#136926=CARTESIAN_POINT('Ctrl Pts',(23.2869566158643,1.86115655030477,-6.20187229984482));
#136927=CARTESIAN_POINT('Ctrl Pts',(23.4163040422321,0.384071906746946,
-6.27904344448659));
#136928=CARTESIAN_POINT('Ctrl Pts',(22.2711926962766,-0.557516319460856,
-6.35621458912835));
#136929=CARTESIAN_POINT('Ctrl Pts',(20.847075549326,-0.145734824703645,
-6.43338573377011));
#136930=CARTESIAN_POINT('Ctrl Pts',(20.3813520855311,1.26175852613438,-6.51055687841187));
#136931=CARTESIAN_POINT('Ctrl Pts',(21.2788217998135,2.44175233570476,-6.58772802305363));
#136932=CARTESIAN_POINT('Ctrl Pts',(22.7595367363648,2.36886773489025,-6.66489916769539));
#136933=CARTESIAN_POINT('Ctrl Pts',(23.5367650912192,1.10642039834334,-6.74207031233716));
#136934=CARTESIAN_POINT('Ctrl Pts',(22.9350802248881,-0.248503589766242,
-6.81924145697891));
#136935=CARTESIAN_POINT('Ctrl Pts',(21.4773553082314,-0.518470781033478,
-6.89641260162068));
#136936=CARTESIAN_POINT('Ctrl Pts',(20.4303611145322,0.531124350736794,
-6.97358374626243));
#136937=CARTESIAN_POINT('Ctrl Pts',(20.70394420746,1.98817585069818,-7.0507548909042));
#136938=CARTESIAN_POINT('Ctrl Pts',(22.0603581532739,2.5864946825963,-7.12792603554596));
#136939=CARTESIAN_POINT('Ctrl Pts',(23.3208704973414,1.80614071010675,-7.20509718018772));
#136940=CARTESIAN_POINT('Ctrl Pts',(23.3900860220554,0.325240171825252,
-7.28226832482948));
#136941=CARTESIAN_POINT('Ctrl Pts',(22.2078580912154,-0.569279815600576,
-7.35943946947124));
#136942=CARTESIAN_POINT('Ctrl Pts',(20.8015468050948,-0.100104107354348,
-7.43661061411301));
#136943=CARTESIAN_POINT('Ctrl Pts',(20.3932551697511,1.32510949694877,-7.51378175875476));
#136944=CARTESIAN_POINT('Ctrl Pts',(21.3377738904494,2.46771968153194,-7.59095290339653));
#136945=CARTESIAN_POINT('Ctrl Pts',(22.8143454284941,2.33503631631273,-7.66812404803829));
#136946=CARTESIAN_POINT('Ctrl Pts',(23.5397456727409,1.04186027006484,-7.74529519268004));
#136947=CARTESIAN_POINT('Ctrl Pts',(22.8837457237093,-0.287005789023116,
-7.82246633732181));
#136948=CARTESIAN_POINT('Ctrl Pts',(21.4161128449277,-0.498860194683393,
-7.89963748196357));
#136949=CARTESIAN_POINT('Ctrl Pts',(20.4128469220958,0.594701672970821,
-7.97680862660533));
#136950=CARTESIAN_POINT('Ctrl Pts',(20.6345657727871,1.55361191795564,-8.0282560563665));
#136951=CARTESIAN_POINT('Ctrl Pts',(20.9210417966052,1.88622649332765,-8.05397977124709));
#136952=CARTESIAN_POINT('Ctrl Pts',(21.6241573086981,-0.220166935833395,
-5.83827701187748));
#136953=CARTESIAN_POINT('Ctrl Pts',(21.2296179738952,-0.11481491977837,
-5.86400802586726));
#136954=CARTESIAN_POINT('Ctrl Pts',(20.556587162553,0.505795232416153,-5.91546275473762));
#136955=CARTESIAN_POINT('Ctrl Pts',(20.7544002901164,1.87183759102959,-5.99264119848858));
#136956=CARTESIAN_POINT('Ctrl Pts',(21.9930159427319,2.47811015788609,-6.06981234313035));
#136957=CARTESIAN_POINT('Ctrl Pts',(23.1933593023089,1.80086892583339,-6.1469834877721));
#136958=CARTESIAN_POINT('Ctrl Pts',(23.3136514075921,0.427191640986089,
-6.22415463241387));
#136959=CARTESIAN_POINT('Ctrl Pts',(22.2487067198108,-0.44847812084011,
-6.30132577705563));
#136960=CARTESIAN_POINT('Ctrl Pts',(20.9242887968032,-0.0655245181906094,
-6.37849692169738));
#136961=CARTESIAN_POINT('Ctrl Pts',(20.4911695804971,1.24343340311209,-6.45566806633915));
#136962=CARTESIAN_POINT('Ctrl Pts',(21.3258094677405,2.34081851204049,-6.5328392109809));
#136963=CARTESIAN_POINT('Ctrl Pts',(22.7028628969708,2.27303639746039,-6.61001035562267));
#136964=CARTESIAN_POINT('Ctrl Pts',(23.4256792506978,1.09897014669149,-6.68718150026444));
#136965=CARTESIAN_POINT('Ctrl Pts',(22.8661169824689,-0.161098674197309,
-6.76435264490619));
#136966=CARTESIAN_POINT('Ctrl Pts',(21.5104440937819,-0.412166072342206,
-6.84152378954795));
#136967=CARTESIAN_POINT('Ctrl Pts',(20.5367475981041,0.563949275608491,
-6.91869493418971));
#136968=CARTESIAN_POINT('Ctrl Pts',(20.7911777568038,1.91899589198159,-6.99586607883148));
#136969=CARTESIAN_POINT('Ctrl Pts',(22.0526322268242,2.47542777424339,-7.07303722347324));
#136970=CARTESIAN_POINT('Ctrl Pts',(23.2248989495656,1.74970462031009,-7.150208368115));
#136971=CARTESIAN_POINT('Ctrl Pts',(23.2892688517734,0.372478582907392,
-7.22737951275675));
#136972=CARTESIAN_POINT('Ctrl Pts',(22.1898060273579,-0.459418081192311,
-7.30455065739853));
#136973=CARTESIAN_POINT('Ctrl Pts',(20.8819474170923,-0.023088304269212,
-7.38172180204028));
#136974=CARTESIAN_POINT('Ctrl Pts',(20.5022393566836,1.30234931558909,-7.45889294668204));
#136975=CARTESIAN_POINT('Ctrl Pts',(21.3806344557018,2.36496794265449,-7.53606409132381));
#136976=CARTESIAN_POINT('Ctrl Pts',(22.7538345563936,2.24157344006209,-7.61323523596556));
#136977=CARTESIAN_POINT('Ctrl Pts',(23.4284511684412,1.03892972713279,-7.69040638060732));
#136978=CARTESIAN_POINT('Ctrl Pts',(22.8183762937372,-0.196905421472411,
-7.76757752524909));
#136979=CARTESIAN_POINT('Ctrl Pts',(21.4534890769687,-0.39392837883621,
-7.84474866989084));
#136980=CARTESIAN_POINT('Ctrl Pts',(20.5204595347103,0.623075693153492,
-7.92191981453261));
#136981=CARTESIAN_POINT('Ctrl Pts',(20.7266563495953,1.51485479835789,-7.97336724429378));
#136982=CARTESIAN_POINT('Ctrl Pts',(20.9930768342227,1.82418377878579,-7.99909095917437));
#136983=CARTESIAN_POINT('Ctrl Pts',(20.9918838262563,1.82521129893647,-8.));
#136984=CARTESIAN_POINT('Ctrl Pts',(20.9541736290457,1.7899949864246,-7.99999999999999));
#136985=CARTESIAN_POINT('Ctrl Pts',(20.9189421813825,1.75244101387378,-8.00000000000001));
#136986=CARTESIAN_POINT('Ctrl Pts',(20.8861950848217,1.71289003134968,-8.));
#136987=CARTESIAN_POINT('Ctrl Pts',(20.853447988261,1.67333904882559,-7.99999999999999));
#136988=CARTESIAN_POINT('Ctrl Pts',(20.8231848331265,1.6317902796713,-7.99999999999998));
#136989=CARTESIAN_POINT('Ctrl Pts',(20.7954373659385,1.58853793355712,-8.00000000000001));
#136990=CARTESIAN_POINT('Ctrl Pts',(20.7732297117916,1.55392096700529,-8.00000000000003));
#136991=CARTESIAN_POINT('Ctrl Pts',(20.7526339197316,1.51821170948909,-8.));
#136992=CARTESIAN_POINT('Ctrl Pts',(20.7336810273727,1.48154467475702,-8.00000000000002));
#136993=CARTESIAN_POINT('Ctrl Pts',(20.726536783042,1.46772312973639,-8.00000000000003));
#136994=CARTESIAN_POINT('Ctrl Pts',(20.7196261229699,1.45376537070319,-7.99999999999999));
#136995=CARTESIAN_POINT('Ctrl Pts',(20.7129512623861,1.43967819719058,-7.99999999999998));
#136996=CARTESIAN_POINT('Ctrl Pts',(20.7070330573699,1.42718793167859,-7.99999999999997));
#136997=CARTESIAN_POINT('Ctrl Pts',(20.7012981529128,1.41459078408099,-8.00000000000003));
#136998=CARTESIAN_POINT('Ctrl Pts',(20.6957608414974,1.40192125070293,-8.00000000000002));
#136999=CARTESIAN_POINT('Ctrl Pts',(20.6737369579797,1.35152994950819,-7.99999999999999));
#137000=CARTESIAN_POINT('Ctrl Pts',(20.6547986385331,1.2999239934859,-8.00000000000001));
#137001=CARTESIAN_POINT('Ctrl Pts',(20.6389780553483,1.24744385996292,-8.00000000000001));
#137002=CARTESIAN_POINT('Ctrl Pts',(20.6231888957401,1.19506796491689,-8.00000000000001));
#137003=CARTESIAN_POINT('Ctrl Pts',(20.6105046386363,1.14182034428139,-8.00000000000002));
#137004=CARTESIAN_POINT('Ctrl Pts',(20.6009968185427,1.0880060551986,-7.99999999999999));
#137005=CARTESIAN_POINT('Ctrl Pts',(20.5944878672644,1.05116537223739,-7.99999999999998));
#137006=CARTESIAN_POINT('Ctrl Pts',(20.5894684106341,1.01405841881779,-8.00000000000001));
#137007=CARTESIAN_POINT('Ctrl Pts',(20.5859738441328,0.976777779161468,
-8.00000000000002));
#137008=CARTESIAN_POINT('Ctrl Pts',(20.5845818516926,0.961927763130589,
-8.00000000000002));
#137009=CARTESIAN_POINT('Ctrl Pts',(20.5834319296435,0.947050157339097,
-7.99999999999998));
#137010=CARTESIAN_POINT('Ctrl Pts',(20.5825268097375,0.932150722589904,
-7.99999999999999));
#137011=CARTESIAN_POINT('Ctrl Pts',(20.5818019843319,0.920219166600302,
-8.));
#137012=CARTESIAN_POINT('Ctrl Pts',(20.5812342253425,0.90827150701319,-7.99999999999999));
#137013=CARTESIAN_POINT('Ctrl Pts',(20.5808254143592,0.896333256574007,
-7.99999999999999));
#137014=CARTESIAN_POINT('Ctrl Pts',(20.5788808866177,0.839548433971287,
-8.00000000000002));
#137015=CARTESIAN_POINT('Ctrl Pts',(20.5805206286002,0.782868663148789,
-8.00000000000002));
#137016=CARTESIAN_POINT('Ctrl Pts',(20.5858066279648,0.726625687387986,
-8.00000000000003));
#137017=CARTESIAN_POINT('Ctrl Pts',(20.5884732528979,0.698252827095684,
-8.00000000000003));
#137018=CARTESIAN_POINT('Ctrl Pts',(20.5920685373646,0.66999072900109,-8.00000000000001));
#137019=CARTESIAN_POINT('Ctrl Pts',(20.5966051943139,0.64188030405106,-8.));
#137020=CARTESIAN_POINT('Ctrl Pts',(20.6053459061087,0.587720351984889,
-7.99999999999999));
#137021=CARTESIAN_POINT('Ctrl Pts',(20.6175777428586,0.534123155199587,
-8.00000000000002));
#137022=CARTESIAN_POINT('Ctrl Pts',(20.6330759201249,0.481297569340178,
-8.00000000000001));
#137023=CARTESIAN_POINT('Ctrl Pts',(20.6416495038376,0.45207448234359,-8.00000000000001));
#137024=CARTESIAN_POINT('Ctrl Pts',(20.6512236307377,0.423087531025189,
-7.99999999999999));
#137025=CARTESIAN_POINT('Ctrl Pts',(20.6617668071571,0.394372949822668,
-8.00000000000001));
#137026=CARTESIAN_POINT('Ctrl Pts',(20.6648815792871,0.385889796957085,
-8.00000000000001));
#137027=CARTESIAN_POINT('Ctrl Pts',(20.6680802804164,0.37743243703309,-8.00000000000001));
#137028=CARTESIAN_POINT('Ctrl Pts',(20.6713586286263,0.369010110250361,
-8.00000000000001));
#137029=CARTESIAN_POINT('Ctrl Pts',(20.6921831588778,0.315510302528568,
-7.99999999999998));
#137030=CARTESIAN_POINT('Ctrl Pts',(20.7162516631977,0.263328227715186,
-8.00000000000001));
#137031=CARTESIAN_POINT('Ctrl Pts',(20.7432800553111,0.212688089663163,
-8.00000000000001));
#137032=CARTESIAN_POINT('Ctrl Pts',(20.7703084474246,0.16204795161114,-8.));
#137033=CARTESIAN_POINT('Ctrl Pts',(20.8002972504436,0.112948872810922,
-8.00000000000002));
#137034=CARTESIAN_POINT('Ctrl Pts',(20.8330152064058,0.0656202583694562,
-7.99999999999999));
#137035=CARTESIAN_POINT('Ctrl Pts',(20.8550444161516,0.033753598492684,
-7.99999999999997));
#137036=CARTESIAN_POINT('Ctrl Pts',(20.8783119487322,0.00268967994438171,
-7.99999999999998));
#137037=CARTESIAN_POINT('Ctrl Pts',(20.9027588922466,-0.0274970785187473,
-7.99999999999999));
#137038=CARTESIAN_POINT('Ctrl Pts',(20.9161338996896,-0.0440123585939095,
-7.99999999999999));
#137039=CARTESIAN_POINT('Ctrl Pts',(20.9298620860546,-0.0602650077312124,
-8.));
#137040=CARTESIAN_POINT('Ctrl Pts',(20.943934853256,-0.076242148539782,
-8.00000000000001));
#137041=CARTESIAN_POINT('Ctrl Pts',(20.9530636468032,-0.0866062807555108,
-8.00000000000002));
#137042=CARTESIAN_POINT('Ctrl Pts',(20.9623392154689,-0.0968561564262098,
-7.99999999999999));
#137043=CARTESIAN_POINT('Ctrl Pts',(20.9717431595962,-0.106971327962954,
-7.99999999999999));
#137044=CARTESIAN_POINT('Ctrl Pts',(21.0128363428694,-0.151172419778212,
-8.00000000000002));
#137045=CARTESIAN_POINT('Ctrl Pts',(21.0564377857545,-0.192874140272209,
-7.99999999999998));
#137046=CARTESIAN_POINT('Ctrl Pts',(21.1023016075224,-0.231816511631777,
-7.99999999999999));
#137047=CARTESIAN_POINT('Ctrl Pts',(21.1275553642185,-0.253259146230811,
-7.99999999999999));
#137048=CARTESIAN_POINT('Ctrl Pts',(21.1534959113046,-0.27386483331401,
-8.00000000000003));
#137049=CARTESIAN_POINT('Ctrl Pts',(21.1800878941763,-0.293586552696765,
-7.99999999999999));
#137050=CARTESIAN_POINT('Ctrl Pts',(21.1924609737589,-0.302762942611214,
-7.99999999999997));
#137051=CARTESIAN_POINT('Ctrl Pts',(21.2049751404292,-0.311747911286012,
-8.00000000000002));
#137052=CARTESIAN_POINT('Ctrl Pts',(21.2176270920186,-0.320536469337559,
-8.));
#137053=CARTESIAN_POINT('Ctrl Pts',(21.2273289146901,-0.327275748345412,
-7.99999999999999));
#137054=CARTESIAN_POINT('Ctrl Pts',(21.2371108801724,-0.333898821072215,
-8.00000000000001));
#137055=CARTESIAN_POINT('Ctrl Pts',(21.2469630076195,-0.340398109798504,
-8.));
#137056=CARTESIAN_POINT('Ctrl Pts',(21.2977187506139,-0.373880850456119,
-7.99999999999999));
#137057=CARTESIAN_POINT('Ctrl Pts',(21.3503919284324,-0.404122029455814,
-7.99999999999999));
#137058=CARTESIAN_POINT('Ctrl Pts',(21.4047547874969,-0.430847423133963,
-7.99999999999997));
#137059=CARTESIAN_POINT('Ctrl Pts',(21.4148034792473,-0.435787473153416,
-7.99999999999997));
#137060=CARTESIAN_POINT('Ctrl Pts',(21.4249100090732,-0.440607300547516,
-7.99999999999999));
#137061=CARTESIAN_POINT('Ctrl Pts',(21.4350730759621,-0.445305031926257,
-7.99999999999999));
#137062=CARTESIAN_POINT('Ctrl Pts',(21.4726734393702,-0.462685258679122,
-7.99999999999997));
#137063=CARTESIAN_POINT('Ctrl Pts',(21.5110471671993,-0.478395112197247,
-7.99999999999998));
#137064=CARTESIAN_POINT('Ctrl Pts',(21.5500882629145,-0.492459351166239,
-7.99999999999999));
#137065=CARTESIAN_POINT('',(20.9909269206557,1.82544017965477,-5.99954793025018));
#137066=CARTESIAN_POINT('Ctrl Pts',(20.9992015084306,1.83363212414324,-6.00000000000001));
#137067=CARTESIAN_POINT('Ctrl Pts',(20.9966508632533,1.83072298777096,-5.9998493100834));
#137068=CARTESIAN_POINT('Ctrl Pts',(20.9941135696973,1.8278021450906,-5.99969862016679));
#137069=CARTESIAN_POINT('Ctrl Pts',(20.9915897346506,1.82486971914787,-5.99954793025018));
#137070=CARTESIAN_POINT('Ctrl Pts',(21.5514861371214,-0.490649428218508,
-5.99999999999999));
#137071=CARTESIAN_POINT('Ctrl Pts',(21.4949834591969,-0.470003582263612,
-6.00000000000002));
#137072=CARTESIAN_POINT('Ctrl Pts',(21.4399877915486,-0.445869143432613,
-6.));
#137073=CARTESIAN_POINT('Ctrl Pts',(21.3866896987483,-0.418529366433886,
-5.99999999999999));
#137074=CARTESIAN_POINT('Ctrl Pts',(21.3328432740675,-0.390908317244221,
-5.99999999999998));
#137075=CARTESIAN_POINT('Ctrl Pts',(21.2807287721543,-0.36001475981561,
-5.99999999999998));
#137076=CARTESIAN_POINT('Ctrl Pts',(21.2305741784146,-0.326096358997265,
-6.));
#137077=CARTESIAN_POINT('Ctrl Pts',(21.1934054239874,-0.300959983311997,
-6.00000000000002));
#137078=CARTESIAN_POINT('Ctrl Pts',(21.1573136603092,-0.27416135946932,
-5.99999999999998));
#137079=CARTESIAN_POINT('Ctrl Pts',(21.1224063705073,-0.245790103209091,
-6.));
#137080=CARTESIAN_POINT('Ctrl Pts',(21.105219694232,-0.231821456555714,
-6.00000000000001));
#137081=CARTESIAN_POINT('Ctrl Pts',(21.0883203569688,-0.217471465991212,
-6.00000000000003));
#137082=CARTESIAN_POINT('Ctrl Pts',(21.0717225016579,-0.202750241854179,
-6.));
#137083=CARTESIAN_POINT('Ctrl Pts',(21.0641043039211,-0.195993393194915,
-5.99999999999999));
#137084=CARTESIAN_POINT('Ctrl Pts',(21.0565478764263,-0.189156706417304,
-6.00000000000002));
#137085=CARTESIAN_POINT('Ctrl Pts',(21.0490604314974,-0.182246490416036,
-6.00000000000002));
#137086=CARTESIAN_POINT('Ctrl Pts',(21.0055579107356,-0.142097705627706,
-6.00000000000003));
#137087=CARTESIAN_POINT('Ctrl Pts',(20.9644984406401,-0.09958055327981,
-6.00000000000001));
#137088=CARTESIAN_POINT('Ctrl Pts',(20.9260875776447,-0.0549349400849231,
-6.));
#137089=CARTESIAN_POINT('Ctrl Pts',(20.8883573993092,-0.0110804984926149,
-5.99999999999999));
#137090=CARTESIAN_POINT('Ctrl Pts',(20.8531823109083,0.0348285706127793,
-6.00000000000002));
#137091=CARTESIAN_POINT('Ctrl Pts',(20.8207996842225,0.0825894135497585,
-6.00000000000004));
#137092=CARTESIAN_POINT('Ctrl Pts',(20.7977058825238,0.116650252605579,
-6.00000000000005));
#137093=CARTESIAN_POINT('Ctrl Pts',(20.7760331558444,0.151653411765795,
-6.00000000000002));
#137094=CARTESIAN_POINT('Ctrl Pts',(20.7558832023643,0.187529331316934,
-6.00000000000003));
#137095=CARTESIAN_POINT('Ctrl Pts',(20.7431189344056,0.210255430951394,
-6.00000000000004));
#137096=CARTESIAN_POINT('Ctrl Pts',(20.7309659887369,0.233331802916497,
-6.00000000000001));
#137097=CARTESIAN_POINT('Ctrl Pts',(20.719453249643,0.256740991241418,-6.));
#137098=CARTESIAN_POINT('Ctrl Pts',(20.7148859970124,0.266027719281294,
-6.));
#137099=CARTESIAN_POINT('Ctrl Pts',(20.7104195531109,0.275367023870494,
-6.));
#137100=CARTESIAN_POINT('Ctrl Pts',(20.7060617989844,0.284744216998827,
-6.));
#137101=CARTESIAN_POINT('Ctrl Pts',(20.6825201841584,0.335402024293288,
-6.00000000000001));
#137102=CARTESIAN_POINT('Ctrl Pts',(20.662098249384,0.387261045497689,-6.00000000000001));
#137103=CARTESIAN_POINT('Ctrl Pts',(20.6450102486691,0.440132204936083,
-6.00000000000001));
#137104=CARTESIAN_POINT('Ctrl Pts',(20.6354739824902,0.469637906510392,
-6.));
#137105=CARTESIAN_POINT('Ctrl Pts',(20.6269768889554,0.499459101243191,
-5.99999999999999));
#137106=CARTESIAN_POINT('Ctrl Pts',(20.6195632260797,0.529564129721978,
-6.));
#137107=CARTESIAN_POINT('Ctrl Pts',(20.6059643035353,0.584785948861191,
-6.00000000000002));
#137108=CARTESIAN_POINT('Ctrl Pts',(20.5960079764508,0.640963673571786,
-6.00000000000001));
#137109=CARTESIAN_POINT('Ctrl Pts',(20.5896384223682,0.697753556830416,
-6.00000000000001));
#137110=CARTESIAN_POINT('Ctrl Pts',(20.587064820506,0.720699362363084,-6.00000000000001));
#137111=CARTESIAN_POINT('Ctrl Pts',(20.5850773566103,0.743744977060889,
-6.00000000000001));
#137112=CARTESIAN_POINT('Ctrl Pts',(20.5836746271151,0.766866927816636,
-5.99999999999999));
#137113=CARTESIAN_POINT('Ctrl Pts',(20.5827714922943,0.781753788699393,
-5.99999999999998));
#137114=CARTESIAN_POINT('Ctrl Pts',(20.5821107673882,0.796678748464092,
-6.));
#137115=CARTESIAN_POINT('Ctrl Pts',(20.5816928183164,0.811599876685016,
-6.));
#137116=CARTESIAN_POINT('Ctrl Pts',(20.5801300585453,0.867391695582489,
-6.));
#137117=CARTESIAN_POINT('Ctrl Pts',(20.581949848881,0.923205339792386,-5.99999999999998));
#137118=CARTESIAN_POINT('Ctrl Pts',(20.5870584639554,0.978720641379529,
-5.99999999999999));
#137119=CARTESIAN_POINT('Ctrl Pts',(20.5921383214789,1.03392343476379,-6.00000000000001));
#137120=CARTESIAN_POINT('Ctrl Pts',(20.60047054055,1.08883235822639,-6.));
#137121=CARTESIAN_POINT('Ctrl Pts',(20.6120117156267,1.1431172831597,-6.));
#137122=CARTESIAN_POINT('Ctrl Pts',(20.6238588849131,1.19884147858242,-6.));
#137123=CARTESIAN_POINT('Ctrl Pts',(20.6390876536583,1.25390950243899,-5.99999999999996));
#137124=CARTESIAN_POINT('Ctrl Pts',(20.6576977119408,1.3079290601828,-6.00000000000001));
#137125=CARTESIAN_POINT('Ctrl Pts',(20.6613927260947,1.31865460587539,-6.00000000000002));
#137126=CARTESIAN_POINT('Ctrl Pts',(20.6652180608678,1.3293295832012,-5.99999999999997));
#137127=CARTESIAN_POINT('Ctrl Pts',(20.6691724961882,1.33994907575922,-5.99999999999997));
#137128=CARTESIAN_POINT('Ctrl Pts',(20.6878284671583,1.39004900882909,-5.99999999999996));
#137129=CARTESIAN_POINT('Ctrl Pts',(20.7093599470678,1.43893173492499,-5.99999999999996));
#137130=CARTESIAN_POINT('Ctrl Pts',(20.7337384463524,1.48628230063181,-5.99999999999997));
#137131=CARTESIAN_POINT('Ctrl Pts',(20.7471332785947,1.51229919678329,-5.99999999999997));
#137132=CARTESIAN_POINT('Ctrl Pts',(20.761388315785,1.53785300092719,-5.99999999999999));
#137133=CARTESIAN_POINT('Ctrl Pts',(20.7765035286841,1.56288657427844,-5.99999999999997));
#137134=CARTESIAN_POINT('Ctrl Pts',(20.7831423587351,1.57388169820809,-5.99999999999996));
#137135=CARTESIAN_POINT('Ctrl Pts',(20.7899483342675,1.58477821309829,-5.99999999999998));
#137136=CARTESIAN_POINT('Ctrl Pts',(20.7969178962072,1.59556525345604,-5.99999999999998));
#137137=CARTESIAN_POINT('Ctrl Pts',(20.824855624804,1.63880547550779,-5.99999999999998));
#137138=CARTESIAN_POINT('Ctrl Pts',(20.8553594001569,1.68019899715349,-5.99999999999999));
#137139=CARTESIAN_POINT('Ctrl Pts',(20.8884135643584,1.71944475979049,-6.));
#137140=CARTESIAN_POINT('Ctrl Pts',(20.8979162936708,1.730727509423,-6.));
#137141=CARTESIAN_POINT('Ctrl Pts',(20.9076300218124,1.74183249577189,-6.00000000000001));
#137142=CARTESIAN_POINT('Ctrl Pts',(20.9175548621962,1.75275191469634,-6.));
#137143=CARTESIAN_POINT('Ctrl Pts',(20.9406639670501,1.7781768068971,-5.99999999999998));
#137144=CARTESIAN_POINT('Ctrl Pts',(20.964917450545,1.8025962199065,-6.));
#137145=CARTESIAN_POINT('Ctrl Pts',(20.9902312754079,1.8259702455601,-6.));
#137146=CARTESIAN_POINT('Origin',(-2.15847961726464E-8,0.999999999999992,
-8.00000000000001));
#137147=CARTESIAN_POINT('',(17.5765008039206,6.73438257216289,-8.00000000000001));
#137148=CARTESIAN_POINT('',(17.2475487250834,6.96527972946289,-8.00000000000001));
#137149=CARTESIAN_POINT('Origin',(18.0333567325795,7.735023696867,-8.00000000000001));
#137150=CARTESIAN_POINT('',(23.3621001218732,4.09289074857519,-8.00000000000001));
#137151=CARTESIAN_POINT('',(11.1961524660154,9.64741492024149,-8.00000000000001));
#137152=CARTESIAN_POINT('',(23.3621001218732,-2.09289074857521,-8.00000000000001));
#137153=CARTESIAN_POINT('Origin',(21.9499999789786,0.999999999999992,-8.00000000000001));
#137154=CARTESIAN_POINT('',(17.5765008039206,-4.73438257216291,-8.00000000000001));
#137155=CARTESIAN_POINT('',(14.2802181394665,-6.23934398201561,-8.00000000000001));
#137156=CARTESIAN_POINT('',(17.2475487250834,-4.96527972946291,-8.00000000000001));
#137157=CARTESIAN_POINT('Origin',(18.0333567325795,-5.73502369686701,-8.00000000000001));
#137158=CARTESIAN_POINT('',(18.2499999789787,0.99999999999999,-8.00000000000001));
#137159=CARTESIAN_POINT('Origin',(-2.10213452200837E-8,0.999999999999992,
-8.00000000000001));
#137160=CARTESIAN_POINT('Origin',(-2.10213452200837E-8,0.999999999999992,
-8.00000000000001));
#137161=CARTESIAN_POINT('Origin',(-2.10213452200837E-8,0.999999999999992,
-4.55000000000001));
#137162=CARTESIAN_POINT('',(7.99999997897866,0.999999999999992,-4.6));
#137163=CARTESIAN_POINT('Origin',(-2.10213452200837E-8,0.999999999999992,
-4.6));
#137164=CARTESIAN_POINT('',(7.89999997897866,0.999999999999992,-4.50000000000001));
#137165=CARTESIAN_POINT('',(7.94999997897866,0.999999999999991,-4.55000000000001));
#137166=CARTESIAN_POINT('Origin',(-2.10213452200837E-8,0.999999999999992,
-4.50000000000001));
#137167=CARTESIAN_POINT('Origin',(-2.10213452200837E-8,0.999999999999992,
-6.00000000000001));
#137168=CARTESIAN_POINT('',(7.99999997897866,0.999999999999992,-6.00000000000001));
#137169=CARTESIAN_POINT('',(7.99999997897866,0.999999999999993,-6.00000000000001));
#137170=CARTESIAN_POINT('Origin',(-2.10213452200837E-8,0.999999999999992,
-6.00000000000001));
#137171=CARTESIAN_POINT('Origin',(-2.10213446649728E-8,0.999999999999992,
-4.50000000000001));
#137172=CARTESIAN_POINT('',(-1.50000000000001,1.00000037997959,-4.50000000000001));
#137173=CARTESIAN_POINT('Origin',(-8.88178376686733E-15,1.00000037997959,
-4.50000000000001));
#137174=CARTESIAN_POINT('Origin',(-2.10213452200837E-8,0.999999999999992,
-9.95000000000001));
#137175=CARTESIAN_POINT('',(18.2499999789787,0.999999999999992,-9.90000000000001));
#137176=CARTESIAN_POINT('',(-18.2500000210213,0.99999999999999,-9.9));
#137177=CARTESIAN_POINT('Origin',(-2.10213452200837E-8,0.999999999999992,
-9.90000000000001));
#137178=CARTESIAN_POINT('',(-18.1500000210213,0.999999999999992,-10.));
#137179=CARTESIAN_POINT('',(-18.2000000210213,0.99999999999999,-9.95000000000001));
#137180=CARTESIAN_POINT('Origin',(-2.10213452200837E-8,0.999999999999992,
-10.));
#137181=CARTESIAN_POINT('Origin',(-2.10213452200837E-8,0.999999999999992,
-9.90000000000001));
#137182=CARTESIAN_POINT('Origin',(-2.10213452200837E-8,0.999999999999992,
-6.00000000000001));
#137183=CARTESIAN_POINT('',(18.2499999789787,0.99999999999999,-6.00000000000001));
#137184=CARTESIAN_POINT('',(17.0965589791457,-5.38515233599081,-7.90000000000001));
#137185=CARTESIAN_POINT('Ctrl Pts',(17.0965589791457,-5.38515233599079,
-7.90000000000003));
#137186=CARTESIAN_POINT('Ctrl Pts',(17.1569700573172,-5.22339870696598,
-7.90000000000003));
#137187=CARTESIAN_POINT('Ctrl Pts',(17.2046206918192,-5.08939852688342,
-7.94381226975377));
#137188=CARTESIAN_POINT('Ctrl Pts',(17.2475487250834,-4.96527972946291,
-8.));
#137189=CARTESIAN_POINT('',(17.0965589791457,-5.38515233599081,-6.1));
#137190=CARTESIAN_POINT('',(17.0965589791457,-5.38515233599081,-6.00000000000001));
#137191=CARTESIAN_POINT('',(-17.0965590211555,-5.38515233607861,-6.1));
#137192=CARTESIAN_POINT('Origin',(-2.10213452200837E-8,0.999999999999992,
-6.1));
#137193=CARTESIAN_POINT('',(-17.0965590211555,-5.38515233607861,-7.90000000000001));
#137194=CARTESIAN_POINT('',(-17.0965590211555,-5.38515233607861,-6.00000000000001));
#137195=CARTESIAN_POINT('Ctrl Pts',(-17.2475487670954,-4.96527972955151,
-7.99999999999999));
#137196=CARTESIAN_POINT('Ctrl Pts',(-17.2046207338306,-5.0893985269718,
-7.94381226975377));
#137197=CARTESIAN_POINT('Ctrl Pts',(-17.1569700993279,-5.2233987070541,
-7.90000000000004));
#137198=CARTESIAN_POINT('Ctrl Pts',(-17.0965590211556,-5.38515233607859,
-7.90000000000004));
#137199=CARTESIAN_POINT('',(-17.0965590211555,7.38515233607859,-7.90000000000001));
#137200=CARTESIAN_POINT('Ctrl Pts',(-17.0965590211555,7.38515233607864,
-7.90000000000007));
#137201=CARTESIAN_POINT('Ctrl Pts',(-17.1569700993279,7.22339870705413,
-7.90000000000008));
#137202=CARTESIAN_POINT('Ctrl Pts',(-17.2046207338306,7.08939852697181,
-7.94381226975381));
#137203=CARTESIAN_POINT('Ctrl Pts',(-17.2475487670954,6.96527972955152,
-8.00000000000005));
#137204=CARTESIAN_POINT('',(-17.0965590211555,7.38515233607859,-6.1));
#137205=CARTESIAN_POINT('',(-17.0965590211555,7.38515233607859,-6.00000000000001));
#137206=CARTESIAN_POINT('',(17.0965589791457,7.38515233599079,-6.1));
#137207=CARTESIAN_POINT('Origin',(-2.10213452200837E-8,0.999999999999992,
-6.1));
#137208=CARTESIAN_POINT('',(17.0965589791457,7.38515233599079,-7.90000000000001));
#137209=CARTESIAN_POINT('',(17.0965589791457,7.38515233599079,-6.00000000000001));
#137210=CARTESIAN_POINT('Ctrl Pts',(17.2475487250834,6.96527972946289,-8.00000000000001));
#137211=CARTESIAN_POINT('Ctrl Pts',(17.2046206918192,7.08939852688341,-7.94381226975377));
#137212=CARTESIAN_POINT('Ctrl Pts',(17.1569700573172,7.22339870696597,-7.90000000000002));
#137213=CARTESIAN_POINT('Ctrl Pts',(17.0965589791457,7.3851523359908,-7.90000000000003));
#137214=CARTESIAN_POINT('Origin',(-8.88178376686733E-15,1.00000037997959,
-10.));
#137215=CARTESIAN_POINT('',(-17.5,1.00000037997959,-10.));
#137216=CARTESIAN_POINT('Origin',(-8.88178376686733E-15,1.00000037997959,
-10.));
#137217=CARTESIAN_POINT('Origin',(-2.10213452200837E-8,0.999999999999992,
-19.05));
#137218=CARTESIAN_POINT('',(18.2499999789787,0.999999999999992,-19.1));
#137219=CARTESIAN_POINT('',(-18.2500000210213,0.999999999999994,-19.1));
#137220=CARTESIAN_POINT('Origin',(-2.10213452200837E-8,0.999999999999992,
-19.1));
#137221=CARTESIAN_POINT('',(-18.1500000210213,0.999999999999992,-19.));
#137222=CARTESIAN_POINT('',(-18.2000000210213,0.999999999999994,-19.05));
#137223=CARTESIAN_POINT('Origin',(-2.10213452200837E-8,0.999999999999992,
-19.));
#137224=CARTESIAN_POINT('Origin',(-2.10213452200837E-8,0.999999999999992,
-19.1));
#137225=CARTESIAN_POINT('Origin',(-2.10213452200837E-8,0.999999999999992,
-6.00000000000001));
#137226=CARTESIAN_POINT('',(18.2499999789787,0.999999999999992,-23.4));
#137227=CARTESIAN_POINT('Origin',(-2.10213452200837E-8,0.999999999999992,
-23.4));
#137228=CARTESIAN_POINT('',(18.2499999789787,0.99999999999999,-6.00000000000001));
#137229=CARTESIAN_POINT('Origin',(-8.88178376686733E-15,1.00000037997959,
-19.));
#137230=CARTESIAN_POINT('',(-17.5,1.00000037997959,-19.));
#137231=CARTESIAN_POINT('Origin',(-8.88178376686733E-15,1.00000037997959,
-19.));
#137232=CARTESIAN_POINT('Origin',(-2.10213452200837E-8,0.999999999999992,
-23.45));
#137233=CARTESIAN_POINT('',(-2.50000002102135,0.999999999999992,-23.4));
#137234=CARTESIAN_POINT('Origin',(-2.10213452200837E-8,0.999999999999992,
-23.4));
#137235=CARTESIAN_POINT('',(-2.60000002102135,0.999999999999992,-23.5));
#137236=CARTESIAN_POINT('',(-2.55000002102135,0.999999999999992,-23.45));
#137237=CARTESIAN_POINT('Origin',(-2.10213452200837E-8,0.999999999999992,
-23.5));
#137238=CARTESIAN_POINT('Origin',(-2.10213446649728E-8,0.999999999999992,
-23.5));
#137239=CARTESIAN_POINT('',(18.1499999789787,0.999999999999992,-23.5));
#137240=CARTESIAN_POINT('Origin',(-2.10213452200837E-8,0.999999999999992,
-23.5));
#137241=CARTESIAN_POINT('Origin',(-2.10213452200837E-8,0.999999999999992,
-6.00000000000001));
#137242=CARTESIAN_POINT('',(-2.50000002102135,0.999999999999992,-23.));
#137243=CARTESIAN_POINT('',(-2.50000002102135,0.999999999999992,-6.00000000000001));
#137244=CARTESIAN_POINT('Origin',(-2.10213452200837E-8,0.999999999999992,
-23.));
#137245=CARTESIAN_POINT('Origin',(-2.10213452200837E-8,0.999999999999992,
-23.45));
#137246=CARTESIAN_POINT('',(18.1999999789787,0.999999999999994,-23.45));
#137247=CARTESIAN_POINT('Origin',(-18.0333567745876,7.73502369695969,-7.95000000000001));
#137248=CARTESIAN_POINT('',(-17.6180332032306,6.82534994715959,-7.90000000000001));
#137249=CARTESIAN_POINT('',(-17.5765008460949,6.73438257217959,-8.00000000000001));
#137250=CARTESIAN_POINT('Origin',(-18.0333567745876,7.73502369695969,-7.90000000000001));
#137251=CARTESIAN_POINT('Origin',(-23.1316149713403,4.25308657096129,-7.95000000000001));
#137252=CARTESIAN_POINT('',(-23.4036325210056,4.18385812481499,-7.90000000000001));
#137253=CARTESIAN_POINT('',(-23.3621001638699,4.09289074983499,-8.00000000000001));
#137254=CARTESIAN_POINT('',(-23.1523811499082,4.29857025845129,-7.90000000000001));
#137255=CARTESIAN_POINT('Origin',(-21.9500000210213,0.999999999999992,-7.95000000000001));
#137256=CARTESIAN_POINT('',(-23.4036325210056,-2.18385812481501,-7.90000000000001));
#137257=CARTESIAN_POINT('',(-23.3621001638699,-2.09289074983501,-8.00000000000001));
#137258=CARTESIAN_POINT('Origin',(-21.9500000210213,0.999999999999992,-7.90000000000001));
#137259=CARTESIAN_POINT('Origin',(-20.0475492979198,-3.66115750855381,-7.95000000000001));
#137260=CARTESIAN_POINT('',(-17.6180332032306,-4.82534994715961,-7.90000000000001));
#137261=CARTESIAN_POINT('',(-17.5765008460949,-4.73438257217951,-8.00000000000001));
#137262=CARTESIAN_POINT('',(-20.0683154764877,-3.70664119604381,-7.90000000000001));
#137263=CARTESIAN_POINT('Origin',(-18.0333567745876,-5.73502369695961,-7.95000000000001));
#137264=CARTESIAN_POINT('Origin',(-18.0333567745876,-5.73502369695961,-7.90000000000001));
#137265=CARTESIAN_POINT('Origin',(18.0333567325795,-5.73502369686701,-7.95000000000001));
#137266=CARTESIAN_POINT('',(17.6180331610714,-4.82534994713601,-7.90000000000001));
#137267=CARTESIAN_POINT('',(17.5765008039206,-4.73438257216291,-8.00000000000001));
#137268=CARTESIAN_POINT('Origin',(18.0333567325795,-5.73502369686701,-7.90000000000001));
#137269=CARTESIAN_POINT('Origin',(14.3009843180419,-6.28482766950221,-7.95000000000001));
#137270=CARTESIAN_POINT('',(23.403632479024,-2.18385812354831,-7.90000000000001));
#137271=CARTESIAN_POINT('',(23.3621001218732,-2.09289074857521,-8.00000000000001));
#137272=CARTESIAN_POINT('',(14.3217504966173,-6.33031135698871,-7.90000000000001));
#137273=CARTESIAN_POINT('Origin',(21.9499999789786,0.999999999999992,-7.95000000000001));
#137274=CARTESIAN_POINT('',(23.403632479024,4.18385812354829,-7.90000000000001));
#137275=CARTESIAN_POINT('',(23.3621001218732,4.09289074857519,-8.00000000000001));
#137276=CARTESIAN_POINT('Origin',(21.9499999789786,0.999999999999992,-7.90000000000001));
#137277=CARTESIAN_POINT('Origin',(11.2169186445908,9.69289860772799,-7.95000000000001));
#137278=CARTESIAN_POINT('',(17.6180331610714,6.82534994713599,-7.90000000000001));
#137279=CARTESIAN_POINT('',(17.5765008039206,6.73438257216289,-8.00000000000001));
#137280=CARTESIAN_POINT('',(11.2376848231662,9.73838229521459,-7.90000000000001));
#137281=CARTESIAN_POINT('Origin',(18.0333567325795,7.735023696867,-7.95000000000001));
#137282=CARTESIAN_POINT('Origin',(18.0333567325795,7.735023696867,-7.90000000000001));
#137283=CARTESIAN_POINT('Origin',(11.2169186448239,9.69289860762159,-6.05000000000001));
#137284=CARTESIAN_POINT('',(23.3621001218732,4.09289074857519,-6.00000000000001));
#137285=CARTESIAN_POINT('',(23.403632479024,4.18385812354829,-6.1));
#137286=CARTESIAN_POINT('',(23.3621001218732,4.09289074857519,-6.00000000000001));
#137287=CARTESIAN_POINT('',(17.6180331610714,6.82534994713599,-6.1));
#137288=CARTESIAN_POINT('',(11.2376848233993,9.73838229510809,-6.1));
#137289=CARTESIAN_POINT('',(17.5765008039206,6.73438257216289,-6.00000000000001));
#137290=CARTESIAN_POINT('',(17.6180331610714,6.82534994713599,-6.1));
#137291=CARTESIAN_POINT('',(11.1961524662485,9.64741492013499,-6.00000000000001));
#137292=CARTESIAN_POINT('Origin',(21.9499999789786,0.999999999999992,-6.05000000000001));
#137293=CARTESIAN_POINT('',(23.3621001218732,-2.09289074857521,-6.00000000000001));
#137294=CARTESIAN_POINT('',(23.403632479024,-2.18385812354831,-6.1));
#137295=CARTESIAN_POINT('',(23.3621001218732,-2.09289074857521,-6.00000000000001));
#137296=CARTESIAN_POINT('Origin',(21.9499999789786,0.999999999999992,-6.1));
#137297=CARTESIAN_POINT('Origin',(21.9499999789786,0.999999999999992,-6.00000000000001));
#137298=CARTESIAN_POINT('Origin',(14.300984318275,-6.28482766939571,-6.05000000000001));
#137299=CARTESIAN_POINT('',(17.5765008039206,-4.73438257216291,-6.00000000000001));
#137300=CARTESIAN_POINT('',(17.6180331610714,-4.82534994713601,-6.1));
#137301=CARTESIAN_POINT('',(17.5765008039206,-4.73438257216291,-6.00000000000001));
#137302=CARTESIAN_POINT('',(14.3217504968504,-6.33031135688231,-6.1));
#137303=CARTESIAN_POINT('',(14.2802181396996,-6.23934398190921,-6.00000000000001));
#137304=CARTESIAN_POINT('Origin',(18.0333567325795,-5.73502369686701,-6.05000000000001));
#137305=CARTESIAN_POINT('',(17.0028792038023,-5.35016519990321,-6.00000000000001));
#137306=CARTESIAN_POINT('',(17.0028792038023,-5.35016519990321,-6.00000000000001));
#137307=CARTESIAN_POINT('Origin',(18.0333567325795,-5.73502369686701,-6.1));
#137308=CARTESIAN_POINT('Origin',(18.0333567325795,-5.73502369686701,-6.00000000000001));
#137309=CARTESIAN_POINT('Origin',(-2.10213452200837E-8,0.999999999999992,
-6.05000000000001));
#137310=CARTESIAN_POINT('',(-17.0028792458123,-5.35016519999051,-6.00000000000001));
#137311=CARTESIAN_POINT('',(-17.0028792458123,-5.35016519999051,-6.00000000000001));
#137312=CARTESIAN_POINT('Origin',(-2.10213452200837E-8,0.999999999999992,
-6.00000000000001));
#137313=CARTESIAN_POINT('Origin',(-18.0333567745876,-5.73502369695961,-6.05000000000001));
#137314=CARTESIAN_POINT('',(-17.576500846095,-4.73438257217951,-6.00000000000001));
#137315=CARTESIAN_POINT('',(-17.6180332032306,-4.82534994715961,-6.1));
#137316=CARTESIAN_POINT('',(-17.576500846095,-4.73438257217951,-6.00000000000001));
#137317=CARTESIAN_POINT('Origin',(-18.0333567745876,-5.73502369695961,-6.1));
#137318=CARTESIAN_POINT('Origin',(-18.0333567745876,-5.73502369695961,-6.00000000000001));
#137319=CARTESIAN_POINT('Origin',(-11.2169186854654,-7.69289860705681,-6.05000000000001));
#137320=CARTESIAN_POINT('',(-23.3621001638699,-2.09289074983501,-6.00000000000001));
#137321=CARTESIAN_POINT('',(-11.1961525068975,-7.64741491956671,-6.00000000000001));
#137322=CARTESIAN_POINT('',(-23.4036325210056,-2.18385812481501,-6.1));
#137323=CARTESIAN_POINT('',(-23.3621001638699,-2.09289074983501,-6.00000000000001));
#137324=CARTESIAN_POINT('',(-11.2376848640332,-7.73838229454681,-6.1));
#137325=CARTESIAN_POINT('Origin',(-21.9500000210213,0.999999999999992,-6.05000000000001));
#137326=CARTESIAN_POINT('',(-23.3621001638699,4.09289074983499,-6.00000000000001));
#137327=CARTESIAN_POINT('',(-23.4036325210056,4.18385812481499,-6.1));
#137328=CARTESIAN_POINT('',(-23.3621001638699,4.09289074983499,-6.00000000000001));
#137329=CARTESIAN_POINT('Origin',(-21.9500000210213,0.999999999999992,-6.1));
#137330=CARTESIAN_POINT('Origin',(-21.9500000210213,0.999999999999992,-6.00000000000001));
#137331=CARTESIAN_POINT('Origin',(-14.3009843588859,8.28482766946429,-6.05000000000001));
#137332=CARTESIAN_POINT('',(-17.5765008460949,6.73438257217959,-6.00000000000001));
#137333=CARTESIAN_POINT('',(-14.280218180318,8.23934398197429,-6.00000000000001));
#137334=CARTESIAN_POINT('',(-17.6180332032306,6.82534994715959,-6.1));
#137335=CARTESIAN_POINT('',(-17.5765008460949,6.73438257217959,-6.00000000000001));
#137336=CARTESIAN_POINT('',(-14.3217505374537,8.33031135695429,-6.1));
#137337=CARTESIAN_POINT('Origin',(-18.0333567745876,7.73502369695969,-6.05000000000001));
#137338=CARTESIAN_POINT('',(-17.0028792458123,7.35016519999049,-6.00000000000001));
#137339=CARTESIAN_POINT('',(-17.0028792458123,7.35016519999049,-6.00000000000001));
#137340=CARTESIAN_POINT('Origin',(-18.0333567745876,7.73502369695969,-6.1));
#137341=CARTESIAN_POINT('Origin',(-18.0333567745876,7.73502369695969,-6.00000000000001));
#137342=CARTESIAN_POINT('Origin',(-2.10213452200837E-8,0.999999999999992,
-6.05000000000001));
#137343=CARTESIAN_POINT('',(17.0028792038023,7.35016519990319,-6.00000000000001));
#137344=CARTESIAN_POINT('',(17.0028792038023,7.35016519990319,-6.00000000000001));
#137345=CARTESIAN_POINT('Origin',(-2.10213452200837E-8,0.999999999999992,
-6.00000000000001));
#137346=CARTESIAN_POINT('Origin',(18.0333567325795,7.735023696867,-6.05000000000001));
#137347=CARTESIAN_POINT('Origin',(18.0333567325795,7.735023696867,-6.1));
#137348=CARTESIAN_POINT('Origin',(18.0333567325795,7.735023696867,-6.00000000000001));
#137349=CARTESIAN_POINT('Origin',(-21.9500000210213,0.999999999999992,-6.00000000000001));
#137350=CARTESIAN_POINT('',(-23.4036325210056,-2.18385812481501,-6.00000000000001));
#137351=CARTESIAN_POINT('',(-23.4036325210056,4.18385812481499,-6.00000000000001));
#137352=CARTESIAN_POINT('Origin',(-23.4036325210056,4.18385812481499,-6.00000000000001));
#137353=CARTESIAN_POINT('',(-17.6180332032306,6.82534994715959,-6.00000000000001));
#137354=CARTESIAN_POINT('Origin',(-18.0333567745876,7.73502369695969,-6.00000000000001));
#137355=CARTESIAN_POINT('Origin',(18.0333567325795,7.735023696867,-6.00000000000001));
#137356=CARTESIAN_POINT('',(17.6180331610714,6.82534994713599,-6.00000000000001));
#137357=CARTESIAN_POINT('Origin',(17.2355011321219,6.99999999999999,-6.00000000000001));
#137358=CARTESIAN_POINT('',(23.403632479024,4.18385812354829,-6.00000000000001));
#137359=CARTESIAN_POINT('Origin',(-2.10213446649728E-8,0.999999999999992,
-6.00000000000001));
#137360=CARTESIAN_POINT('Origin',(-18.0333567745876,-5.73502369695961,-6.00000000000001));
#137361=CARTESIAN_POINT('',(-17.6180332032306,-4.82534994715961,-6.00000000000001));
#137362=CARTESIAN_POINT('Origin',(18.0333567325795,-5.73502369686701,-6.00000000000001));
#137363=CARTESIAN_POINT('',(17.6180331610714,-4.82534994713601,-6.00000000000001));
#137364=CARTESIAN_POINT('Origin',(23.403632479024,-2.18385812354831,-6.00000000000001));
#137365=CARTESIAN_POINT('',(23.403632479024,-2.18385812354831,-6.00000000000001));
#137366=CARTESIAN_POINT('Origin',(-8.88178376686733E-15,1.00000037997959,
-0.150000000000006));
#137367=CARTESIAN_POINT('',(-1.00000000000001,1.00000037997959,-0.300000000000006));
#137368=CARTESIAN_POINT('Origin',(-8.88178376686733E-15,1.00000037997959,
-0.300000000000006));
#137369=CARTESIAN_POINT('',(-1.30000000000001,1.00000037997959,-5.55111512312578E-15));
#137370=CARTESIAN_POINT('',(-1.15000000000001,1.00000037997959,-0.150000000000006));
#137371=CARTESIAN_POINT('Origin',(-8.88178376686733E-15,1.00000037997959,
-5.55111512312578E-15));
#137372=CARTESIAN_POINT('Origin',(-8.88178376686733E-15,1.00000037997959,
-5.55111512312578E-15));
#137373=CARTESIAN_POINT('',(-1.00000000000001,1.00000037997959,-0.500000000000006));
#137374=CARTESIAN_POINT('',(-1.00000000000001,1.00000037997959,-5.55111512312578E-15));
#137375=CARTESIAN_POINT('Origin',(-8.88178376686733E-15,1.00000037997959,
-0.500000000000006));
#137376=CARTESIAN_POINT('Origin',(-8.88178376686733E-15,1.00000037997959,
-5.55111512312578E-15));
#137377=CARTESIAN_POINT('',(1.70199570552156,0.213339323115793,-5.55111512312578E-15));
#137378=CARTESIAN_POINT('',(1.83933121789749,0.63601456862469,-6.66133814775094E-15));
#137379=CARTESIAN_POINT('Origin',(-8.88178376686733E-15,1.00000037997959,
-6.66133814775094E-15));
#137380=CARTESIAN_POINT('',(2.18514148705334,0.567582069807293,-6.66133814775094E-15));
#137381=CARTESIAN_POINT('',(1.74123355294296,0.65542714523029,-6.66133814775094E-15));
#137382=CARTESIAN_POINT('',(2.99888829585913,0.91833650204669,-6.66133814775094E-15));
#137383=CARTESIAN_POINT('Ctrl Pts',(2.18514148705334,0.567582069807293,
-6.66133814775094E-15));
#137384=CARTESIAN_POINT('Ctrl Pts',(2.26527289401707,0.55964143937159,-6.66133814775094E-15));
#137385=CARTESIAN_POINT('Ctrl Pts',(2.44985190263044,0.59248302306639,-1.66533453693774E-14));
#137386=CARTESIAN_POINT('Ctrl Pts',(2.72265593195598,0.710483544687093,
-1.66533453693774E-14));
#137387=CARTESIAN_POINT('Ctrl Pts',(2.89581178365771,0.830373026122091,
-6.66133814775094E-15));
#137388=CARTESIAN_POINT('Ctrl Pts',(2.99888829585914,0.91833650204669,-6.66133814775094E-15));
#137389=CARTESIAN_POINT('',(2.99888829585914,1.08166425791249,-7.21644966006351E-15));
#137390=CARTESIAN_POINT('Origin',(-8.88178376686733E-15,1.00000037997959,
-6.66133814775094E-15));
#137391=CARTESIAN_POINT('',(2.18514148705334,1.43241869015189,-6.66133814775094E-15));
#137392=CARTESIAN_POINT('Ctrl Pts',(2.99888829585914,1.08166425791249,-6.66133814775094E-15));
#137393=CARTESIAN_POINT('Ctrl Pts',(2.88267087431383,1.18084192839999,-6.66133814775094E-15));
#137394=CARTESIAN_POINT('Ctrl Pts',(2.76068287246971,1.26224670259339,1.33226762955019E-14));
#137395=CARTESIAN_POINT('Ctrl Pts',(2.50485018029661,1.38709985462769,-3.66373598126302E-14));
#137396=CARTESIAN_POINT('Ctrl Pts',(2.33008073891961,1.44678146098259,4.32986979603811E-14));
#137397=CARTESIAN_POINT('Ctrl Pts',(2.18514148705334,1.43241869015189,-6.66133814775094E-15));
#137398=CARTESIAN_POINT('',(1.83933121789749,1.36398619133449,-6.66133814775094E-15));
#137399=CARTESIAN_POINT('',(1.74123355294296,1.34457361472889,-6.66133814775094E-15));
#137400=CARTESIAN_POINT('',(1.70199570552156,1.78666143684349,-6.66133814775094E-15));
#137401=CARTESIAN_POINT('Origin',(-8.88178376686733E-15,1.00000037997959,
-6.66133814775094E-15));
#137402=CARTESIAN_POINT('',(2.02198570368039,1.93456055863369,-6.66133814775094E-15));
#137403=CARTESIAN_POINT('',(1.61122260122708,1.74470618047739,-6.66133814775094E-15));
#137404=CARTESIAN_POINT('',(2.47415241867612,2.69663522848389,-6.66133814775094E-15));
#137405=CARTESIAN_POINT('Ctrl Pts',(2.02198570368039,1.93456055863369,-6.66133814775094E-15));
#137406=CARTESIAN_POINT('Ctrl Pts',(2.09148075916129,1.97523651292379,-6.66133814775094E-15));
#137407=CARTESIAN_POINT('Ctrl Pts',(2.22151143449857,2.11031491885179,-2.72004641033164E-14));
#137408=CARTESIAN_POINT('Ctrl Pts',(2.37285866081655,2.36613447758449,-1.66533453693774E-14));
#137409=CARTESIAN_POINT('Ctrl Pts',(2.44246540247316,2.56488442784669,-6.66133814775094E-15));
#137410=CARTESIAN_POINT('Ctrl Pts',(2.47415241867613,2.69663522848389,-6.66133814775094E-15));
#137411=CARTESIAN_POINT('',(2.3781507724882,2.82877015863239,-7.21644966006351E-15));
#137412=CARTESIAN_POINT('Origin',(-8.88178376686733E-15,1.00000037997959,
-6.66133814775094E-15));
#137413=CARTESIAN_POINT('',(1.5136474925994,2.63422808185029,-6.66133814775094E-15));
#137414=CARTESIAN_POINT('Ctrl Pts',(2.3781507724882,2.82877015863239,-6.66133814775094E-15));
#137415=CARTESIAN_POINT('Ctrl Pts',(2.22583373134628,2.84069569307559,-6.66133814775094E-15));
#137416=CARTESIAN_POINT('Ctrl Pts',(2.07929453452094,2.83485055831319,1.33226762955019E-14));
#137417=CARTESIAN_POINT('Ctrl Pts',(1.7989342669203,2.78548400016299,-3.66373598126302E-14));
#137418=CARTESIAN_POINT('Ctrl Pts',(1.62246358563372,2.73104096226529,4.32986979603811E-14));
#137419=CARTESIAN_POINT('Ctrl Pts',(1.5136474925994,2.63422808185029,-6.66133814775094E-15));
#137420=CARTESIAN_POINT('',(1.27410472160532,2.37560285103839,-6.66133814775094E-15));
#137421=CARTESIAN_POINT('',(1.20615246978637,2.30223738591519,-6.66133814775094E-15));
#137422=CARTESIAN_POINT('',(0.914555682342743,2.63683051896609,-5.55111512312578E-15));
#137423=CARTESIAN_POINT('Origin',(-8.88178376686733E-15,1.00000037997959,
-6.66133814775094E-15));
#137424=CARTESIAN_POINT('',(1.08650010626791,2.94456882374649,-5.55111512312578E-15));
#137425=CARTESIAN_POINT('',(0.865779379284463,2.54953291155349,-5.55111512312578E-15));
#137426=CARTESIAN_POINT('',(1.00437441090659,3.82687710928989,-5.55111512312578E-15));
#137427=CARTESIAN_POINT('Ctrl Pts',(1.08650010626791,2.94456882374649,-5.55111512312578E-15));
#137428=CARTESIAN_POINT('Ctrl Pts',(1.11881406112232,3.01832453074849,-5.55111512312578E-15));
#137429=CARTESIAN_POINT('Ctrl Pts',(1.14461503405761,3.20403080265529,-2.60902410786912E-14));
#137430=CARTESIAN_POINT('Ctrl Pts',(1.11669065572569,3.49995129618689,-5.55111512312578E-15));
#137431=CARTESIAN_POINT('Ctrl Pts',(1.05618025388954,3.70166331173879,-5.55111512312578E-15));
#137432=CARTESIAN_POINT('Ctrl Pts',(1.00437441090659,3.82687710928989,-5.55111512312578E-15));
#137433=CARTESIAN_POINT('',(0.849040484398591,3.87734816150549,-6.10622663543835E-15));
#137434=CARTESIAN_POINT('Origin',(-8.88178376686733E-15,1.00000037997959,
-5.55111512312578E-15));
#137435=CARTESIAN_POINT('',(0.263991602958535,3.21181803679069,-5.55111512312578E-15));
#137436=CARTESIAN_POINT('Ctrl Pts',(0.849040484398591,3.87734816150549,
-5.55111512312578E-15));
#137437=CARTESIAN_POINT('Ctrl Pts',(0.71880375631047,3.79746641108109,-5.55111512312578E-15));
#137438=CARTESIAN_POINT('Ctrl Pts',(0.603686786061961,3.70660417322209,
1.4432899320127E-14));
#137439=CARTESIAN_POINT('Ctrl Pts',(0.405887597345406,3.50187433061819,
-3.5527136788005E-14));
#137440=CARTESIAN_POINT('Ctrl Pts',(0.295120488144862,3.35410179701789,
4.44089209850062E-14));
#137441=CARTESIAN_POINT('Ctrl Pts',(0.263991602958535,3.21181803679069,
-5.55111512312578E-15));
#137442=CARTESIAN_POINT('',(0.222213526886636,2.86178612180609,-5.55111512312578E-15));
#137443=CARTESIAN_POINT('',(0.210362138786015,2.76249088224209,-5.55111512312578E-15));
#137444=CARTESIAN_POINT('',(-0.222213526886654,2.86178612180609,-6.66133814775094E-15));
#137445=CARTESIAN_POINT('Origin',(-8.88178376686733E-15,1.00000037997959,
-6.66133814775094E-15));
#137446=CARTESIAN_POINT('',(-0.263991602958553,3.21181803679069,-6.66133814775094E-15));
#137447=CARTESIAN_POINT('',(-0.210362138786033,2.76249088224209,-6.66133814775094E-15));
#137448=CARTESIAN_POINT('',(-0.849040484398609,3.87734816150549,-6.66133814775094E-15));
#137449=CARTESIAN_POINT('Ctrl Pts',(-0.263991602958553,3.21181803679069,
-6.66133814775094E-15));
#137450=CARTESIAN_POINT('Ctrl Pts',(-0.28120158117407,3.29048132329419,
-6.66133814775094E-15));
#137451=CARTESIAN_POINT('Ctrl Pts',(-0.369482464710247,3.45588532446969,
-2.72004641033164E-14));
#137452=CARTESIAN_POINT('Ctrl Pts',(-0.566011153087274,3.67887612480449,
-1.66533453693774E-14));
#137453=CARTESIAN_POINT('Ctrl Pts',(-0.733529853433388,3.80649878184449,
-6.66133814775094E-15));
#137454=CARTESIAN_POINT('Ctrl Pts',(-0.849040484398609,3.87734816150549,
-6.66133814775094E-15));
#137455=CARTESIAN_POINT('',(-1.00437441090661,3.82687710928989,-7.21644966006351E-15));
#137456=CARTESIAN_POINT('Origin',(-8.88178376686733E-15,1.00000037997959,
-6.66133814775094E-15));
#137457=CARTESIAN_POINT('',(-1.08650010626793,2.94456882374649,-6.66133814775094E-15));
#137458=CARTESIAN_POINT('Ctrl Pts',(-1.00437441090661,3.82687710928989,
-6.66133814775094E-15));
#137459=CARTESIAN_POINT('Ctrl Pts',(-1.06278482239486,3.68570018757899,
-6.66133814775094E-15));
#137460=CARTESIAN_POINT('Ctrl Pts',(-1.1025089125507,3.54452700216369,1.33226762955019E-14));
#137461=CARTESIAN_POINT('Ctrl Pts',(-1.14219463053897,3.26263359077969,
-3.66373598126302E-14));
#137462=CARTESIAN_POINT('Ctrl Pts',(-1.14494860503893,3.07797590342699,
4.32986979603811E-14));
#137463=CARTESIAN_POINT('Ctrl Pts',(-1.08650010626793,2.94456882374649,
-6.66133814775094E-15));
#137464=CARTESIAN_POINT('',(-0.914555682342761,2.63683051896609,-6.66133814775094E-15));
#137465=CARTESIAN_POINT('',(-0.86577937928448,2.54953291155349,-6.66133814775094E-15));
#137466=CARTESIAN_POINT('',(-1.27410472160534,2.37560285103839,-6.66133814775094E-15));
#137467=CARTESIAN_POINT('Origin',(-8.88178376686733E-15,1.00000037997959,
-6.66133814775094E-15));
#137468=CARTESIAN_POINT('',(-1.51364749259942,2.63422808185029,-6.66133814775094E-15));
#137469=CARTESIAN_POINT('',(-1.20615246978639,2.30223738591519,-6.66133814775094E-15));
#137470=CARTESIAN_POINT('',(-2.37815077248822,2.82877015863239,-6.66133814775094E-15));
#137471=CARTESIAN_POINT('Ctrl Pts',(-1.51364749259942,2.63422808185029,
-6.66133814775094E-15));
#137472=CARTESIAN_POINT('Ctrl Pts',(-1.57380777715219,2.68775224607759,
-6.66133814775094E-15));
#137473=CARTESIAN_POINT('Ctrl Pts',(-1.74245715676096,2.76967728864719,
-2.72004641033164E-14));
#137474=CARTESIAN_POINT('Ctrl Pts',(-2.03252503861004,2.83456450287859,
-1.66533453693774E-14));
#137475=CARTESIAN_POINT('Ctrl Pts',(-2.2430564885075,2.83934725180989,-6.66133814775094E-15));
#137476=CARTESIAN_POINT('Ctrl Pts',(-2.37815077248822,2.82877015863239,
-6.66133814775094E-15));
#137477=CARTESIAN_POINT('',(-2.47415241867615,2.69663522848389,-7.21644966006351E-15));
#137478=CARTESIAN_POINT('Origin',(-8.88178376686733E-15,1.00000037997959,
-6.66133814775094E-15));
#137479=CARTESIAN_POINT('',(-2.02198570368041,1.93456055863369,-6.66133814775094E-15));
#137480=CARTESIAN_POINT('Ctrl Pts',(-2.47415241867615,2.69663522848389,
-6.66133814775094E-15));
#137481=CARTESIAN_POINT('Ctrl Pts',(-2.43842572167288,2.54808792115299,
-6.66133814775094E-15));
#137482=CARTESIAN_POINT('Ctrl Pts',(-2.38758357586867,2.41052711593049,
1.33226762955019E-14));
#137483=CARTESIAN_POINT('Ctrl Pts',(-2.25399711176357,2.15914377278389,
-3.66373598126302E-14));
#137484=CARTESIAN_POINT('Ctrl Pts',(-2.14768624646963,2.00813398766899,
4.32986979603811E-14));
#137485=CARTESIAN_POINT('Ctrl Pts',(-2.02198570368042,1.93456055863379,
-6.66133814775094E-15));
#137486=CARTESIAN_POINT('',(-1.70199570552158,1.78666143684349,-6.66133814775094E-15));
#137487=CARTESIAN_POINT('',(-1.6112226012271,1.74470618047739,-6.66133814775094E-15));
#137488=CARTESIAN_POINT('',(-1.83933121789751,1.36398619133449,-6.66133814775094E-15));
#137489=CARTESIAN_POINT('Origin',(-8.88178376686733E-15,1.00000037997959,
-6.66133814775094E-15));
#137490=CARTESIAN_POINT('',(-2.18514148705336,1.43241869015189,-6.66133814775094E-15));
#137491=CARTESIAN_POINT('',(-1.74123355294298,1.34457361472889,-6.66133814775094E-15));
#137492=CARTESIAN_POINT('',(-2.99888829585915,1.08166425791249,-6.66133814775094E-15));
#137493=CARTESIAN_POINT('Ctrl Pts',(-2.18514148705336,1.43241869015189,
-6.66133814775094E-15));
#137494=CARTESIAN_POINT('Ctrl Pts',(-2.26527289401709,1.44035932058759,
-6.66133814775094E-15));
#137495=CARTESIAN_POINT('Ctrl Pts',(-2.4498539131878,1.40751653520809,-2.72004641033164E-14));
#137496=CARTESIAN_POINT('Ctrl Pts',(-2.72265866540928,1.28951572275389,
-6.66133814775094E-15));
#137497=CARTESIAN_POINT('Ctrl Pts',(-2.89581178365773,1.16962773383709,
-6.66133814775094E-15));
#137498=CARTESIAN_POINT('Ctrl Pts',(-2.99888829585916,1.08166425791249,
-6.66133814775094E-15));
#137499=CARTESIAN_POINT('',(-2.99888829585916,0.91833650204669,-7.21644966006351E-15));
#137500=CARTESIAN_POINT('Origin',(-8.88178376686733E-15,1.00000037997959,
-6.66133814775094E-15));
#137501=CARTESIAN_POINT('',(-2.18514148705336,0.567582069807293,-6.66133814775094E-15));
#137502=CARTESIAN_POINT('Ctrl Pts',(-2.99888829585916,0.91833650204669,
-6.66133814775094E-15));
#137503=CARTESIAN_POINT('Ctrl Pts',(-2.88267087431385,0.81915883155919,
-6.66133814775094E-15));
#137504=CARTESIAN_POINT('Ctrl Pts',(-2.76068292952053,0.737754056010891,
1.33226762955019E-14));
#137505=CARTESIAN_POINT('Ctrl Pts',(-2.50485030710536,0.61290091813639,
-3.66373598126302E-14));
#137506=CARTESIAN_POINT('Ctrl Pts',(-2.33008073891963,0.553219298973793,
4.32986979603811E-14));
#137507=CARTESIAN_POINT('Ctrl Pts',(-2.18514148705336,0.567582069807391,
-6.66133814775094E-15));
#137508=CARTESIAN_POINT('',(-1.83933121789751,0.63601456862469,-6.66133814775094E-15));
#137509=CARTESIAN_POINT('',(-1.74123355294298,0.65542714523029,-6.66133814775094E-15));
#137510=CARTESIAN_POINT('',(-1.70199570552158,0.213339323115793,-5.55111512312578E-15));
#137511=CARTESIAN_POINT('Origin',(-8.88178376686733E-15,1.00000037997959,
-6.66133814775094E-15));
#137512=CARTESIAN_POINT('',(-2.02198570368041,0.0654402013254929,-5.55111512312578E-15));
#137513=CARTESIAN_POINT('',(-1.6112226012271,0.255294579481791,-5.55111512312578E-15));
#137514=CARTESIAN_POINT('',(-2.47415241867615,-0.696634468524611,-5.55111512312578E-15));
#137515=CARTESIAN_POINT('Ctrl Pts',(-2.02198570368041,0.0654402013254929,
-5.55111512312578E-15));
#137516=CARTESIAN_POINT('Ctrl Pts',(-2.09148075916131,0.0247642470353915,
-5.55111512312578E-15));
#137517=CARTESIAN_POINT('Ctrl Pts',(-2.22149393751475,-0.110273189124808,
-2.60902410786912E-14));
#137518=CARTESIAN_POINT('Ctrl Pts',(-2.37283326403248,-0.366080159665607,
-5.55111512312578E-15));
#137519=CARTESIAN_POINT('Ctrl Pts',(-2.44246540247318,-0.564883667887508,
-5.55111512312578E-15));
#137520=CARTESIAN_POINT('Ctrl Pts',(-2.47415241867615,-0.696634468524611,
-5.55111512312578E-15));
#137521=CARTESIAN_POINT('',(-2.37815077248822,-0.82876939867321,-6.10622663543836E-15));
#137522=CARTESIAN_POINT('Origin',(-8.88178376686733E-15,1.00000037997959,
-5.55111512312578E-15));
#137523=CARTESIAN_POINT('',(-1.51364749259942,-0.634227321891108,-5.55111512312578E-15));
#137524=CARTESIAN_POINT('Ctrl Pts',(-2.37815077248822,-0.82876939867321,
-5.55111512312578E-15));
#137525=CARTESIAN_POINT('Ctrl Pts',(-2.2258337313463,-0.84069493311631,
-5.55111512312578E-15));
#137526=CARTESIAN_POINT('Ctrl Pts',(-2.07929557892755,-0.834850597287109,
1.4432899320127E-14));
#137527=CARTESIAN_POINT('Ctrl Pts',(-1.79893681959492,-0.785484727221708,
-3.5527136788005E-14));
#137528=CARTESIAN_POINT('Ctrl Pts',(-1.62246358563374,-0.731040202306308,
4.44089209850062E-14));
#137529=CARTESIAN_POINT('Ctrl Pts',(-1.51364749259942,-0.634227321891108,
-5.55111512312578E-15));
#137530=CARTESIAN_POINT('',(-1.27410472160534,-0.375602091079212,-5.55111512312578E-15));
#137531=CARTESIAN_POINT('',(-1.20615246978639,-0.302236625956009,-5.55111512312578E-15));
#137532=CARTESIAN_POINT('',(-0.914555682342761,-0.636829759006909,-6.66133814775094E-15));
#137533=CARTESIAN_POINT('Origin',(-8.88178376686733E-15,1.00000037997959,
-6.66133814775094E-15));
#137534=CARTESIAN_POINT('',(-1.08650010626793,-0.944568063787212,-6.66133814775094E-15));
#137535=CARTESIAN_POINT('',(-0.865779379284481,-0.54953215159431,-6.66133814775094E-15));
#137536=CARTESIAN_POINT('',(-1.00437441090661,-1.82687634933071,-6.66133814775094E-15));
#137537=CARTESIAN_POINT('Ctrl Pts',(-1.08650010626793,-0.944568063787212,
-6.66133814775094E-15));
#137538=CARTESIAN_POINT('Ctrl Pts',(-1.11881406112234,-1.01832377078921,
-6.66133814775094E-15));
#137539=CARTESIAN_POINT('Ctrl Pts',(-1.14463100585987,-1.20396029950631,
-2.72004641033164E-14));
#137540=CARTESIAN_POINT('Ctrl Pts',(-1.11670822644255,-1.49985676817681,
-1.66533453693774E-14));
#137541=CARTESIAN_POINT('Ctrl Pts',(-1.05618025388956,-1.70166255177951,
-6.66133814775094E-15));
#137542=CARTESIAN_POINT('Ctrl Pts',(-1.00437441090661,-1.82687634933071,
-6.66133814775094E-15));
#137543=CARTESIAN_POINT('',(-0.849040484398609,-1.87734740154631,-7.21644966006351E-15));
#137544=CARTESIAN_POINT('Origin',(-8.88178376686733E-15,1.00000037997959,
-6.66133814775094E-15));
#137545=CARTESIAN_POINT('',(-0.263991602958553,-1.21181727683151,-6.66133814775094E-15));
#137546=CARTESIAN_POINT('Ctrl Pts',(-0.849040484398609,-1.87734740154631,
-6.66133814775094E-15));
#137547=CARTESIAN_POINT('Ctrl Pts',(-0.718803756310478,-1.79746565112191,
-6.66133814775094E-15));
#137548=CARTESIAN_POINT('Ctrl Pts',(-0.603687404582928,-1.70660550831901,
1.33226762955019E-14));
#137549=CARTESIAN_POINT('Ctrl Pts',(-0.405889607552643,-1.50187812695961,
-3.66373598126302E-14));
#137550=CARTESIAN_POINT('Ctrl Pts',(-0.295120488144882,-1.35410103706051,
4.32986979603811E-14));
#137551=CARTESIAN_POINT('Ctrl Pts',(-0.263991602958552,-1.21181727683151,
-6.66133814775094E-15));
#137552=CARTESIAN_POINT('',(-0.222213526886654,-0.861785361846907,-6.66133814775094E-15));
#137553=CARTESIAN_POINT('',(-0.210362138786033,-0.762490122282808,-6.66133814775094E-15));
#137554=CARTESIAN_POINT('',(0.222213526886635,-0.861785361846907,-6.66133814775094E-15));
#137555=CARTESIAN_POINT('Origin',(-8.88178376686733E-15,1.00000037997959,
-6.66133814775094E-15));
#137556=CARTESIAN_POINT('',(0.263991602958534,-1.21181727683151,-6.66133814775094E-15));
#137557=CARTESIAN_POINT('',(0.210362138786014,-0.762490122282808,-6.66133814775094E-15));
#137558=CARTESIAN_POINT('',(0.849040484398591,-1.87734740154631,-6.66133814775094E-15));
#137559=CARTESIAN_POINT('Ctrl Pts',(0.263991602958534,-1.21181727683151,
-6.66133814775094E-15));
#137560=CARTESIAN_POINT('Ctrl Pts',(0.281201581174052,-1.29048056333501,
-6.66133814775094E-15));
#137561=CARTESIAN_POINT('Ctrl Pts',(0.369415546990755,-1.45582621508241,
-2.72004641033164E-14));
#137562=CARTESIAN_POINT('Ctrl Pts',(0.565925030419526,-1.67879393332191,
-6.66133814775094E-15));
#137563=CARTESIAN_POINT('Ctrl Pts',(0.733529853433378,-1.80649802188531,
-6.66133814775094E-15));
#137564=CARTESIAN_POINT('Ctrl Pts',(0.849040484398591,-1.87734740154631,
-6.66133814775094E-15));
#137565=CARTESIAN_POINT('',(1.00437441090659,-1.82687634933071,-7.21644966006351E-15));
#137566=CARTESIAN_POINT('Origin',(-8.88178376686733E-15,1.00000037997959,
-6.66133814775094E-15));
#137567=CARTESIAN_POINT('',(1.08650010626791,-0.944568063787212,-6.66133814775094E-15));
#137568=CARTESIAN_POINT('Ctrl Pts',(1.00437441090659,-1.82687634933071,
-6.66133814775094E-15));
#137569=CARTESIAN_POINT('Ctrl Pts',(1.06278482239484,-1.68569942761981,
-6.66133814775094E-15));
#137570=CARTESIAN_POINT('Ctrl Pts',(1.10250949831874,-1.54452789700551,
1.33226762955019E-14));
#137571=CARTESIAN_POINT('Ctrl Pts',(1.14219547135593,-1.26263671791611,
-3.66373598126302E-14));
#137572=CARTESIAN_POINT('Ctrl Pts',(1.14494860503891,-1.07797514346901,
4.32986979603811E-14));
#137573=CARTESIAN_POINT('Ctrl Pts',(1.08650010626791,-0.944568063787212,
-6.66133814775094E-15));
#137574=CARTESIAN_POINT('',(0.914555682342743,-0.636829759006909,-6.66133814775094E-15));
#137575=CARTESIAN_POINT('',(0.865779379284462,-0.54953215159431,-6.66133814775094E-15));
#137576=CARTESIAN_POINT('',(1.27410472160532,-0.375602091079212,-5.55111512312578E-15));
#137577=CARTESIAN_POINT('Origin',(-8.88178376686733E-15,1.00000037997959,
-6.66133814775094E-15));
#137578=CARTESIAN_POINT('',(1.5136474925994,-0.634227321891108,-5.55111512312578E-15));
#137579=CARTESIAN_POINT('',(1.20615246978637,-0.302236625956009,-5.55111512312578E-15));
#137580=CARTESIAN_POINT('',(2.3781507724882,-0.82876939867321,-5.55111512312578E-15));
#137581=CARTESIAN_POINT('Ctrl Pts',(1.5136474925994,-0.634227321891108,
-5.55111512312578E-15));
#137582=CARTESIAN_POINT('Ctrl Pts',(1.57380777715217,-0.687751486118411,
-5.55111512312578E-15));
#137583=CARTESIAN_POINT('Ctrl Pts',(1.74240355763935,-0.769671725923708,
-1.55431223447522E-14));
#137584=CARTESIAN_POINT('Ctrl Pts',(2.03245399589892,-0.834554549185307,
-5.55111512312578E-15));
#137585=CARTESIAN_POINT('Ctrl Pts',(2.24305648850748,-0.839346491850712,
-5.55111512312578E-15));
#137586=CARTESIAN_POINT('Ctrl Pts',(2.3781507724882,-0.82876939867321,-5.55111512312578E-15));
#137587=CARTESIAN_POINT('',(2.47415241867613,-0.696634468524611,-6.10622663543836E-15));
#137588=CARTESIAN_POINT('Origin',(-8.88178376686733E-15,1.00000037997959,
-5.55111512312578E-15));
#137589=CARTESIAN_POINT('',(2.02198570368039,0.0654402013254929,-5.55111512312578E-15));
#137590=CARTESIAN_POINT('Ctrl Pts',(2.47415241867613,-0.696634468524611,
-5.55111512312578E-15));
#137591=CARTESIAN_POINT('Ctrl Pts',(2.43842572167286,-0.548087161193807,
-5.55111512312578E-15));
#137592=CARTESIAN_POINT('Ctrl Pts',(2.38758447134345,-0.410526973901209,
1.4432899320127E-14));
#137593=CARTESIAN_POINT('Ctrl Pts',(2.2539989302801,-0.159144637220008,
-3.5527136788005E-14));
#137594=CARTESIAN_POINT('Ctrl Pts',(2.14768624646961,-0.0081332277100099,
4.44089209850062E-14));
#137595=CARTESIAN_POINT('Ctrl Pts',(2.0219857036804,0.0654402013254929,
-5.55111512312578E-15));
#137596=CARTESIAN_POINT('',(1.61122260122708,0.255294579481791,-5.55111512312578E-15));
#137597=CARTESIAN_POINT('Origin',(-8.88178376686733E-15,1.00000037997959,
-0.500000000000006));
#137598=CARTESIAN_POINT('Origin',(-8.88178376686733E-15,1.00000037997959,
-4.00000000000001));
#137599=CARTESIAN_POINT('',(0.914555682342742,-0.636829759006909,-4.00000000000001));
#137600=CARTESIAN_POINT('',(1.27410472160532,-0.375602091079212,-4.00000000000001));
#137601=CARTESIAN_POINT('Origin',(-8.88178376686733E-15,1.00000037997959,
-4.00000000000001));
#137602=CARTESIAN_POINT('',(1.0865001062679,-0.944568063787212,-4.00000000000001));
#137603=CARTESIAN_POINT('',(0.865779379284462,-0.54953215159431,-4.00000000000001));
#137604=CARTESIAN_POINT('',(1.00437441090659,-1.82687634933071,-4.00000000000001));
#137605=CARTESIAN_POINT('Ctrl Pts',(1.00437441090659,-1.82687634933071,
-4.00000000000001));
#137606=CARTESIAN_POINT('Ctrl Pts',(1.06278482239484,-1.68569942761981,
-4.00000000000001));
#137607=CARTESIAN_POINT('Ctrl Pts',(1.10250949831874,-1.54452789700551,
-3.99999999999999));
#137608=CARTESIAN_POINT('Ctrl Pts',(1.14219547135593,-1.26263671791611,
-4.00000000000004));
#137609=CARTESIAN_POINT('Ctrl Pts',(1.14494860503891,-1.07797514346901,
-3.99999999999996));
#137610=CARTESIAN_POINT('Ctrl Pts',(1.08650010626791,-0.944568063787212,
-4.00000000000001));
#137611=CARTESIAN_POINT('',(0.84904048439859,-1.87734740154631,-4.00000000000001));
#137612=CARTESIAN_POINT('Origin',(-8.88178376686733E-15,1.00000037997959,
-4.00000000000001));
#137613=CARTESIAN_POINT('',(0.263991602958534,-1.21181727683151,-4.00000000000001));
#137614=CARTESIAN_POINT('Ctrl Pts',(0.263991602958534,-1.21181727683151,
-4.00000000000001));
#137615=CARTESIAN_POINT('Ctrl Pts',(0.281201581174052,-1.29048056333501,
-4.00000000000001));
#137616=CARTESIAN_POINT('Ctrl Pts',(0.369415546990755,-1.45582621508241,
-4.00000000000003));
#137617=CARTESIAN_POINT('Ctrl Pts',(0.565925030419526,-1.67879393332191,
-4.00000000000001));
#137618=CARTESIAN_POINT('Ctrl Pts',(0.733529853433378,-1.80649802188531,
-4.00000000000001));
#137619=CARTESIAN_POINT('Ctrl Pts',(0.849040484398591,-1.87734740154631,
-4.00000000000001));
#137620=CARTESIAN_POINT('',(0.222213526886635,-0.861785361846907,-4.00000000000001));
#137621=CARTESIAN_POINT('',(0.210362138786014,-0.762490122282808,-4.00000000000001));
#137622=CARTESIAN_POINT('',(-0.222213526886654,-0.861785361846907,-4.00000000000001));
#137623=CARTESIAN_POINT('Origin',(-8.88178376686733E-15,1.00000037997959,
-4.00000000000001));
#137624=CARTESIAN_POINT('',(-0.263991602958553,-1.21181727683151,-4.00000000000001));
#137625=CARTESIAN_POINT('',(-0.210362138786033,-0.762490122282808,-4.00000000000001));
#137626=CARTESIAN_POINT('',(-0.84904048439861,-1.87734740154631,-4.00000000000001));
#137627=CARTESIAN_POINT('Ctrl Pts',(-0.84904048439861,-1.87734740154631,
-4.00000000000001));
#137628=CARTESIAN_POINT('Ctrl Pts',(-0.718803756310479,-1.79746565112191,
-4.00000000000001));
#137629=CARTESIAN_POINT('Ctrl Pts',(-0.603687404582929,-1.70660550831901,
-3.99999999999999));
#137630=CARTESIAN_POINT('Ctrl Pts',(-0.405889607552644,-1.50187812695961,
-4.00000000000004));
#137631=CARTESIAN_POINT('Ctrl Pts',(-0.295120488144883,-1.35410103706051,
-3.99999999999996));
#137632=CARTESIAN_POINT('Ctrl Pts',(-0.263991602958553,-1.21181727683151,
-4.00000000000001));
#137633=CARTESIAN_POINT('',(-1.00437441090661,-1.82687634933071,-4.00000000000001));
#137634=CARTESIAN_POINT('Origin',(-8.88178376686733E-15,1.00000037997959,
-4.00000000000001));
#137635=CARTESIAN_POINT('',(-1.08650010626793,-0.944568063787212,-4.00000000000001));
#137636=CARTESIAN_POINT('Ctrl Pts',(-1.08650010626793,-0.944568063787212,
-4.00000000000001));
#137637=CARTESIAN_POINT('Ctrl Pts',(-1.11881406112234,-1.01832377078921,
-4.00000000000001));
#137638=CARTESIAN_POINT('Ctrl Pts',(-1.14463100585987,-1.20396029950631,
-4.00000000000003));
#137639=CARTESIAN_POINT('Ctrl Pts',(-1.11670822644255,-1.49985676817681,
-4.00000000000002));
#137640=CARTESIAN_POINT('Ctrl Pts',(-1.05618025388956,-1.70166255177951,
-4.00000000000001));
#137641=CARTESIAN_POINT('Ctrl Pts',(-1.00437441090661,-1.82687634933071,
-4.00000000000001));
#137642=CARTESIAN_POINT('',(-0.914555682342761,-0.636829759006909,-4.00000000000001));
#137643=CARTESIAN_POINT('',(-0.865779379284481,-0.54953215159431,-4.00000000000001));
#137644=CARTESIAN_POINT('',(-1.27410472160534,-0.375602091079212,-4.00000000000001));
#137645=CARTESIAN_POINT('Origin',(-8.88178376686733E-15,1.00000037997959,
-4.00000000000001));
#137646=CARTESIAN_POINT('',(-1.51364749259942,-0.634227321891108,-4.00000000000001));
#137647=CARTESIAN_POINT('',(-1.20615246978639,-0.302236625956009,-4.00000000000001));
#137648=CARTESIAN_POINT('',(-2.37815077248822,-0.82876939867321,-4.00000000000001));
#137649=CARTESIAN_POINT('Ctrl Pts',(-2.37815077248822,-0.82876939867321,
-4.00000000000001));
#137650=CARTESIAN_POINT('Ctrl Pts',(-2.2258337313463,-0.84069493311631,
-4.00000000000001));
#137651=CARTESIAN_POINT('Ctrl Pts',(-2.07929557892755,-0.834850597287109,
-3.99999999999999));
#137652=CARTESIAN_POINT('Ctrl Pts',(-1.79893681959492,-0.785484727221708,
-4.00000000000004));
#137653=CARTESIAN_POINT('Ctrl Pts',(-1.62246358563374,-0.731040202306308,
-3.99999999999996));
#137654=CARTESIAN_POINT('Ctrl Pts',(-1.51364749259942,-0.634227321891108,
-4.00000000000001));
#137655=CARTESIAN_POINT('',(-2.47415241867615,-0.696634468524611,-4.00000000000001));
#137656=CARTESIAN_POINT('Origin',(-8.88178376686733E-15,1.00000037997959,
-4.00000000000001));
#137657=CARTESIAN_POINT('',(-2.02198570368041,0.0654402013254929,-4.00000000000001));
#137658=CARTESIAN_POINT('Ctrl Pts',(-2.02198570368041,0.0654402013254929,
-4.00000000000001));
#137659=CARTESIAN_POINT('Ctrl Pts',(-2.09148075916131,0.0247642470353915,
-4.00000000000001));
#137660=CARTESIAN_POINT('Ctrl Pts',(-2.22149393751475,-0.110273189124808,
-4.00000000000003));
#137661=CARTESIAN_POINT('Ctrl Pts',(-2.37283326403248,-0.366080159665607,
-4.00000000000001));
#137662=CARTESIAN_POINT('Ctrl Pts',(-2.44246540247318,-0.564883667887508,
-4.00000000000001));
#137663=CARTESIAN_POINT('Ctrl Pts',(-2.47415241867615,-0.696634468524611,
-4.00000000000001));
#137664=CARTESIAN_POINT('',(-1.70199570552158,0.213339323115793,-4.00000000000001));
#137665=CARTESIAN_POINT('',(-1.6112226012271,0.255294579481791,-4.00000000000001));
#137666=CARTESIAN_POINT('',(-1.83933121789751,0.63601456862469,-4.00000000000001));
#137667=CARTESIAN_POINT('Origin',(-8.88178376686733E-15,1.00000037997959,
-4.00000000000001));
#137668=CARTESIAN_POINT('',(-2.18514148705336,0.567582069807293,-4.00000000000001));
#137669=CARTESIAN_POINT('',(-1.74123355294298,0.65542714523029,-4.00000000000001));
#137670=CARTESIAN_POINT('',(-2.99888829585916,0.91833650204669,-4.00000000000001));
#137671=CARTESIAN_POINT('Ctrl Pts',(-2.99888829585916,0.91833650204669,
-4.00000000000001));
#137672=CARTESIAN_POINT('Ctrl Pts',(-2.88267087431385,0.81915883155919,
-4.00000000000001));
#137673=CARTESIAN_POINT('Ctrl Pts',(-2.76068292952053,0.737754056010891,
-3.99999999999999));
#137674=CARTESIAN_POINT('Ctrl Pts',(-2.50485030710536,0.61290091813639,
-4.00000000000004));
#137675=CARTESIAN_POINT('Ctrl Pts',(-2.33008073891963,0.553219298973793,
-3.99999999999996));
#137676=CARTESIAN_POINT('Ctrl Pts',(-2.18514148705336,0.567582069807391,
-4.00000000000001));
#137677=CARTESIAN_POINT('',(-2.99888829585915,1.08166425791249,-4.00000000000001));
#137678=CARTESIAN_POINT('Origin',(-8.88178376686733E-15,1.00000037997959,
-4.00000000000001));
#137679=CARTESIAN_POINT('',(-2.18514148705336,1.43241869015189,-4.00000000000001));
#137680=CARTESIAN_POINT('Ctrl Pts',(-2.18514148705336,1.43241869015189,
-4.00000000000001));
#137681=CARTESIAN_POINT('Ctrl Pts',(-2.26527289401709,1.44035932058759,
-4.00000000000001));
#137682=CARTESIAN_POINT('Ctrl Pts',(-2.4498539131878,1.40751653520809,-4.00000000000003));
#137683=CARTESIAN_POINT('Ctrl Pts',(-2.72265866540928,1.28951572275389,
-4.00000000000001));
#137684=CARTESIAN_POINT('Ctrl Pts',(-2.89581178365773,1.16962773383709,
-4.00000000000001));
#137685=CARTESIAN_POINT('Ctrl Pts',(-2.99888829585916,1.08166425791249,
-4.00000000000001));
#137686=CARTESIAN_POINT('',(-1.83933121789751,1.36398619133449,-4.00000000000001));
#137687=CARTESIAN_POINT('',(-1.74123355294298,1.34457361472889,-4.00000000000001));
#137688=CARTESIAN_POINT('',(-1.70199570552158,1.78666143684349,-4.00000000000001));
#137689=CARTESIAN_POINT('Origin',(-8.88178376686733E-15,1.00000037997959,
-4.00000000000001));
#137690=CARTESIAN_POINT('',(-2.02198570368041,1.93456055863369,-4.00000000000001));
#137691=CARTESIAN_POINT('',(-1.6112226012271,1.74470618047739,-4.00000000000001));
#137692=CARTESIAN_POINT('',(-2.47415241867615,2.69663522848389,-4.00000000000001));
#137693=CARTESIAN_POINT('Ctrl Pts',(-2.47415241867615,2.69663522848389,
-4.00000000000001));
#137694=CARTESIAN_POINT('Ctrl Pts',(-2.43842572167288,2.54808792115299,
-4.00000000000001));
#137695=CARTESIAN_POINT('Ctrl Pts',(-2.38758357586867,2.41052711593049,
-3.99999999999999));
#137696=CARTESIAN_POINT('Ctrl Pts',(-2.25399711176357,2.15914377278389,
-4.00000000000004));
#137697=CARTESIAN_POINT('Ctrl Pts',(-2.14768624646963,2.00813398766899,
-3.99999999999996));
#137698=CARTESIAN_POINT('Ctrl Pts',(-2.02198570368042,1.93456055863379,
-4.00000000000001));
#137699=CARTESIAN_POINT('',(-2.37815077248822,2.82877015863239,-4.00000000000001));
#137700=CARTESIAN_POINT('Origin',(-8.88178376686733E-15,1.00000037997959,
-4.00000000000001));
#137701=CARTESIAN_POINT('',(-1.51364749259942,2.63422808185029,-4.00000000000001));
#137702=CARTESIAN_POINT('Ctrl Pts',(-1.51364749259942,2.63422808185029,
-4.00000000000001));
#137703=CARTESIAN_POINT('Ctrl Pts',(-1.57380777715219,2.68775224607759,
-4.00000000000001));
#137704=CARTESIAN_POINT('Ctrl Pts',(-1.74245715676096,2.76967728864719,
-4.00000000000003));
#137705=CARTESIAN_POINT('Ctrl Pts',(-2.03252503861004,2.83456450287859,
-4.00000000000002));
#137706=CARTESIAN_POINT('Ctrl Pts',(-2.2430564885075,2.83934725180989,-4.00000000000001));
#137707=CARTESIAN_POINT('Ctrl Pts',(-2.37815077248822,2.82877015863239,
-4.00000000000001));
#137708=CARTESIAN_POINT('',(-1.27410472160534,2.37560285103839,-4.00000000000001));
#137709=CARTESIAN_POINT('',(-1.20615246978639,2.30223738591519,-4.00000000000001));
#137710=CARTESIAN_POINT('',(-0.914555682342761,2.63683051896609,-4.00000000000001));
#137711=CARTESIAN_POINT('Origin',(-8.88178376686733E-15,1.00000037997959,
-4.00000000000001));
#137712=CARTESIAN_POINT('',(-1.08650010626793,2.94456882374649,-4.00000000000001));
#137713=CARTESIAN_POINT('',(-0.86577937928448,2.54953291155349,-4.00000000000001));
#137714=CARTESIAN_POINT('',(-1.00437441090661,3.82687710928989,-4.00000000000001));
#137715=CARTESIAN_POINT('Ctrl Pts',(-1.00437441090661,3.82687710928989,
-4.00000000000001));
#137716=CARTESIAN_POINT('Ctrl Pts',(-1.06278482239486,3.68570018757899,
-4.00000000000001));
#137717=CARTESIAN_POINT('Ctrl Pts',(-1.1025089125507,3.54452700216369,-3.99999999999999));
#137718=CARTESIAN_POINT('Ctrl Pts',(-1.14219463053897,3.26263359077969,
-4.00000000000004));
#137719=CARTESIAN_POINT('Ctrl Pts',(-1.14494860503893,3.07797590342699,
-3.99999999999996));
#137720=CARTESIAN_POINT('Ctrl Pts',(-1.08650010626793,2.94456882374649,
-4.00000000000001));
#137721=CARTESIAN_POINT('',(-0.849040484398609,3.87734816150549,-4.00000000000001));
#137722=CARTESIAN_POINT('Origin',(-8.88178376686733E-15,1.00000037997959,
-4.00000000000001));
#137723=CARTESIAN_POINT('',(-0.263991602958553,3.21181803679069,-4.00000000000001));
#137724=CARTESIAN_POINT('Ctrl Pts',(-0.263991602958553,3.21181803679069,
-4.00000000000001));
#137725=CARTESIAN_POINT('Ctrl Pts',(-0.28120158117407,3.29048132329419,
-4.00000000000001));
#137726=CARTESIAN_POINT('Ctrl Pts',(-0.369482464710247,3.45588532446969,
-4.00000000000003));
#137727=CARTESIAN_POINT('Ctrl Pts',(-0.566011153087274,3.67887612480449,
-4.00000000000002));
#137728=CARTESIAN_POINT('Ctrl Pts',(-0.733529853433388,3.80649878184449,
-4.00000000000001));
#137729=CARTESIAN_POINT('Ctrl Pts',(-0.849040484398609,3.87734816150549,
-4.00000000000001));
#137730=CARTESIAN_POINT('',(-0.222213526886653,2.86178612180609,-4.00000000000001));
#137731=CARTESIAN_POINT('',(-0.210362138786032,2.76249088224209,-4.00000000000001));
#137732=CARTESIAN_POINT('',(0.222213526886636,2.86178612180609,-4.00000000000001));
#137733=CARTESIAN_POINT('Origin',(-8.88178376686733E-15,1.00000037997959,
-4.00000000000001));
#137734=CARTESIAN_POINT('',(0.263991602958535,3.21181803679069,-4.00000000000001));
#137735=CARTESIAN_POINT('',(0.210362138786015,2.76249088224209,-4.00000000000001));
#137736=CARTESIAN_POINT('',(0.849040484398591,3.87734816150549,-4.00000000000001));
#137737=CARTESIAN_POINT('Ctrl Pts',(0.849040484398591,3.87734816150549,
-4.00000000000001));
#137738=CARTESIAN_POINT('Ctrl Pts',(0.71880375631047,3.79746641108109,-4.00000000000001));
#137739=CARTESIAN_POINT('Ctrl Pts',(0.603686786061961,3.70660417322209,
-3.99999999999999));
#137740=CARTESIAN_POINT('Ctrl Pts',(0.405887597345406,3.50187433061819,
-4.00000000000004));
#137741=CARTESIAN_POINT('Ctrl Pts',(0.295120488144862,3.35410179701789,
-3.99999999999996));
#137742=CARTESIAN_POINT('Ctrl Pts',(0.263991602958535,3.21181803679069,
-4.00000000000001));
#137743=CARTESIAN_POINT('',(1.00437441090659,3.82687710928989,-4.00000000000001));
#137744=CARTESIAN_POINT('Origin',(-8.88178376686733E-15,1.00000037997959,
-4.00000000000001));
#137745=CARTESIAN_POINT('',(1.08650010626791,2.94456882374649,-4.00000000000001));
#137746=CARTESIAN_POINT('Ctrl Pts',(1.08650010626791,2.94456882374649,-4.00000000000001));
#137747=CARTESIAN_POINT('Ctrl Pts',(1.11881406112232,3.01832453074849,-4.00000000000001));
#137748=CARTESIAN_POINT('Ctrl Pts',(1.14461503405761,3.20403080265529,-4.00000000000003));
#137749=CARTESIAN_POINT('Ctrl Pts',(1.11669065572569,3.49995129618689,-4.00000000000001));
#137750=CARTESIAN_POINT('Ctrl Pts',(1.05618025388954,3.70166331173879,-4.00000000000001));
#137751=CARTESIAN_POINT('Ctrl Pts',(1.00437441090659,3.82687710928989,-4.00000000000001));
#137752=CARTESIAN_POINT('',(0.914555682342743,2.63683051896609,-4.00000000000001));
#137753=CARTESIAN_POINT('',(0.865779379284463,2.54953291155349,-4.00000000000001));
#137754=CARTESIAN_POINT('',(1.27410472160532,2.37560285103839,-4.00000000000001));
#137755=CARTESIAN_POINT('Origin',(-8.88178376686733E-15,1.00000037997959,
-4.00000000000001));
#137756=CARTESIAN_POINT('',(1.5136474925994,2.63422808185029,-4.00000000000001));
#137757=CARTESIAN_POINT('',(1.20615246978637,2.30223738591519,-4.00000000000001));
#137758=CARTESIAN_POINT('',(2.3781507724882,2.82877015863239,-4.00000000000001));
#137759=CARTESIAN_POINT('Ctrl Pts',(2.3781507724882,2.82877015863239,-4.00000000000001));
#137760=CARTESIAN_POINT('Ctrl Pts',(2.22583373134628,2.84069569307559,-4.00000000000001));
#137761=CARTESIAN_POINT('Ctrl Pts',(2.07929453452094,2.83485055831319,-3.99999999999999));
#137762=CARTESIAN_POINT('Ctrl Pts',(1.7989342669203,2.78548400016299,-4.00000000000004));
#137763=CARTESIAN_POINT('Ctrl Pts',(1.62246358563372,2.73104096226529,-3.99999999999996));
#137764=CARTESIAN_POINT('Ctrl Pts',(1.5136474925994,2.63422808185029,-4.00000000000001));
#137765=CARTESIAN_POINT('',(2.47415241867612,2.69663522848389,-4.00000000000001));
#137766=CARTESIAN_POINT('Origin',(-8.88178376686733E-15,1.00000037997959,
-4.00000000000001));
#137767=CARTESIAN_POINT('',(2.02198570368039,1.93456055863369,-4.00000000000001));
#137768=CARTESIAN_POINT('Ctrl Pts',(2.02198570368039,1.93456055863369,-4.00000000000001));
#137769=CARTESIAN_POINT('Ctrl Pts',(2.09148075916129,1.97523651292379,-4.00000000000001));
#137770=CARTESIAN_POINT('Ctrl Pts',(2.22151143449857,2.11031491885179,-4.00000000000003));
#137771=CARTESIAN_POINT('Ctrl Pts',(2.37285866081655,2.36613447758449,-4.00000000000002));
#137772=CARTESIAN_POINT('Ctrl Pts',(2.44246540247316,2.56488442784669,-4.00000000000001));
#137773=CARTESIAN_POINT('Ctrl Pts',(2.47415241867613,2.69663522848389,-4.00000000000001));
#137774=CARTESIAN_POINT('',(1.70199570552156,1.78666143684349,-4.00000000000001));
#137775=CARTESIAN_POINT('',(1.61122260122708,1.74470618047739,-4.00000000000001));
#137776=CARTESIAN_POINT('',(1.83933121789749,1.36398619133449,-4.00000000000001));
#137777=CARTESIAN_POINT('Origin',(-8.88178376686733E-15,1.00000037997959,
-4.00000000000001));
#137778=CARTESIAN_POINT('',(2.18514148705334,1.43241869015189,-4.00000000000001));
#137779=CARTESIAN_POINT('',(1.74123355294296,1.34457361472889,-4.00000000000001));
#137780=CARTESIAN_POINT('',(2.99888829585914,1.08166425791249,-4.00000000000001));
#137781=CARTESIAN_POINT('Ctrl Pts',(2.99888829585914,1.08166425791249,-4.00000000000001));
#137782=CARTESIAN_POINT('Ctrl Pts',(2.88267087431383,1.18084192839999,-4.00000000000001));
#137783=CARTESIAN_POINT('Ctrl Pts',(2.76068287246971,1.26224670259339,-3.99999999999999));
#137784=CARTESIAN_POINT('Ctrl Pts',(2.50485018029661,1.38709985462769,-4.00000000000004));
#137785=CARTESIAN_POINT('Ctrl Pts',(2.33008073891961,1.44678146098259,-3.99999999999996));
#137786=CARTESIAN_POINT('Ctrl Pts',(2.18514148705334,1.43241869015189,-4.00000000000001));
#137787=CARTESIAN_POINT('',(2.99888829585913,0.91833650204669,-4.00000000000001));
#137788=CARTESIAN_POINT('Origin',(-8.88178376686733E-15,1.00000037997959,
-4.00000000000001));
#137789=CARTESIAN_POINT('',(2.18514148705334,0.567582069807293,-4.00000000000001));
#137790=CARTESIAN_POINT('Ctrl Pts',(2.18514148705334,0.567582069807293,
-4.00000000000001));
#137791=CARTESIAN_POINT('Ctrl Pts',(2.26527289401707,0.55964143937159,-4.00000000000001));
#137792=CARTESIAN_POINT('Ctrl Pts',(2.44985190263044,0.59248302306639,-4.00000000000002));
#137793=CARTESIAN_POINT('Ctrl Pts',(2.72265593195598,0.710483544687093,
-4.00000000000002));
#137794=CARTESIAN_POINT('Ctrl Pts',(2.89581178365771,0.830373026122091,
-4.00000000000001));
#137795=CARTESIAN_POINT('Ctrl Pts',(2.99888829585914,0.91833650204669,-4.00000000000001));
#137796=CARTESIAN_POINT('',(1.83933121789749,0.63601456862469,-4.00000000000001));
#137797=CARTESIAN_POINT('',(1.74123355294296,0.65542714523029,-4.00000000000001));
#137798=CARTESIAN_POINT('',(1.70199570552156,0.213339323115793,-4.00000000000001));
#137799=CARTESIAN_POINT('Origin',(-8.88178376686733E-15,1.00000037997959,
-4.00000000000001));
#137800=CARTESIAN_POINT('',(2.02198570368039,0.0654402013254929,-4.00000000000001));
#137801=CARTESIAN_POINT('',(1.61122260122708,0.255294579481791,-4.00000000000001));
#137802=CARTESIAN_POINT('',(2.47415241867613,-0.696634468524611,-4.00000000000001));
#137803=CARTESIAN_POINT('Ctrl Pts',(2.47415241867613,-0.696634468524611,
-4.00000000000001));
#137804=CARTESIAN_POINT('Ctrl Pts',(2.43842572167286,-0.548087161193807,
-4.00000000000001));
#137805=CARTESIAN_POINT('Ctrl Pts',(2.38758447134345,-0.410526973901209,
-3.99999999999999));
#137806=CARTESIAN_POINT('Ctrl Pts',(2.2539989302801,-0.159144637220008,
-4.00000000000004));
#137807=CARTESIAN_POINT('Ctrl Pts',(2.14768624646961,-0.0081332277100099,
-3.99999999999996));
#137808=CARTESIAN_POINT('Ctrl Pts',(2.0219857036804,0.0654402013254929,
-4.00000000000001));
#137809=CARTESIAN_POINT('',(2.3781507724882,-0.82876939867321,-4.00000000000001));
#137810=CARTESIAN_POINT('Origin',(-8.88178376686733E-15,1.00000037997959,
-4.00000000000001));
#137811=CARTESIAN_POINT('',(1.5136474925994,-0.634227321891108,-4.00000000000001));
#137812=CARTESIAN_POINT('Ctrl Pts',(1.5136474925994,-0.634227321891108,
-4.00000000000001));
#137813=CARTESIAN_POINT('Ctrl Pts',(1.57380777715217,-0.687751486118411,
-4.00000000000001));
#137814=CARTESIAN_POINT('Ctrl Pts',(1.74240355763935,-0.769671725923708,
-4.00000000000002));
#137815=CARTESIAN_POINT('Ctrl Pts',(2.03245399589892,-0.834554549185307,
-4.00000000000001));
#137816=CARTESIAN_POINT('Ctrl Pts',(2.24305648850748,-0.839346491850712,
-4.00000000000001));
#137817=CARTESIAN_POINT('Ctrl Pts',(2.3781507724882,-0.82876939867321,-4.00000000000001));
#137818=CARTESIAN_POINT('',(1.20615246978637,-0.302236625956009,-4.00000000000001));
#137819=CARTESIAN_POINT('',(-1.50000000000001,1.00000037997959,-4.00000000000001));
#137820=CARTESIAN_POINT('Origin',(-8.88178376686733E-15,1.00000037997959,
-4.00000000000001));
#137821=CARTESIAN_POINT('Origin',(1.20615246978637,-0.302236625956009,-4.00000000000001));
#137822=CARTESIAN_POINT('',(1.27410472160532,-0.375602091079212,-4.00000000000001));
#137823=CARTESIAN_POINT('',(1.5136474925994,-0.634227321891108,-4.00000000000001));
#137824=CARTESIAN_POINT('Ctrl Pts',(1.5136474925994,-0.634227321891108,
-4.00000000000001));
#137825=CARTESIAN_POINT('Ctrl Pts',(1.5136474925994,-0.634227321891108,
1.75999999999999));
#137826=CARTESIAN_POINT('Ctrl Pts',(1.57380777715217,-0.687751486118411,
-4.00000000000001));
#137827=CARTESIAN_POINT('Ctrl Pts',(1.57380777715217,-0.687751486118411,
1.75999999999999));
#137828=CARTESIAN_POINT('Ctrl Pts',(1.74240355763935,-0.769671725923708,
-4.00000000000002));
#137829=CARTESIAN_POINT('Ctrl Pts',(1.74240355763935,-0.769671725923708,
1.75999999999998));
#137830=CARTESIAN_POINT('Ctrl Pts',(2.03245399589892,-0.834554549185307,
-4.00000000000001));
#137831=CARTESIAN_POINT('Ctrl Pts',(2.03245399589892,-0.834554549185307,
1.75999999999999));
#137832=CARTESIAN_POINT('Ctrl Pts',(2.24305648850748,-0.839346491850712,
-4.00000000000001));
#137833=CARTESIAN_POINT('Ctrl Pts',(2.24305648850748,-0.839346491850712,
1.75999999999999));
#137834=CARTESIAN_POINT('Ctrl Pts',(2.3781507724882,-0.82876939867321,-4.00000000000001));
#137835=CARTESIAN_POINT('Ctrl Pts',(2.3781507724882,-0.82876939867321,1.75999999999999));
#137836=CARTESIAN_POINT('',(2.3781507724882,-0.82876939867321,-5.55111512312578E-15));
#137837=CARTESIAN_POINT('Origin',(-8.88178376686733E-15,1.00000037997959,
-4.00000000000001));
#137838=CARTESIAN_POINT('',(2.47415241867613,-0.696634468524611,-4.00000000000001));
#137839=CARTESIAN_POINT('Ctrl Pts',(2.47415241867613,-0.696634468524611,
-4.00000000000001));
#137840=CARTESIAN_POINT('Ctrl Pts',(2.47415241867613,-0.696634468524611,
1.76000000000005));
#137841=CARTESIAN_POINT('Ctrl Pts',(2.43842572167286,-0.548087161193807,
-4.00000000000001));
#137842=CARTESIAN_POINT('Ctrl Pts',(2.43842572167286,-0.548087161193807,
1.76000000000005));
#137843=CARTESIAN_POINT('Ctrl Pts',(2.38758447134345,-0.410526973901209,
-3.99999999999999));
#137844=CARTESIAN_POINT('Ctrl Pts',(2.38758447134345,-0.410526973901209,
1.76000000000007));
#137845=CARTESIAN_POINT('Ctrl Pts',(2.2539989302801,-0.159144637220008,
-4.00000000000004));
#137846=CARTESIAN_POINT('Ctrl Pts',(2.2539989302801,-0.159144637220008,
1.76000000000002));
#137847=CARTESIAN_POINT('Ctrl Pts',(2.14768624646961,-0.00813322771000991,
-3.99999999999996));
#137848=CARTESIAN_POINT('Ctrl Pts',(2.14768624646961,-0.00813322771000991,
1.7600000000001));
#137849=CARTESIAN_POINT('Ctrl Pts',(2.0219857036804,0.0654402013254929,
-4.00000000000001));
#137850=CARTESIAN_POINT('Ctrl Pts',(2.0219857036804,0.0654402013254929,
1.76000000000005));
#137851=CARTESIAN_POINT('',(2.02198570368039,0.0654402013254929,-4.00000000000001));
#137852=CARTESIAN_POINT('Origin',(2.02198570368039,0.0654402013254929,-4.00000000000001));
#137853=CARTESIAN_POINT('',(1.70199570552156,0.213339323115793,-4.00000000000001));
#137854=CARTESIAN_POINT('Origin',(-8.88178376686733E-15,1.00000037997959,
-4.00000000000001));
#137855=CARTESIAN_POINT('',(0.914555682342743,-0.636829759006909,-4.00000000000001));
#137856=CARTESIAN_POINT('Origin',(-8.88178376686733E-15,1.00000037997959,
-4.00000000000001));
#137857=CARTESIAN_POINT('',(1.83933121789749,0.63601456862469,-4.00000000000001));
#137858=CARTESIAN_POINT('Origin',(0.210362138786014,-0.762490122282808,
-4.00000000000001));
#137859=CARTESIAN_POINT('',(0.222213526886635,-0.861785361846907,-4.00000000000001));
#137860=CARTESIAN_POINT('',(0.263991602958534,-1.21181727683151,-4.00000000000001));
#137861=CARTESIAN_POINT('Ctrl Pts',(0.263991602958534,-1.21181727683151,
-4.00000000000001));
#137862=CARTESIAN_POINT('Ctrl Pts',(0.263991602958534,-1.21181727683151,
1.75999999999999));
#137863=CARTESIAN_POINT('Ctrl Pts',(0.281201581174052,-1.29048056333501,
-4.00000000000001));
#137864=CARTESIAN_POINT('Ctrl Pts',(0.281201581174052,-1.29048056333501,
1.75999999999999));
#137865=CARTESIAN_POINT('Ctrl Pts',(0.369415546990755,-1.45582621508241,
-4.00000000000003));
#137866=CARTESIAN_POINT('Ctrl Pts',(0.369415546990755,-1.45582621508241,
1.75999999999997));
#137867=CARTESIAN_POINT('Ctrl Pts',(0.565925030419526,-1.67879393332191,
-4.00000000000001));
#137868=CARTESIAN_POINT('Ctrl Pts',(0.565925030419526,-1.67879393332191,
1.75999999999999));
#137869=CARTESIAN_POINT('Ctrl Pts',(0.733529853433378,-1.80649802188531,
-4.00000000000001));
#137870=CARTESIAN_POINT('Ctrl Pts',(0.733529853433378,-1.80649802188531,
1.75999999999999));
#137871=CARTESIAN_POINT('Ctrl Pts',(0.849040484398591,-1.87734740154631,
-4.00000000000001));
#137872=CARTESIAN_POINT('Ctrl Pts',(0.849040484398591,-1.87734740154631,
1.75999999999999));
#137873=CARTESIAN_POINT('',(0.849040484398591,-1.87734740154631,-6.66133814775094E-15));
#137874=CARTESIAN_POINT('Origin',(-8.88178376686733E-15,1.00000037997959,
-4.00000000000001));
#137875=CARTESIAN_POINT('',(1.00437441090659,-1.82687634933071,-4.00000000000001));
#137876=CARTESIAN_POINT('Ctrl Pts',(1.00437441090659,-1.82687634933071,
-4.00000000000001));
#137877=CARTESIAN_POINT('Ctrl Pts',(1.00437441090659,-1.82687634933071,
1.76000000000005));
#137878=CARTESIAN_POINT('Ctrl Pts',(1.06278482239484,-1.68569942761981,
-4.00000000000001));
#137879=CARTESIAN_POINT('Ctrl Pts',(1.06278482239484,-1.68569942761981,
1.76000000000005));
#137880=CARTESIAN_POINT('Ctrl Pts',(1.10250949831874,-1.54452789700551,
-3.99999999999999));
#137881=CARTESIAN_POINT('Ctrl Pts',(1.10250949831874,-1.54452789700551,
1.76000000000007));
#137882=CARTESIAN_POINT('Ctrl Pts',(1.14219547135593,-1.26263671791611,
-4.00000000000004));
#137883=CARTESIAN_POINT('Ctrl Pts',(1.14219547135593,-1.26263671791611,
1.76000000000002));
#137884=CARTESIAN_POINT('Ctrl Pts',(1.14494860503891,-1.07797514346901,
-3.99999999999996));
#137885=CARTESIAN_POINT('Ctrl Pts',(1.14494860503891,-1.07797514346901,
1.7600000000001));
#137886=CARTESIAN_POINT('Ctrl Pts',(1.08650010626791,-0.944568063787212,
-4.00000000000001));
#137887=CARTESIAN_POINT('Ctrl Pts',(1.08650010626791,-0.944568063787212,
1.76000000000005));
#137888=CARTESIAN_POINT('',(1.0865001062679,-0.944568063787212,-4.00000000000001));
#137889=CARTESIAN_POINT('Origin',(1.0865001062679,-0.944568063787212,-4.00000000000001));
#137890=CARTESIAN_POINT('Origin',(-8.88178376686733E-15,1.00000037997959,
-4.00000000000001));
#137891=CARTESIAN_POINT('',(-0.222213526886654,-0.861785361846907,-4.00000000000001));
#137892=CARTESIAN_POINT('Origin',(-0.865779379284481,-0.54953215159431,
-4.00000000000001));
#137893=CARTESIAN_POINT('',(-0.914555682342761,-0.636829759006909,-4.00000000000001));
#137894=CARTESIAN_POINT('',(-1.08650010626793,-0.944568063787212,-4.00000000000001));
#137895=CARTESIAN_POINT('Ctrl Pts',(-1.08650010626793,-0.944568063787212,
-4.00000000000001));
#137896=CARTESIAN_POINT('Ctrl Pts',(-1.08650010626793,-0.944568063787212,
1.75999999999999));
#137897=CARTESIAN_POINT('Ctrl Pts',(-1.11881406112234,-1.01832377078921,
-4.00000000000001));
#137898=CARTESIAN_POINT('Ctrl Pts',(-1.11881406112234,-1.01832377078921,
1.75999999999999));
#137899=CARTESIAN_POINT('Ctrl Pts',(-1.14463100585987,-1.20396029950631,
-4.00000000000003));
#137900=CARTESIAN_POINT('Ctrl Pts',(-1.14463100585987,-1.20396029950631,
1.75999999999997));
#137901=CARTESIAN_POINT('Ctrl Pts',(-1.11670822644255,-1.49985676817681,
-4.00000000000002));
#137902=CARTESIAN_POINT('Ctrl Pts',(-1.11670822644255,-1.49985676817681,
1.75999999999998));
#137903=CARTESIAN_POINT('Ctrl Pts',(-1.05618025388956,-1.70166255177951,
-4.00000000000001));
#137904=CARTESIAN_POINT('Ctrl Pts',(-1.05618025388956,-1.70166255177951,
1.75999999999999));
#137905=CARTESIAN_POINT('Ctrl Pts',(-1.00437441090661,-1.82687634933071,
-4.00000000000001));
#137906=CARTESIAN_POINT('Ctrl Pts',(-1.00437441090661,-1.82687634933071,
1.75999999999999));
#137907=CARTESIAN_POINT('',(-1.00437441090661,-1.82687634933071,-6.66133814775094E-15));
#137908=CARTESIAN_POINT('Origin',(-8.88178376686733E-15,1.00000037997959,
-4.00000000000001));
#137909=CARTESIAN_POINT('',(-0.84904048439861,-1.87734740154631,-4.00000000000001));
#137910=CARTESIAN_POINT('Ctrl Pts',(-0.84904048439861,-1.87734740154631,
-4.00000000000001));
#137911=CARTESIAN_POINT('Ctrl Pts',(-0.849040484398609,-1.87734740154631,
1.76000000000005));
#137912=CARTESIAN_POINT('Ctrl Pts',(-0.718803756310479,-1.79746565112191,
-4.00000000000001));
#137913=CARTESIAN_POINT('Ctrl Pts',(-0.718803756310478,-1.79746565112191,
1.76000000000005));
#137914=CARTESIAN_POINT('Ctrl Pts',(-0.603687404582929,-1.70660550831901,
-3.99999999999999));
#137915=CARTESIAN_POINT('Ctrl Pts',(-0.603687404582928,-1.70660550831901,
1.76000000000007));
#137916=CARTESIAN_POINT('Ctrl Pts',(-0.405889607552644,-1.50187812695961,
-4.00000000000004));
#137917=CARTESIAN_POINT('Ctrl Pts',(-0.405889607552643,-1.50187812695961,
1.76000000000002));
#137918=CARTESIAN_POINT('Ctrl Pts',(-0.295120488144883,-1.35410103706051,
-3.99999999999996));
#137919=CARTESIAN_POINT('Ctrl Pts',(-0.295120488144882,-1.35410103706051,
1.7600000000001));
#137920=CARTESIAN_POINT('Ctrl Pts',(-0.263991602958553,-1.21181727683151,
-4.00000000000001));
#137921=CARTESIAN_POINT('Ctrl Pts',(-0.263991602958552,-1.21181727683151,
1.76000000000005));
#137922=CARTESIAN_POINT('',(-0.263991602958553,-1.21181727683151,-4.00000000000001));
#137923=CARTESIAN_POINT('Origin',(-0.263991602958553,-1.21181727683151,
-4.00000000000001));
#137924=CARTESIAN_POINT('Origin',(-8.88178376686733E-15,1.00000037997959,
-4.00000000000001));
#137925=CARTESIAN_POINT('',(-1.27410472160534,-0.375602091079212,-4.00000000000001));
#137926=CARTESIAN_POINT('Origin',(-1.6112226012271,0.255294579481791,-4.00000000000001));
#137927=CARTESIAN_POINT('',(-1.70199570552158,0.213339323115793,-4.00000000000001));
#137928=CARTESIAN_POINT('',(-2.02198570368041,0.0654402013254929,-4.00000000000001));
#137929=CARTESIAN_POINT('Ctrl Pts',(-2.02198570368041,0.0654402013254929,
-4.00000000000001));
#137930=CARTESIAN_POINT('Ctrl Pts',(-2.02198570368041,0.0654402013254929,
1.75999999999999));
#137931=CARTESIAN_POINT('Ctrl Pts',(-2.09148075916131,0.0247642470353915,
-4.00000000000001));
#137932=CARTESIAN_POINT('Ctrl Pts',(-2.09148075916131,0.0247642470353915,
1.75999999999999));
#137933=CARTESIAN_POINT('Ctrl Pts',(-2.22149393751475,-0.110273189124808,
-4.00000000000003));
#137934=CARTESIAN_POINT('Ctrl Pts',(-2.22149393751475,-0.110273189124808,
1.75999999999997));
#137935=CARTESIAN_POINT('Ctrl Pts',(-2.37283326403248,-0.366080159665607,
-4.00000000000001));
#137936=CARTESIAN_POINT('Ctrl Pts',(-2.37283326403248,-0.366080159665607,
1.75999999999999));
#137937=CARTESIAN_POINT('Ctrl Pts',(-2.44246540247318,-0.564883667887508,
-4.00000000000001));
#137938=CARTESIAN_POINT('Ctrl Pts',(-2.44246540247318,-0.564883667887508,
1.75999999999999));
#137939=CARTESIAN_POINT('Ctrl Pts',(-2.47415241867615,-0.696634468524611,
-4.00000000000001));
#137940=CARTESIAN_POINT('Ctrl Pts',(-2.47415241867615,-0.696634468524611,
1.75999999999999));
#137941=CARTESIAN_POINT('',(-2.47415241867615,-0.696634468524611,-5.55111512312578E-15));
#137942=CARTESIAN_POINT('Origin',(-8.88178376686733E-15,1.00000037997959,
-4.00000000000001));
#137943=CARTESIAN_POINT('',(-2.37815077248822,-0.82876939867321,-4.00000000000001));
#137944=CARTESIAN_POINT('Ctrl Pts',(-2.37815077248822,-0.82876939867321,
-4.00000000000001));
#137945=CARTESIAN_POINT('Ctrl Pts',(-2.37815077248822,-0.82876939867321,
1.76000000000005));
#137946=CARTESIAN_POINT('Ctrl Pts',(-2.2258337313463,-0.84069493311631,
-4.00000000000001));
#137947=CARTESIAN_POINT('Ctrl Pts',(-2.2258337313463,-0.84069493311631,
1.76000000000005));
#137948=CARTESIAN_POINT('Ctrl Pts',(-2.07929557892755,-0.834850597287109,
-3.99999999999999));
#137949=CARTESIAN_POINT('Ctrl Pts',(-2.07929557892755,-0.834850597287109,
1.76000000000007));
#137950=CARTESIAN_POINT('Ctrl Pts',(-1.79893681959492,-0.785484727221708,
-4.00000000000004));
#137951=CARTESIAN_POINT('Ctrl Pts',(-1.79893681959492,-0.785484727221708,
1.76000000000002));
#137952=CARTESIAN_POINT('Ctrl Pts',(-1.62246358563374,-0.731040202306308,
-3.99999999999996));
#137953=CARTESIAN_POINT('Ctrl Pts',(-1.62246358563374,-0.731040202306308,
1.7600000000001));
#137954=CARTESIAN_POINT('Ctrl Pts',(-1.51364749259942,-0.634227321891108,
-4.00000000000001));
#137955=CARTESIAN_POINT('Ctrl Pts',(-1.51364749259942,-0.634227321891108,
1.76000000000005));
#137956=CARTESIAN_POINT('',(-1.51364749259942,-0.634227321891108,-4.00000000000001));
#137957=CARTESIAN_POINT('Origin',(-1.51364749259942,-0.634227321891108,
-4.00000000000001));
#137958=CARTESIAN_POINT('Origin',(-8.88178376686733E-15,1.00000037997959,
-4.00000000000001));
#137959=CARTESIAN_POINT('',(-1.83933121789751,0.63601456862469,-4.00000000000001));
#137960=CARTESIAN_POINT('Origin',(-1.74123355294298,1.34457361472889,-4.00000000000001));
#137961=CARTESIAN_POINT('',(-1.83933121789751,1.36398619133449,-4.00000000000001));
#137962=CARTESIAN_POINT('',(-2.18514148705336,1.43241869015189,-4.00000000000001));
#137963=CARTESIAN_POINT('Ctrl Pts',(-2.18514148705336,1.43241869015189,
-4.00000000000001));
#137964=CARTESIAN_POINT('Ctrl Pts',(-2.18514148705336,1.43241869015189,
1.75999999999999));
#137965=CARTESIAN_POINT('Ctrl Pts',(-2.26527289401709,1.44035932058759,
-4.00000000000001));
#137966=CARTESIAN_POINT('Ctrl Pts',(-2.26527289401709,1.44035932058759,
1.75999999999999));
#137967=CARTESIAN_POINT('Ctrl Pts',(-2.4498539131878,1.40751653520809,-4.00000000000003));
#137968=CARTESIAN_POINT('Ctrl Pts',(-2.4498539131878,1.40751653520809,1.75999999999997));
#137969=CARTESIAN_POINT('Ctrl Pts',(-2.72265866540928,1.28951572275389,
-4.00000000000001));
#137970=CARTESIAN_POINT('Ctrl Pts',(-2.72265866540928,1.28951572275389,
1.75999999999999));
#137971=CARTESIAN_POINT('Ctrl Pts',(-2.89581178365773,1.16962773383709,
-4.00000000000001));
#137972=CARTESIAN_POINT('Ctrl Pts',(-2.89581178365773,1.16962773383709,
1.75999999999999));
#137973=CARTESIAN_POINT('Ctrl Pts',(-2.99888829585916,1.08166425791249,
-4.00000000000001));
#137974=CARTESIAN_POINT('Ctrl Pts',(-2.99888829585916,1.08166425791249,
1.75999999999999));
#137975=CARTESIAN_POINT('',(-2.99888829585915,1.08166425791249,-6.66133814775094E-15));
#137976=CARTESIAN_POINT('Origin',(-8.88178376686733E-15,1.00000037997959,
-4.00000000000001));
#137977=CARTESIAN_POINT('',(-2.99888829585916,0.91833650204669,-4.00000000000001));
#137978=CARTESIAN_POINT('Ctrl Pts',(-2.99888829585916,0.91833650204669,
-4.00000000000001));
#137979=CARTESIAN_POINT('Ctrl Pts',(-2.99888829585916,0.91833650204669,
1.76000000000005));
#137980=CARTESIAN_POINT('Ctrl Pts',(-2.88267087431385,0.81915883155919,
-4.00000000000001));
#137981=CARTESIAN_POINT('Ctrl Pts',(-2.88267087431385,0.81915883155919,
1.76000000000005));
#137982=CARTESIAN_POINT('Ctrl Pts',(-2.76068292952053,0.737754056010891,
-3.99999999999999));
#137983=CARTESIAN_POINT('Ctrl Pts',(-2.76068292952053,0.737754056010891,
1.76000000000007));
#137984=CARTESIAN_POINT('Ctrl Pts',(-2.50485030710536,0.61290091813639,
-4.00000000000004));
#137985=CARTESIAN_POINT('Ctrl Pts',(-2.50485030710536,0.61290091813639,
1.76000000000002));
#137986=CARTESIAN_POINT('Ctrl Pts',(-2.33008073891963,0.553219298973793,
-3.99999999999996));
#137987=CARTESIAN_POINT('Ctrl Pts',(-2.33008073891963,0.553219298973793,
1.7600000000001));
#137988=CARTESIAN_POINT('Ctrl Pts',(-2.18514148705336,0.567582069807391,
-4.00000000000001));
#137989=CARTESIAN_POINT('Ctrl Pts',(-2.18514148705336,0.567582069807391,
1.76000000000005));
#137990=CARTESIAN_POINT('',(-2.18514148705336,0.567582069807293,-4.00000000000001));
#137991=CARTESIAN_POINT('Origin',(-2.18514148705336,0.567582069807293,-4.00000000000001));
#137992=CARTESIAN_POINT('Origin',(-8.88178376686733E-15,1.00000037997959,
-4.00000000000001));
#137993=CARTESIAN_POINT('',(-1.70199570552158,1.78666143684349,-4.00000000000001));
#137994=CARTESIAN_POINT('Origin',(-1.20615246978639,2.30223738591519,-4.00000000000001));
#137995=CARTESIAN_POINT('',(-1.27410472160534,2.37560285103839,-4.00000000000001));
#137996=CARTESIAN_POINT('',(-1.51364749259942,2.63422808185029,-4.00000000000001));
#137997=CARTESIAN_POINT('Ctrl Pts',(-1.51364749259942,2.63422808185029,
-4.00000000000001));
#137998=CARTESIAN_POINT('Ctrl Pts',(-1.51364749259942,2.63422808185029,
1.75999999999999));
#137999=CARTESIAN_POINT('Ctrl Pts',(-1.57380777715219,2.68775224607759,
-4.00000000000001));
#138000=CARTESIAN_POINT('Ctrl Pts',(-1.57380777715219,2.68775224607759,
1.75999999999999));
#138001=CARTESIAN_POINT('Ctrl Pts',(-1.74245715676096,2.76967728864719,
-4.00000000000003));
#138002=CARTESIAN_POINT('Ctrl Pts',(-1.74245715676096,2.76967728864719,
1.75999999999997));
#138003=CARTESIAN_POINT('Ctrl Pts',(-2.03252503861004,2.83456450287859,
-4.00000000000002));
#138004=CARTESIAN_POINT('Ctrl Pts',(-2.03252503861004,2.83456450287859,
1.75999999999998));
#138005=CARTESIAN_POINT('Ctrl Pts',(-2.2430564885075,2.83934725180989,-4.00000000000001));
#138006=CARTESIAN_POINT('Ctrl Pts',(-2.2430564885075,2.83934725180989,1.75999999999999));
#138007=CARTESIAN_POINT('Ctrl Pts',(-2.37815077248822,2.82877015863239,
-4.00000000000001));
#138008=CARTESIAN_POINT('Ctrl Pts',(-2.37815077248822,2.82877015863239,
1.75999999999999));
#138009=CARTESIAN_POINT('',(-2.37815077248822,2.82877015863239,-6.66133814775094E-15));
#138010=CARTESIAN_POINT('Origin',(-8.88178376686733E-15,1.00000037997959,
-4.00000000000001));
#138011=CARTESIAN_POINT('',(-2.47415241867615,2.69663522848389,-4.00000000000001));
#138012=CARTESIAN_POINT('Ctrl Pts',(-2.47415241867615,2.69663522848389,
-4.00000000000001));
#138013=CARTESIAN_POINT('Ctrl Pts',(-2.47415241867615,2.69663522848389,
1.76000000000005));
#138014=CARTESIAN_POINT('Ctrl Pts',(-2.43842572167288,2.54808792115299,
-4.00000000000001));
#138015=CARTESIAN_POINT('Ctrl Pts',(-2.43842572167288,2.54808792115299,
1.76000000000005));
#138016=CARTESIAN_POINT('Ctrl Pts',(-2.38758357586867,2.41052711593049,
-3.99999999999999));
#138017=CARTESIAN_POINT('Ctrl Pts',(-2.38758357586867,2.41052711593049,
1.76000000000007));
#138018=CARTESIAN_POINT('Ctrl Pts',(-2.25399711176357,2.15914377278389,
-4.00000000000004));
#138019=CARTESIAN_POINT('Ctrl Pts',(-2.25399711176357,2.15914377278389,
1.76000000000002));
#138020=CARTESIAN_POINT('Ctrl Pts',(-2.14768624646963,2.00813398766899,
-3.99999999999996));
#138021=CARTESIAN_POINT('Ctrl Pts',(-2.14768624646963,2.00813398766899,
1.7600000000001));
#138022=CARTESIAN_POINT('Ctrl Pts',(-2.02198570368042,1.93456055863379,
-4.00000000000001));
#138023=CARTESIAN_POINT('Ctrl Pts',(-2.02198570368042,1.93456055863379,
1.76000000000005));
#138024=CARTESIAN_POINT('',(-2.02198570368041,1.93456055863369,-4.00000000000001));
#138025=CARTESIAN_POINT('Origin',(-2.02198570368041,1.93456055863369,-4.00000000000001));
#138026=CARTESIAN_POINT('Origin',(-8.88178376686733E-15,1.00000037997959,
-4.00000000000001));
#138027=CARTESIAN_POINT('',(-0.914555682342761,2.63683051896609,-4.00000000000001));
#138028=CARTESIAN_POINT('Origin',(-0.210362138786032,2.76249088224209,-4.00000000000001));
#138029=CARTESIAN_POINT('',(-0.222213526886654,2.86178612180609,-4.00000000000001));
#138030=CARTESIAN_POINT('',(-0.263991602958553,3.21181803679069,-4.00000000000001));
#138031=CARTESIAN_POINT('Ctrl Pts',(-0.263991602958553,3.21181803679069,
-4.00000000000001));
#138032=CARTESIAN_POINT('Ctrl Pts',(-0.263991602958553,3.21181803679069,
1.75999999999999));
#138033=CARTESIAN_POINT('Ctrl Pts',(-0.28120158117407,3.29048132329419,
-4.00000000000001));
#138034=CARTESIAN_POINT('Ctrl Pts',(-0.28120158117407,3.29048132329419,
1.75999999999999));
#138035=CARTESIAN_POINT('Ctrl Pts',(-0.369482464710247,3.45588532446969,
-4.00000000000003));
#138036=CARTESIAN_POINT('Ctrl Pts',(-0.369482464710247,3.45588532446969,
1.75999999999997));
#138037=CARTESIAN_POINT('Ctrl Pts',(-0.566011153087274,3.67887612480449,
-4.00000000000002));
#138038=CARTESIAN_POINT('Ctrl Pts',(-0.566011153087274,3.67887612480449,
1.75999999999998));
#138039=CARTESIAN_POINT('Ctrl Pts',(-0.733529853433388,3.80649878184449,
-4.00000000000001));
#138040=CARTESIAN_POINT('Ctrl Pts',(-0.733529853433388,3.80649878184449,
1.75999999999999));
#138041=CARTESIAN_POINT('Ctrl Pts',(-0.849040484398609,3.87734816150549,
-4.00000000000001));
#138042=CARTESIAN_POINT('Ctrl Pts',(-0.849040484398609,3.87734816150549,
1.75999999999999));
#138043=CARTESIAN_POINT('',(-0.849040484398609,3.87734816150549,-6.66133814775094E-15));
#138044=CARTESIAN_POINT('Origin',(-8.88178376686733E-15,1.00000037997959,
-4.00000000000001));
#138045=CARTESIAN_POINT('',(-1.00437441090661,3.82687710928989,-4.00000000000001));
#138046=CARTESIAN_POINT('Ctrl Pts',(-1.00437441090661,3.82687710928989,
-4.00000000000001));
#138047=CARTESIAN_POINT('Ctrl Pts',(-1.00437441090661,3.82687710928989,
1.76000000000005));
#138048=CARTESIAN_POINT('Ctrl Pts',(-1.06278482239486,3.68570018757899,
-4.00000000000001));
#138049=CARTESIAN_POINT('Ctrl Pts',(-1.06278482239486,3.68570018757899,
1.76000000000005));
#138050=CARTESIAN_POINT('Ctrl Pts',(-1.1025089125507,3.54452700216369,-3.99999999999999));
#138051=CARTESIAN_POINT('Ctrl Pts',(-1.1025089125507,3.54452700216369,1.76000000000007));
#138052=CARTESIAN_POINT('Ctrl Pts',(-1.14219463053897,3.26263359077969,
-4.00000000000004));
#138053=CARTESIAN_POINT('Ctrl Pts',(-1.14219463053897,3.26263359077969,
1.76000000000002));
#138054=CARTESIAN_POINT('Ctrl Pts',(-1.14494860503893,3.07797590342699,
-3.99999999999996));
#138055=CARTESIAN_POINT('Ctrl Pts',(-1.14494860503893,3.07797590342699,
1.7600000000001));
#138056=CARTESIAN_POINT('Ctrl Pts',(-1.08650010626793,2.94456882374649,
-4.00000000000001));
#138057=CARTESIAN_POINT('Ctrl Pts',(-1.08650010626793,2.94456882374649,
1.76000000000005));
#138058=CARTESIAN_POINT('',(-1.08650010626792,2.94456882374639,-4.00000000000001));
#138059=CARTESIAN_POINT('Origin',(-1.08650010626793,2.94456882374649,-4.00000000000001));
#138060=CARTESIAN_POINT('Origin',(-8.88178376686733E-15,1.00000037997959,
-4.00000000000001));
#138061=CARTESIAN_POINT('',(0.222213526886636,2.86178612180609,-4.00000000000001));
#138062=CARTESIAN_POINT('Origin',(0.865779379284463,2.54953291155349,-4.00000000000001));
#138063=CARTESIAN_POINT('',(0.914555682342743,2.63683051896609,-4.00000000000001));
#138064=CARTESIAN_POINT('',(1.08650010626791,2.94456882374639,-4.00000000000001));
#138065=CARTESIAN_POINT('Ctrl Pts',(1.08650010626791,2.94456882374649,-4.00000000000001));
#138066=CARTESIAN_POINT('Ctrl Pts',(1.08650010626791,2.94456882374649,1.75999999999999));
#138067=CARTESIAN_POINT('Ctrl Pts',(1.11881406112232,3.01832453074849,-4.00000000000001));
#138068=CARTESIAN_POINT('Ctrl Pts',(1.11881406112232,3.01832453074849,1.75999999999999));
#138069=CARTESIAN_POINT('Ctrl Pts',(1.14461503405761,3.20403080265529,-4.00000000000003));
#138070=CARTESIAN_POINT('Ctrl Pts',(1.14461503405761,3.20403080265529,1.75999999999997));
#138071=CARTESIAN_POINT('Ctrl Pts',(1.11669065572569,3.49995129618689,-4.00000000000001));
#138072=CARTESIAN_POINT('Ctrl Pts',(1.11669065572569,3.49995129618689,1.75999999999999));
#138073=CARTESIAN_POINT('Ctrl Pts',(1.05618025388954,3.70166331173879,-4.00000000000001));
#138074=CARTESIAN_POINT('Ctrl Pts',(1.05618025388954,3.70166331173879,1.75999999999999));
#138075=CARTESIAN_POINT('Ctrl Pts',(1.00437441090659,3.82687710928989,-4.00000000000001));
#138076=CARTESIAN_POINT('Ctrl Pts',(1.00437441090659,3.82687710928989,1.75999999999999));
#138077=CARTESIAN_POINT('',(1.00437441090659,3.82687710928989,-5.55111512312578E-15));
#138078=CARTESIAN_POINT('Origin',(-8.88178376686733E-15,1.00000037997959,
-4.00000000000001));
#138079=CARTESIAN_POINT('',(0.849040484398591,3.87734816150549,-4.00000000000001));
#138080=CARTESIAN_POINT('Ctrl Pts',(0.849040484398591,3.87734816150549,
-4.00000000000001));
#138081=CARTESIAN_POINT('Ctrl Pts',(0.849040484398591,3.87734816150549,
1.76000000000005));
#138082=CARTESIAN_POINT('Ctrl Pts',(0.71880375631047,3.79746641108109,-4.00000000000001));
#138083=CARTESIAN_POINT('Ctrl Pts',(0.71880375631047,3.79746641108109,1.76000000000005));
#138084=CARTESIAN_POINT('Ctrl Pts',(0.603686786061961,3.70660417322209,
-3.99999999999999));
#138085=CARTESIAN_POINT('Ctrl Pts',(0.603686786061961,3.70660417322209,
1.76000000000007));
#138086=CARTESIAN_POINT('Ctrl Pts',(0.405887597345406,3.50187433061819,
-4.00000000000004));
#138087=CARTESIAN_POINT('Ctrl Pts',(0.405887597345406,3.50187433061819,
1.76000000000002));
#138088=CARTESIAN_POINT('Ctrl Pts',(0.295120488144862,3.35410179701789,
-3.99999999999996));
#138089=CARTESIAN_POINT('Ctrl Pts',(0.295120488144862,3.35410179701789,
1.7600000000001));
#138090=CARTESIAN_POINT('Ctrl Pts',(0.263991602958535,3.21181803679069,
-4.00000000000001));
#138091=CARTESIAN_POINT('Ctrl Pts',(0.263991602958535,3.21181803679069,
1.76000000000005));
#138092=CARTESIAN_POINT('',(0.263991602958535,3.21181803679069,-4.00000000000001));
#138093=CARTESIAN_POINT('Origin',(0.263991602958535,3.21181803679069,-4.00000000000001));
#138094=CARTESIAN_POINT('Origin',(-8.88178376686733E-15,1.00000037997959,
-4.00000000000001));
#138095=CARTESIAN_POINT('',(1.27410472160532,2.37560285103839,-4.00000000000001));
#138096=CARTESIAN_POINT('Origin',(1.61122260122708,1.74470618047739,-4.00000000000001));
#138097=CARTESIAN_POINT('',(1.70199570552156,1.78666143684349,-4.00000000000001));
#138098=CARTESIAN_POINT('',(2.02198570368039,1.93456055863369,-4.00000000000001));
#138099=CARTESIAN_POINT('Ctrl Pts',(2.02198570368039,1.93456055863369,-4.00000000000001));
#138100=CARTESIAN_POINT('Ctrl Pts',(2.02198570368039,1.93456055863369,1.75999999999999));
#138101=CARTESIAN_POINT('Ctrl Pts',(2.09148075916129,1.97523651292379,-4.00000000000001));
#138102=CARTESIAN_POINT('Ctrl Pts',(2.09148075916129,1.97523651292379,1.75999999999999));
#138103=CARTESIAN_POINT('Ctrl Pts',(2.22151143449857,2.11031491885179,-4.00000000000003));
#138104=CARTESIAN_POINT('Ctrl Pts',(2.22151143449857,2.11031491885179,1.75999999999997));
#138105=CARTESIAN_POINT('Ctrl Pts',(2.37285866081655,2.36613447758449,-4.00000000000002));
#138106=CARTESIAN_POINT('Ctrl Pts',(2.37285866081655,2.36613447758449,1.75999999999998));
#138107=CARTESIAN_POINT('Ctrl Pts',(2.44246540247316,2.56488442784669,-4.00000000000001));
#138108=CARTESIAN_POINT('Ctrl Pts',(2.44246540247316,2.56488442784669,1.75999999999999));
#138109=CARTESIAN_POINT('Ctrl Pts',(2.47415241867613,2.69663522848389,-4.00000000000001));
#138110=CARTESIAN_POINT('Ctrl Pts',(2.47415241867613,2.69663522848389,1.75999999999999));
#138111=CARTESIAN_POINT('',(2.47415241867612,2.69663522848389,-6.66133814775094E-15));
#138112=CARTESIAN_POINT('Origin',(-8.88178376686733E-15,1.00000037997959,
-4.00000000000001));
#138113=CARTESIAN_POINT('',(2.3781507724882,2.82877015863239,-4.00000000000001));
#138114=CARTESIAN_POINT('Ctrl Pts',(2.3781507724882,2.82877015863239,-4.00000000000001));
#138115=CARTESIAN_POINT('Ctrl Pts',(2.3781507724882,2.82877015863239,1.76000000000005));
#138116=CARTESIAN_POINT('Ctrl Pts',(2.22583373134628,2.84069569307559,-4.00000000000001));
#138117=CARTESIAN_POINT('Ctrl Pts',(2.22583373134628,2.84069569307559,1.76000000000005));
#138118=CARTESIAN_POINT('Ctrl Pts',(2.07929453452094,2.83485055831319,-3.99999999999999));
#138119=CARTESIAN_POINT('Ctrl Pts',(2.07929453452094,2.83485055831319,1.76000000000007));
#138120=CARTESIAN_POINT('Ctrl Pts',(1.7989342669203,2.78548400016299,-4.00000000000004));
#138121=CARTESIAN_POINT('Ctrl Pts',(1.7989342669203,2.78548400016299,1.76000000000002));
#138122=CARTESIAN_POINT('Ctrl Pts',(1.62246358563372,2.73104096226529,-3.99999999999996));
#138123=CARTESIAN_POINT('Ctrl Pts',(1.62246358563372,2.73104096226529,1.7600000000001));
#138124=CARTESIAN_POINT('Ctrl Pts',(1.5136474925994,2.63422808185029,-4.00000000000001));
#138125=CARTESIAN_POINT('Ctrl Pts',(1.5136474925994,2.63422808185029,1.76000000000005));
#138126=CARTESIAN_POINT('',(1.5136474925994,2.63422808185029,-4.00000000000001));
#138127=CARTESIAN_POINT('Origin',(1.5136474925994,2.63422808185029,-4.00000000000001));
#138128=CARTESIAN_POINT('Origin',(-8.88178376686733E-15,1.00000037997959,
-4.00000000000001));
#138129=CARTESIAN_POINT('',(1.83933121789749,1.36398619133449,-4.00000000000001));
#138130=CARTESIAN_POINT('Origin',(1.74123355294296,0.65542714523029,-4.00000000000001));
#138131=CARTESIAN_POINT('',(2.18514148705334,0.567582069807293,-4.00000000000001));
#138132=CARTESIAN_POINT('Ctrl Pts',(2.18514148705334,0.567582069807293,
-4.00000000000001));
#138133=CARTESIAN_POINT('Ctrl Pts',(2.18514148705334,0.567582069807293,
1.75999999999999));
#138134=CARTESIAN_POINT('Ctrl Pts',(2.26527289401707,0.55964143937159,-4.00000000000001));
#138135=CARTESIAN_POINT('Ctrl Pts',(2.26527289401707,0.55964143937159,1.75999999999999));
#138136=CARTESIAN_POINT('Ctrl Pts',(2.44985190263044,0.59248302306639,-4.00000000000002));
#138137=CARTESIAN_POINT('Ctrl Pts',(2.44985190263044,0.59248302306639,1.75999999999998));
#138138=CARTESIAN_POINT('Ctrl Pts',(2.72265593195598,0.710483544687093,
-4.00000000000002));
#138139=CARTESIAN_POINT('Ctrl Pts',(2.72265593195598,0.710483544687093,
1.75999999999998));
#138140=CARTESIAN_POINT('Ctrl Pts',(2.89581178365771,0.830373026122091,
-4.00000000000001));
#138141=CARTESIAN_POINT('Ctrl Pts',(2.89581178365771,0.830373026122091,
1.75999999999999));
#138142=CARTESIAN_POINT('Ctrl Pts',(2.99888829585914,0.91833650204669,-4.00000000000001));
#138143=CARTESIAN_POINT('Ctrl Pts',(2.99888829585914,0.91833650204669,1.75999999999999));
#138144=CARTESIAN_POINT('',(2.99888829585913,0.91833650204669,-6.66133814775094E-15));
#138145=CARTESIAN_POINT('Origin',(-8.88178376686733E-15,1.00000037997959,
-4.00000000000001));
#138146=CARTESIAN_POINT('',(2.99888829585914,1.08166425791249,-4.00000000000001));
#138147=CARTESIAN_POINT('Ctrl Pts',(2.99888829585914,1.08166425791249,-4.00000000000001));
#138148=CARTESIAN_POINT('Ctrl Pts',(2.99888829585914,1.08166425791249,1.76000000000005));
#138149=CARTESIAN_POINT('Ctrl Pts',(2.88267087431383,1.18084192839999,-4.00000000000001));
#138150=CARTESIAN_POINT('Ctrl Pts',(2.88267087431383,1.18084192839999,1.76000000000005));
#138151=CARTESIAN_POINT('Ctrl Pts',(2.76068287246971,1.26224670259339,-3.99999999999999));
#138152=CARTESIAN_POINT('Ctrl Pts',(2.76068287246971,1.26224670259339,1.76000000000007));
#138153=CARTESIAN_POINT('Ctrl Pts',(2.50485018029661,1.38709985462769,-4.00000000000004));
#138154=CARTESIAN_POINT('Ctrl Pts',(2.50485018029661,1.38709985462769,1.76000000000002));
#138155=CARTESIAN_POINT('Ctrl Pts',(2.33008073891961,1.44678146098259,-3.99999999999996));
#138156=CARTESIAN_POINT('Ctrl Pts',(2.33008073891961,1.44678146098259,1.7600000000001));
#138157=CARTESIAN_POINT('Ctrl Pts',(2.18514148705334,1.43241869015189,-4.00000000000001));
#138158=CARTESIAN_POINT('Ctrl Pts',(2.18514148705334,1.43241869015189,1.76000000000005));
#138159=CARTESIAN_POINT('',(2.18514148705334,1.43241869015189,-4.00000000000001));
#138160=CARTESIAN_POINT('Origin',(2.18514148705334,1.43241869015189,-4.00000000000001));
#138161=CARTESIAN_POINT('Origin',(-8.88178376686733E-15,1.00000037997959,
-18.425));
#138162=CARTESIAN_POINT('',(-17.5,1.00000037997959,-18.4));
#138163=CARTESIAN_POINT('',(8.13264802145921,-14.4954839996407,-18.4));
#138164=CARTESIAN_POINT('Origin',(-8.88178376686733E-15,1.00000037997959,
-18.4));
#138165=CARTESIAN_POINT('',(8.08617574705085,-14.4069383746142,-18.45));
#138166=CARTESIAN_POINT('',(8.10941188425504,-14.4512111871275,-18.425));
#138167=CARTESIAN_POINT('Origin',(4.44089252863457E-15,1.00000037997959,
-18.45));
#138168=CARTESIAN_POINT('Origin',(-8.88178376686733E-15,1.00000037997959,
-18.4));
#138169=CARTESIAN_POINT('Origin',(-8.88178376686733E-15,1.00000037997959,
-18.475));
#138170=CARTESIAN_POINT('',(-17.5,1.00000037997959,-18.5));
#138171=CARTESIAN_POINT('',(8.13264802145921,-14.4954839996407,-18.5));
#138172=CARTESIAN_POINT('Origin',(-8.88178376686733E-15,1.00000037997959,
-18.5));
#138173=CARTESIAN_POINT('',(8.10941188425504,-14.4512111871275,-18.475));
#138174=CARTESIAN_POINT('Origin',(-8.88178376686733E-15,1.00000037997959,
-18.5));
#138175=CARTESIAN_POINT('Origin',(-8.88178376686733E-15,1.00000037997959,
-10.));
#138176=CARTESIAN_POINT('',(-17.5,1.00000037997959,-17.9285714285714));
#138177=CARTESIAN_POINT('',(-17.5,1.00000037997959,-10.));
#138178=CARTESIAN_POINT('',(8.13264802145921,-14.4954839996407,-17.9285714285714));
#138179=CARTESIAN_POINT('Origin',(-8.88178376686733E-15,1.00000037997959,
-17.9285714285714));
#138180=CARTESIAN_POINT('Origin',(-8.88178376686733E-15,1.00000037997959,
-17.9285714285714));
#138181=CARTESIAN_POINT('Origin',(-8.88178376686733E-15,1.00000037997959,
-10.));
#138182=CARTESIAN_POINT('',(-17.5,1.00000037997959,-10.));
#138183=CARTESIAN_POINT('Origin',(-8.88178376686733E-15,1.00000037997959,
-17.8535714285714));
#138184=CARTESIAN_POINT('',(-17.5,1.00000037997959,-17.8285714285714));
#138185=CARTESIAN_POINT('',(8.13264802145921,-14.4954839996407,-17.8285714285714));
#138186=CARTESIAN_POINT('Origin',(-8.88178376686733E-15,1.00000037997959,
-17.8285714285714));
#138187=CARTESIAN_POINT('',(8.08617574705085,-14.4069383746142,-17.8785714285714));
#138188=CARTESIAN_POINT('',(8.10941188425504,-14.4512111871275,-17.8535714285714));
#138189=CARTESIAN_POINT('Origin',(4.44089252863457E-15,1.00000037997959,
-17.8785714285714));
#138190=CARTESIAN_POINT('Origin',(-8.88178376686733E-15,1.00000037997959,
-17.8285714285714));
#138191=CARTESIAN_POINT('Origin',(-8.88178376686733E-15,1.00000037997959,
-17.9035714285714));
#138192=CARTESIAN_POINT('',(8.10941188425504,-14.4512111871275,-17.9035714285714));
#138193=CARTESIAN_POINT('Origin',(-8.88178376686733E-15,1.00000037997959,
-10.));
#138194=CARTESIAN_POINT('',(-17.5,1.00000037997959,-17.3571428571429));
#138195=CARTESIAN_POINT('',(-17.5,1.00000037997959,-10.));
#138196=CARTESIAN_POINT('',(8.13264802145921,-14.4954839996407,-17.3571428571429));
#138197=CARTESIAN_POINT('Origin',(-8.88178376686733E-15,1.00000037997959,
-17.3571428571429));
#138198=CARTESIAN_POINT('Origin',(-8.88178376686733E-15,1.00000037997959,
-17.3571428571429));
#138199=CARTESIAN_POINT('Origin',(-8.88178376686733E-15,1.00000037997959,
-17.2821428571429));
#138200=CARTESIAN_POINT('',(-17.5,1.00000037997959,-17.2571428571429));
#138201=CARTESIAN_POINT('',(8.13264802145921,-14.4954839996407,-17.2571428571429));
#138202=CARTESIAN_POINT('Origin',(-8.88178376686733E-15,1.00000037997959,
-17.2571428571429));
#138203=CARTESIAN_POINT('',(8.08617574705085,-14.4069383746142,-17.3071428571429));
#138204=CARTESIAN_POINT('',(8.10941188425504,-14.4512111871275,-17.2821428571429));
#138205=CARTESIAN_POINT('Origin',(4.44089252863457E-15,1.00000037997959,
-17.3071428571429));
#138206=CARTESIAN_POINT('Origin',(-8.88178376686733E-15,1.00000037997959,
-17.2571428571429));
#138207=CARTESIAN_POINT('Origin',(-8.88178376686733E-15,1.00000037997959,
-17.3321428571429));
#138208=CARTESIAN_POINT('',(8.10941188425504,-14.4512111871275,-17.3321428571429));
#138209=CARTESIAN_POINT('Origin',(-8.88178376686733E-15,1.00000037997959,
-10.));
#138210=CARTESIAN_POINT('',(-17.5,1.00000037997959,-16.7857142857143));
#138211=CARTESIAN_POINT('',(-17.5,1.00000037997959,-10.));
#138212=CARTESIAN_POINT('',(8.13264802145921,-14.4954839996407,-16.7857142857143));
#138213=CARTESIAN_POINT('Origin',(-8.88178376686733E-15,1.00000037997959,
-16.7857142857143));
#138214=CARTESIAN_POINT('Origin',(-8.88178376686733E-15,1.00000037997959,
-16.7857142857143));
#138215=CARTESIAN_POINT('Origin',(-8.88178376686733E-15,1.00000037997959,
-16.7107142857143));
#138216=CARTESIAN_POINT('',(-17.5,1.00000037997959,-16.6857142857143));
#138217=CARTESIAN_POINT('',(8.13264802145921,-14.4954839996407,-16.6857142857143));
#138218=CARTESIAN_POINT('Origin',(-8.88178376686733E-15,1.00000037997959,
-16.6857142857143));
#138219=CARTESIAN_POINT('',(8.08617574705085,-14.4069383746142,-16.7357142857143));
#138220=CARTESIAN_POINT('',(8.10941188425504,-14.4512111871275,-16.7107142857143));
#138221=CARTESIAN_POINT('Origin',(4.44089252863457E-15,1.00000037997959,
-16.7357142857143));
#138222=CARTESIAN_POINT('Origin',(-8.88178376686733E-15,1.00000037997959,
-16.6857142857143));
#138223=CARTESIAN_POINT('Origin',(-8.88178376686733E-15,1.00000037997959,
-16.7607142857143));
#138224=CARTESIAN_POINT('',(8.10941188425504,-14.4512111871275,-16.7607142857143));
#138225=CARTESIAN_POINT('Origin',(-8.88178376686733E-15,1.00000037997959,
-10.));
#138226=CARTESIAN_POINT('',(-17.5,1.00000037997959,-16.2142857142857));
#138227=CARTESIAN_POINT('',(-17.5,1.00000037997959,-10.));
#138228=CARTESIAN_POINT('',(8.13264802145921,-14.4954839996407,-16.2142857142857));
#138229=CARTESIAN_POINT('Origin',(-8.88178376686733E-15,1.00000037997959,
-16.2142857142857));
#138230=CARTESIAN_POINT('Origin',(-8.88178376686733E-15,1.00000037997959,
-16.2142857142857));
#138231=CARTESIAN_POINT('Origin',(-8.88178376686733E-15,1.00000037997959,
-16.1392857142857));
#138232=CARTESIAN_POINT('',(-17.5,1.00000037997959,-16.1142857142857));
#138233=CARTESIAN_POINT('',(8.13264802145921,-14.4954839996407,-16.1142857142857));
#138234=CARTESIAN_POINT('Origin',(-8.88178376686733E-15,1.00000037997959,
-16.1142857142857));
#138235=CARTESIAN_POINT('',(8.08617574705085,-14.4069383746142,-16.1642857142857));
#138236=CARTESIAN_POINT('',(8.10941188425504,-14.4512111871275,-16.1392857142857));
#138237=CARTESIAN_POINT('Origin',(4.44089252863457E-15,1.00000037997959,
-16.1642857142857));
#138238=CARTESIAN_POINT('Origin',(-8.88178376686733E-15,1.00000037997959,
-16.1142857142857));
#138239=CARTESIAN_POINT('Origin',(-8.88178376686733E-15,1.00000037997959,
-16.1892857142857));
#138240=CARTESIAN_POINT('',(8.10941188425504,-14.4512111871275,-16.1892857142857));
#138241=CARTESIAN_POINT('Origin',(-8.88178376686733E-15,1.00000037997959,
-10.));
#138242=CARTESIAN_POINT('',(-17.5,1.00000037997959,-15.6428571428571));
#138243=CARTESIAN_POINT('',(-17.5,1.00000037997959,-10.));
#138244=CARTESIAN_POINT('',(8.13264802145921,-14.4954839996407,-15.6428571428571));
#138245=CARTESIAN_POINT('Origin',(-8.88178376686733E-15,1.00000037997959,
-15.6428571428571));
#138246=CARTESIAN_POINT('Origin',(-8.88178376686733E-15,1.00000037997959,
-15.6428571428571));
#138247=CARTESIAN_POINT('Origin',(-8.88178376686733E-15,1.00000037997959,
-15.5678571428571));
#138248=CARTESIAN_POINT('',(-17.5,1.00000037997959,-15.5428571428571));
#138249=CARTESIAN_POINT('',(8.13264802145921,-14.4954839996407,-15.5428571428571));
#138250=CARTESIAN_POINT('Origin',(-8.88178376686733E-15,1.00000037997959,
-15.5428571428571));
#138251=CARTESIAN_POINT('',(8.08617574705085,-14.4069383746142,-15.5928571428572));
#138252=CARTESIAN_POINT('',(8.10941188425504,-14.4512111871275,-15.5678571428571));
#138253=CARTESIAN_POINT('Origin',(4.44089252863457E-15,1.00000037997959,
-15.5928571428571));
#138254=CARTESIAN_POINT('Origin',(-8.88178376686733E-15,1.00000037997959,
-15.5428571428571));
#138255=CARTESIAN_POINT('Origin',(-8.88178376686733E-15,1.00000037997959,
-15.6178571428571));
#138256=CARTESIAN_POINT('',(8.10941188425504,-14.4512111871275,-15.6178571428571));
#138257=CARTESIAN_POINT('Origin',(-8.88178376686733E-15,1.00000037997959,
-10.));
#138258=CARTESIAN_POINT('',(-17.5,1.00000037997959,-15.0714285714286));
#138259=CARTESIAN_POINT('',(-17.5,1.00000037997959,-10.));
#138260=CARTESIAN_POINT('',(8.13264802145921,-14.4954839996407,-15.0714285714286));
#138261=CARTESIAN_POINT('Origin',(-8.88178376686733E-15,1.00000037997959,
-15.0714285714286));
#138262=CARTESIAN_POINT('Origin',(-8.88178376686733E-15,1.00000037997959,
-15.0714285714286));
#138263=CARTESIAN_POINT('Origin',(-8.88178376686733E-15,1.00000037997959,
-14.9964285714286));
#138264=CARTESIAN_POINT('',(-17.5,1.00000037997959,-14.9714285714286));
#138265=CARTESIAN_POINT('',(8.13264802145921,-14.4954839996407,-14.9714285714286));
#138266=CARTESIAN_POINT('Origin',(-8.88178376686733E-15,1.00000037997959,
-14.9714285714286));
#138267=CARTESIAN_POINT('',(8.08617574705085,-14.4069383746142,-15.0214285714286));
#138268=CARTESIAN_POINT('',(8.10941188425504,-14.4512111871275,-14.9964285714286));
#138269=CARTESIAN_POINT('Origin',(4.44089252863457E-15,1.00000037997959,
-15.0214285714286));
#138270=CARTESIAN_POINT('Origin',(-8.88178376686733E-15,1.00000037997959,
-14.9714285714286));
#138271=CARTESIAN_POINT('Origin',(-8.88178376686733E-15,1.00000037997959,
-15.0464285714286));
#138272=CARTESIAN_POINT('',(8.10941188425504,-14.4512111871275,-15.0464285714286));
#138273=CARTESIAN_POINT('Origin',(-8.88178376686733E-15,1.00000037997959,
-10.));
#138274=CARTESIAN_POINT('',(-17.5,1.00000037997959,-14.5));
#138275=CARTESIAN_POINT('',(-17.5,1.00000037997959,-10.));
#138276=CARTESIAN_POINT('',(8.13264802145921,-14.4954839996407,-14.5));
#138277=CARTESIAN_POINT('Origin',(-8.88178376686733E-15,1.00000037997959,
-14.5));
#138278=CARTESIAN_POINT('Origin',(-8.88178376686733E-15,1.00000037997959,
-14.5));
#138279=CARTESIAN_POINT('Origin',(-8.88178376686733E-15,1.00000037997959,
-14.425));
#138280=CARTESIAN_POINT('',(-17.5,1.00000037997959,-14.4));
#138281=CARTESIAN_POINT('',(8.13264802145921,-14.4954839996407,-14.4));
#138282=CARTESIAN_POINT('Origin',(-8.88178376686733E-15,1.00000037997959,
-14.4));
#138283=CARTESIAN_POINT('',(8.08617574705085,-14.4069383746142,-14.45));
#138284=CARTESIAN_POINT('',(8.10941188425504,-14.4512111871275,-14.425));
#138285=CARTESIAN_POINT('Origin',(4.44089252863457E-15,1.00000037997959,
-14.45));
#138286=CARTESIAN_POINT('Origin',(-8.88178376686733E-15,1.00000037997959,
-14.4));
#138287=CARTESIAN_POINT('Origin',(-8.88178376686733E-15,1.00000037997959,
-14.475));
#138288=CARTESIAN_POINT('',(8.10941188425504,-14.4512111871275,-14.475));
#138289=CARTESIAN_POINT('Origin',(-8.88178376686733E-15,1.00000037997959,
-10.));
#138290=CARTESIAN_POINT('',(-17.5,1.00000037997959,-13.9285714285714));
#138291=CARTESIAN_POINT('',(-17.5,1.00000037997959,-10.));
#138292=CARTESIAN_POINT('',(8.13264802145921,-14.4954839996407,-13.9285714285714));
#138293=CARTESIAN_POINT('Origin',(-8.88178376686733E-15,1.00000037997959,
-13.9285714285714));
#138294=CARTESIAN_POINT('Origin',(-8.88178376686733E-15,1.00000037997959,
-13.9285714285714));
#138295=CARTESIAN_POINT('Origin',(-8.88178376686733E-15,1.00000037997959,
-13.8535714285714));
#138296=CARTESIAN_POINT('',(-17.5,1.00000037997959,-13.8285714285714));
#138297=CARTESIAN_POINT('',(8.13264802145921,-14.4954839996407,-13.8285714285714));
#138298=CARTESIAN_POINT('Origin',(-8.88178376686733E-15,1.00000037997959,
-13.8285714285714));
#138299=CARTESIAN_POINT('',(8.08617574705085,-14.4069383746142,-13.8785714285714));
#138300=CARTESIAN_POINT('',(8.10941188425504,-14.4512111871275,-13.8535714285714));
#138301=CARTESIAN_POINT('Origin',(4.44089252863457E-15,1.00000037997959,
-13.8785714285714));
#138302=CARTESIAN_POINT('Origin',(-8.88178376686733E-15,1.00000037997959,
-13.8285714285714));
#138303=CARTESIAN_POINT('Origin',(-8.88178376686733E-15,1.00000037997959,
-13.9035714285714));
#138304=CARTESIAN_POINT('',(8.10941188425504,-14.4512111871275,-13.9035714285714));
#138305=CARTESIAN_POINT('Origin',(-8.88178376686733E-15,1.00000037997959,
-10.));
#138306=CARTESIAN_POINT('',(-17.5,1.00000037997959,-13.3571428571429));
#138307=CARTESIAN_POINT('',(-17.5,1.00000037997959,-10.));
#138308=CARTESIAN_POINT('',(8.13264802145921,-14.4954839996407,-13.3571428571429));
#138309=CARTESIAN_POINT('Origin',(-8.88178376686733E-15,1.00000037997959,
-13.3571428571429));
#138310=CARTESIAN_POINT('Origin',(-8.88178376686733E-15,1.00000037997959,
-13.3571428571429));
#138311=CARTESIAN_POINT('Origin',(-8.88178376686733E-15,1.00000037997959,
-13.2821428571429));
#138312=CARTESIAN_POINT('',(-17.5,1.00000037997959,-13.2571428571429));
#138313=CARTESIAN_POINT('',(8.13264802145921,-14.4954839996407,-13.2571428571429));
#138314=CARTESIAN_POINT('Origin',(-8.88178376686733E-15,1.00000037997959,
-13.2571428571429));
#138315=CARTESIAN_POINT('',(8.08617574705085,-14.4069383746142,-13.3071428571429));
#138316=CARTESIAN_POINT('',(8.10941188425504,-14.4512111871275,-13.2821428571429));
#138317=CARTESIAN_POINT('Origin',(4.44089252863457E-15,1.00000037997959,
-13.3071428571429));
#138318=CARTESIAN_POINT('Origin',(-8.88178376686733E-15,1.00000037997959,
-13.2571428571429));
#138319=CARTESIAN_POINT('Origin',(-8.88178376686733E-15,1.00000037997959,
-13.3321428571429));
#138320=CARTESIAN_POINT('',(8.10941188425504,-14.4512111871275,-13.3321428571429));
#138321=CARTESIAN_POINT('Origin',(-8.88178376686733E-15,1.00000037997959,
-10.));
#138322=CARTESIAN_POINT('',(-17.5,1.00000037997959,-12.7857142857143));
#138323=CARTESIAN_POINT('',(-17.5,1.00000037997959,-10.));
#138324=CARTESIAN_POINT('',(8.13264802145921,-14.4954839996407,-12.7857142857143));
#138325=CARTESIAN_POINT('Origin',(-8.88178376686733E-15,1.00000037997959,
-12.7857142857143));
#138326=CARTESIAN_POINT('Origin',(-8.88178376686733E-15,1.00000037997959,
-12.7857142857143));
#138327=CARTESIAN_POINT('Origin',(-8.88178376686733E-15,1.00000037997959,
-12.7107142857143));
#138328=CARTESIAN_POINT('',(-17.5,1.00000037997959,-12.6857142857143));
#138329=CARTESIAN_POINT('',(8.13264802145921,-14.4954839996407,-12.6857142857143));
#138330=CARTESIAN_POINT('Origin',(-8.88178376686733E-15,1.00000037997959,
-12.6857142857143));
#138331=CARTESIAN_POINT('',(8.08617574705085,-14.4069383746142,-12.7357142857143));
#138332=CARTESIAN_POINT('',(8.10941188425504,-14.4512111871275,-12.7107142857143));
#138333=CARTESIAN_POINT('Origin',(4.44089252863457E-15,1.00000037997959,
-12.7357142857143));
#138334=CARTESIAN_POINT('Origin',(-8.88178376686733E-15,1.00000037997959,
-12.6857142857143));
#138335=CARTESIAN_POINT('Origin',(-8.88178376686733E-15,1.00000037997959,
-12.7607142857143));
#138336=CARTESIAN_POINT('',(8.10941188425504,-14.4512111871275,-12.7607142857143));
#138337=CARTESIAN_POINT('Origin',(-8.88178376686733E-15,1.00000037997959,
-10.));
#138338=CARTESIAN_POINT('',(-17.5,1.00000037997959,-12.2142857142857));
#138339=CARTESIAN_POINT('',(-17.5,1.00000037997959,-10.));
#138340=CARTESIAN_POINT('',(8.13264802145921,-14.4954839996407,-12.2142857142857));
#138341=CARTESIAN_POINT('Origin',(-8.88178376686733E-15,1.00000037997959,
-12.2142857142857));
#138342=CARTESIAN_POINT('Origin',(-8.88178376686733E-15,1.00000037997959,
-12.2142857142857));
#138343=CARTESIAN_POINT('Origin',(-8.88178376686733E-15,1.00000037997959,
-12.1392857142857));
#138344=CARTESIAN_POINT('',(-17.5,1.00000037997959,-12.1142857142857));
#138345=CARTESIAN_POINT('',(8.13264802145921,-14.4954839996407,-12.1142857142857));
#138346=CARTESIAN_POINT('Origin',(-8.88178376686733E-15,1.00000037997959,
-12.1142857142857));
#138347=CARTESIAN_POINT('',(8.08617574705085,-14.4069383746142,-12.1642857142857));
#138348=CARTESIAN_POINT('',(8.10941188425504,-14.4512111871275,-12.1392857142857));
#138349=CARTESIAN_POINT('Origin',(4.44089252863457E-15,1.00000037997959,
-12.1642857142857));
#138350=CARTESIAN_POINT('Origin',(-8.88178376686733E-15,1.00000037997959,
-12.1142857142857));
#138351=CARTESIAN_POINT('Origin',(-8.88178376686733E-15,1.00000037997959,
-12.1892857142857));
#138352=CARTESIAN_POINT('',(8.10941188425504,-14.4512111871275,-12.1892857142857));
#138353=CARTESIAN_POINT('Origin',(-8.88178376686733E-15,1.00000037997959,
-10.));
#138354=CARTESIAN_POINT('',(-17.5,1.00000037997959,-11.6428571428571));
#138355=CARTESIAN_POINT('',(-17.5,1.00000037997959,-10.));
#138356=CARTESIAN_POINT('',(8.13264802145921,-14.4954839996407,-11.6428571428571));
#138357=CARTESIAN_POINT('Origin',(-8.88178376686733E-15,1.00000037997959,
-11.6428571428571));
#138358=CARTESIAN_POINT('Origin',(-8.88178376686733E-15,1.00000037997959,
-11.6428571428571));
#138359=CARTESIAN_POINT('Origin',(-8.88178376686733E-15,1.00000037997959,
-11.5678571428571));
#138360=CARTESIAN_POINT('',(-17.5,1.00000037997959,-11.5428571428571));
#138361=CARTESIAN_POINT('',(8.13264802145921,-14.4954839996407,-11.5428571428571));
#138362=CARTESIAN_POINT('Origin',(-8.88178376686733E-15,1.00000037997959,
-11.5428571428571));
#138363=CARTESIAN_POINT('',(8.08617574705085,-14.4069383746142,-11.5928571428572));
#138364=CARTESIAN_POINT('',(8.10941188425504,-14.4512111871275,-11.5678571428571));
#138365=CARTESIAN_POINT('Origin',(4.44089252863457E-15,1.00000037997959,
-11.5928571428571));
#138366=CARTESIAN_POINT('Origin',(-8.88178376686733E-15,1.00000037997959,
-11.5428571428571));
#138367=CARTESIAN_POINT('Origin',(-8.88178376686733E-15,1.00000037997959,
-11.6178571428571));
#138368=CARTESIAN_POINT('',(8.10941188425504,-14.4512111871275,-11.6178571428571));
#138369=CARTESIAN_POINT('Origin',(-8.88178376686733E-15,1.00000037997959,
-10.));
#138370=CARTESIAN_POINT('',(-17.5,1.00000037997959,-11.0714285714286));
#138371=CARTESIAN_POINT('',(-17.5,1.00000037997959,-10.));
#138372=CARTESIAN_POINT('',(8.13264802145921,-14.4954839996407,-11.0714285714286));
#138373=CARTESIAN_POINT('Origin',(-8.88178376686733E-15,1.00000037997959,
-11.0714285714286));
#138374=CARTESIAN_POINT('Origin',(-8.88178376686733E-15,1.00000037997959,
-11.0714285714286));
#138375=CARTESIAN_POINT('Origin',(-8.88178376686733E-15,1.00000037997959,
-10.9964285714286));
#138376=CARTESIAN_POINT('',(-17.5,1.00000037997959,-10.9714285714286));
#138377=CARTESIAN_POINT('',(8.13264802145921,-14.4954839996407,-10.9714285714286));
#138378=CARTESIAN_POINT('Origin',(-8.88178376686733E-15,1.00000037997959,
-10.9714285714286));
#138379=CARTESIAN_POINT('',(8.08617574705085,-14.4069383746142,-11.0214285714286));
#138380=CARTESIAN_POINT('',(8.10941188425504,-14.4512111871275,-10.9964285714286));
#138381=CARTESIAN_POINT('Origin',(4.44089252863457E-15,1.00000037997959,
-11.0214285714286));
#138382=CARTESIAN_POINT('Origin',(-8.88178376686733E-15,1.00000037997959,
-10.9714285714286));
#138383=CARTESIAN_POINT('Origin',(-8.88178376686733E-15,1.00000037997959,
-11.0464285714286));
#138384=CARTESIAN_POINT('',(8.10941188425504,-14.4512111871275,-11.0464285714286));
#138385=CARTESIAN_POINT('Origin',(21.9499999789786,0.999999999999992,-6.00000000000001));
#138386=CARTESIAN_POINT('Origin',(-8.88178376686733E-15,1.00000037997959,
-10.));
#138387=CARTESIAN_POINT('',(-17.5,1.00000037997959,-10.5));
#138388=CARTESIAN_POINT('',(-17.5,1.00000037997959,-10.));
#138389=CARTESIAN_POINT('',(8.13264802145921,-14.4954839996407,-10.5));
#138390=CARTESIAN_POINT('Origin',(-8.88178376686733E-15,1.00000037997959,
-10.5));
#138391=CARTESIAN_POINT('Origin',(-8.88178376686733E-15,1.00000037997959,
-10.5));
#138392=CARTESIAN_POINT('Origin',(-8.88178376686733E-15,1.00000037997959,
-10.425));
#138393=CARTESIAN_POINT('',(-17.5,1.00000037997959,-10.4));
#138394=CARTESIAN_POINT('',(8.13264802145921,-14.4954839996407,-10.4));
#138395=CARTESIAN_POINT('Origin',(-8.88178376686733E-15,1.00000037997959,
-10.4));
#138396=CARTESIAN_POINT('Origin',(-8.88178376686733E-15,1.00000037997959,
-10.4));
#138397=CARTESIAN_POINT('',(8.08617574705085,-14.4069383746142,-10.45));
#138398=CARTESIAN_POINT('',(8.10941188425504,-14.4512111871275,-10.425));
#138399=CARTESIAN_POINT('Origin',(4.44089252863457E-15,1.00000037997959,
-10.45));
#138400=CARTESIAN_POINT('Origin',(-8.88178376686733E-15,1.00000037997959,
-10.475));
#138401=CARTESIAN_POINT('',(8.10941188425504,-14.4512111871275,-10.475));
#138402=CARTESIAN_POINT('Origin',(-8.88178376686733E-15,1.00000037997959,
-10.));
#138403=CARTESIAN_POINT('',(-17.5,1.00000037997959,-10.));
#138404=CARTESIAN_POINT('Origin',(-8.88178376686733E-15,1.00000037997959,
-5.55111512312578E-15));
#138405=CARTESIAN_POINT('',(-1.50000000000001,1.00000037997959,-5.55111512312578E-15));
#138406=CARTESIAN_POINT('Origin',(-17.2355011741645,-5.00000000000001,-6.00000000000001));
#138407=CARTESIAN_POINT('Origin',(-2.10213452200843E-8,0.999999999999992,
-23.));
#459193=UNCERTAINTY_MEASURE_WITH_UNIT(LENGTH_MEASURE(0.01),#459243,
'DISTANCE_ACCURACY_VALUE',
'Maximum model space distance between geometric entities at asserted c
onnectivities');
#459216=UNCERTAINTY_MEASURE_WITH_UNIT(LENGTH_MEASURE(0.01),#459243,
'DISTANCE_ACCURACY_VALUE',
'Maximum model space distance between geometric entities at asserted c
onnectivities');
#459219=(
GEOMETRIC_REPRESENTATION_CONTEXT(3)
GLOBAL_UNCERTAINTY_ASSIGNED_CONTEXT((#459193))
GLOBAL_UNIT_ASSIGNED_CONTEXT((#459243,#459245,#459246))
REPRESENTATION_CONTEXT('','3D')
);
#459242=(
GEOMETRIC_REPRESENTATION_CONTEXT(3)
GLOBAL_UNCERTAINTY_ASSIGNED_CONTEXT((#459216))
GLOBAL_UNIT_ASSIGNED_CONTEXT((#459243,#459245,#459246))
REPRESENTATION_CONTEXT('','3D')
);
#459243=(
LENGTH_UNIT()
NAMED_UNIT(*)
SI_UNIT(.MILLI.,.METRE.)
);
#459245=(
NAMED_UNIT(*)
PLANE_ANGLE_UNIT()
SI_UNIT($,.RADIAN.)
);
#459246=(
NAMED_UNIT(*)
SI_UNIT($,.STERADIAN.)
SOLID_ANGLE_UNIT()
);
#459249=SHAPE_DEFINITION_REPRESENTATION(#459274,#459330);
#459274=PRODUCT_DEFINITION_SHAPE('',$,#459356);
#459330=SHAPE_REPRESENTATION('',(#94906),#459219);
#459353=PRODUCT_DEFINITION_CONTEXT('part definition',#459430,'design');
#459356=PRODUCT_DEFINITION('Stepper Motor','Stepper Motor',#459381,#459353);
#459381=PRODUCT_DEFINITION_FORMATION('',$,#459434);
#459430=APPLICATION_CONTEXT(
'Core Data for Automotive Mechanical Design Process');
#459431=PRODUCT_CONTEXT('part definition',#459430,'mechanical');
#459434=PRODUCT('Stepper Motor','Stepper Motor',$,(#459431));
#459534=COLOUR_RGB('Off White',0.89,0.88,0.83);
#459535=FILL_AREA_STYLE_COLOUR('',#459534);
#459536=FILL_AREA_STYLE('',(#459535));
#459537=SURFACE_STYLE_FILL_AREA(#459536);
#459538=SURFACE_SIDE_STYLE('',(#459537));
#459539=SURFACE_STYLE_USAGE(.BOTH.,#459538);
#459540=PRESENTATION_STYLE_ASSIGNMENT((#459539));
ENDSEC;
END-ISO-10303-21;
